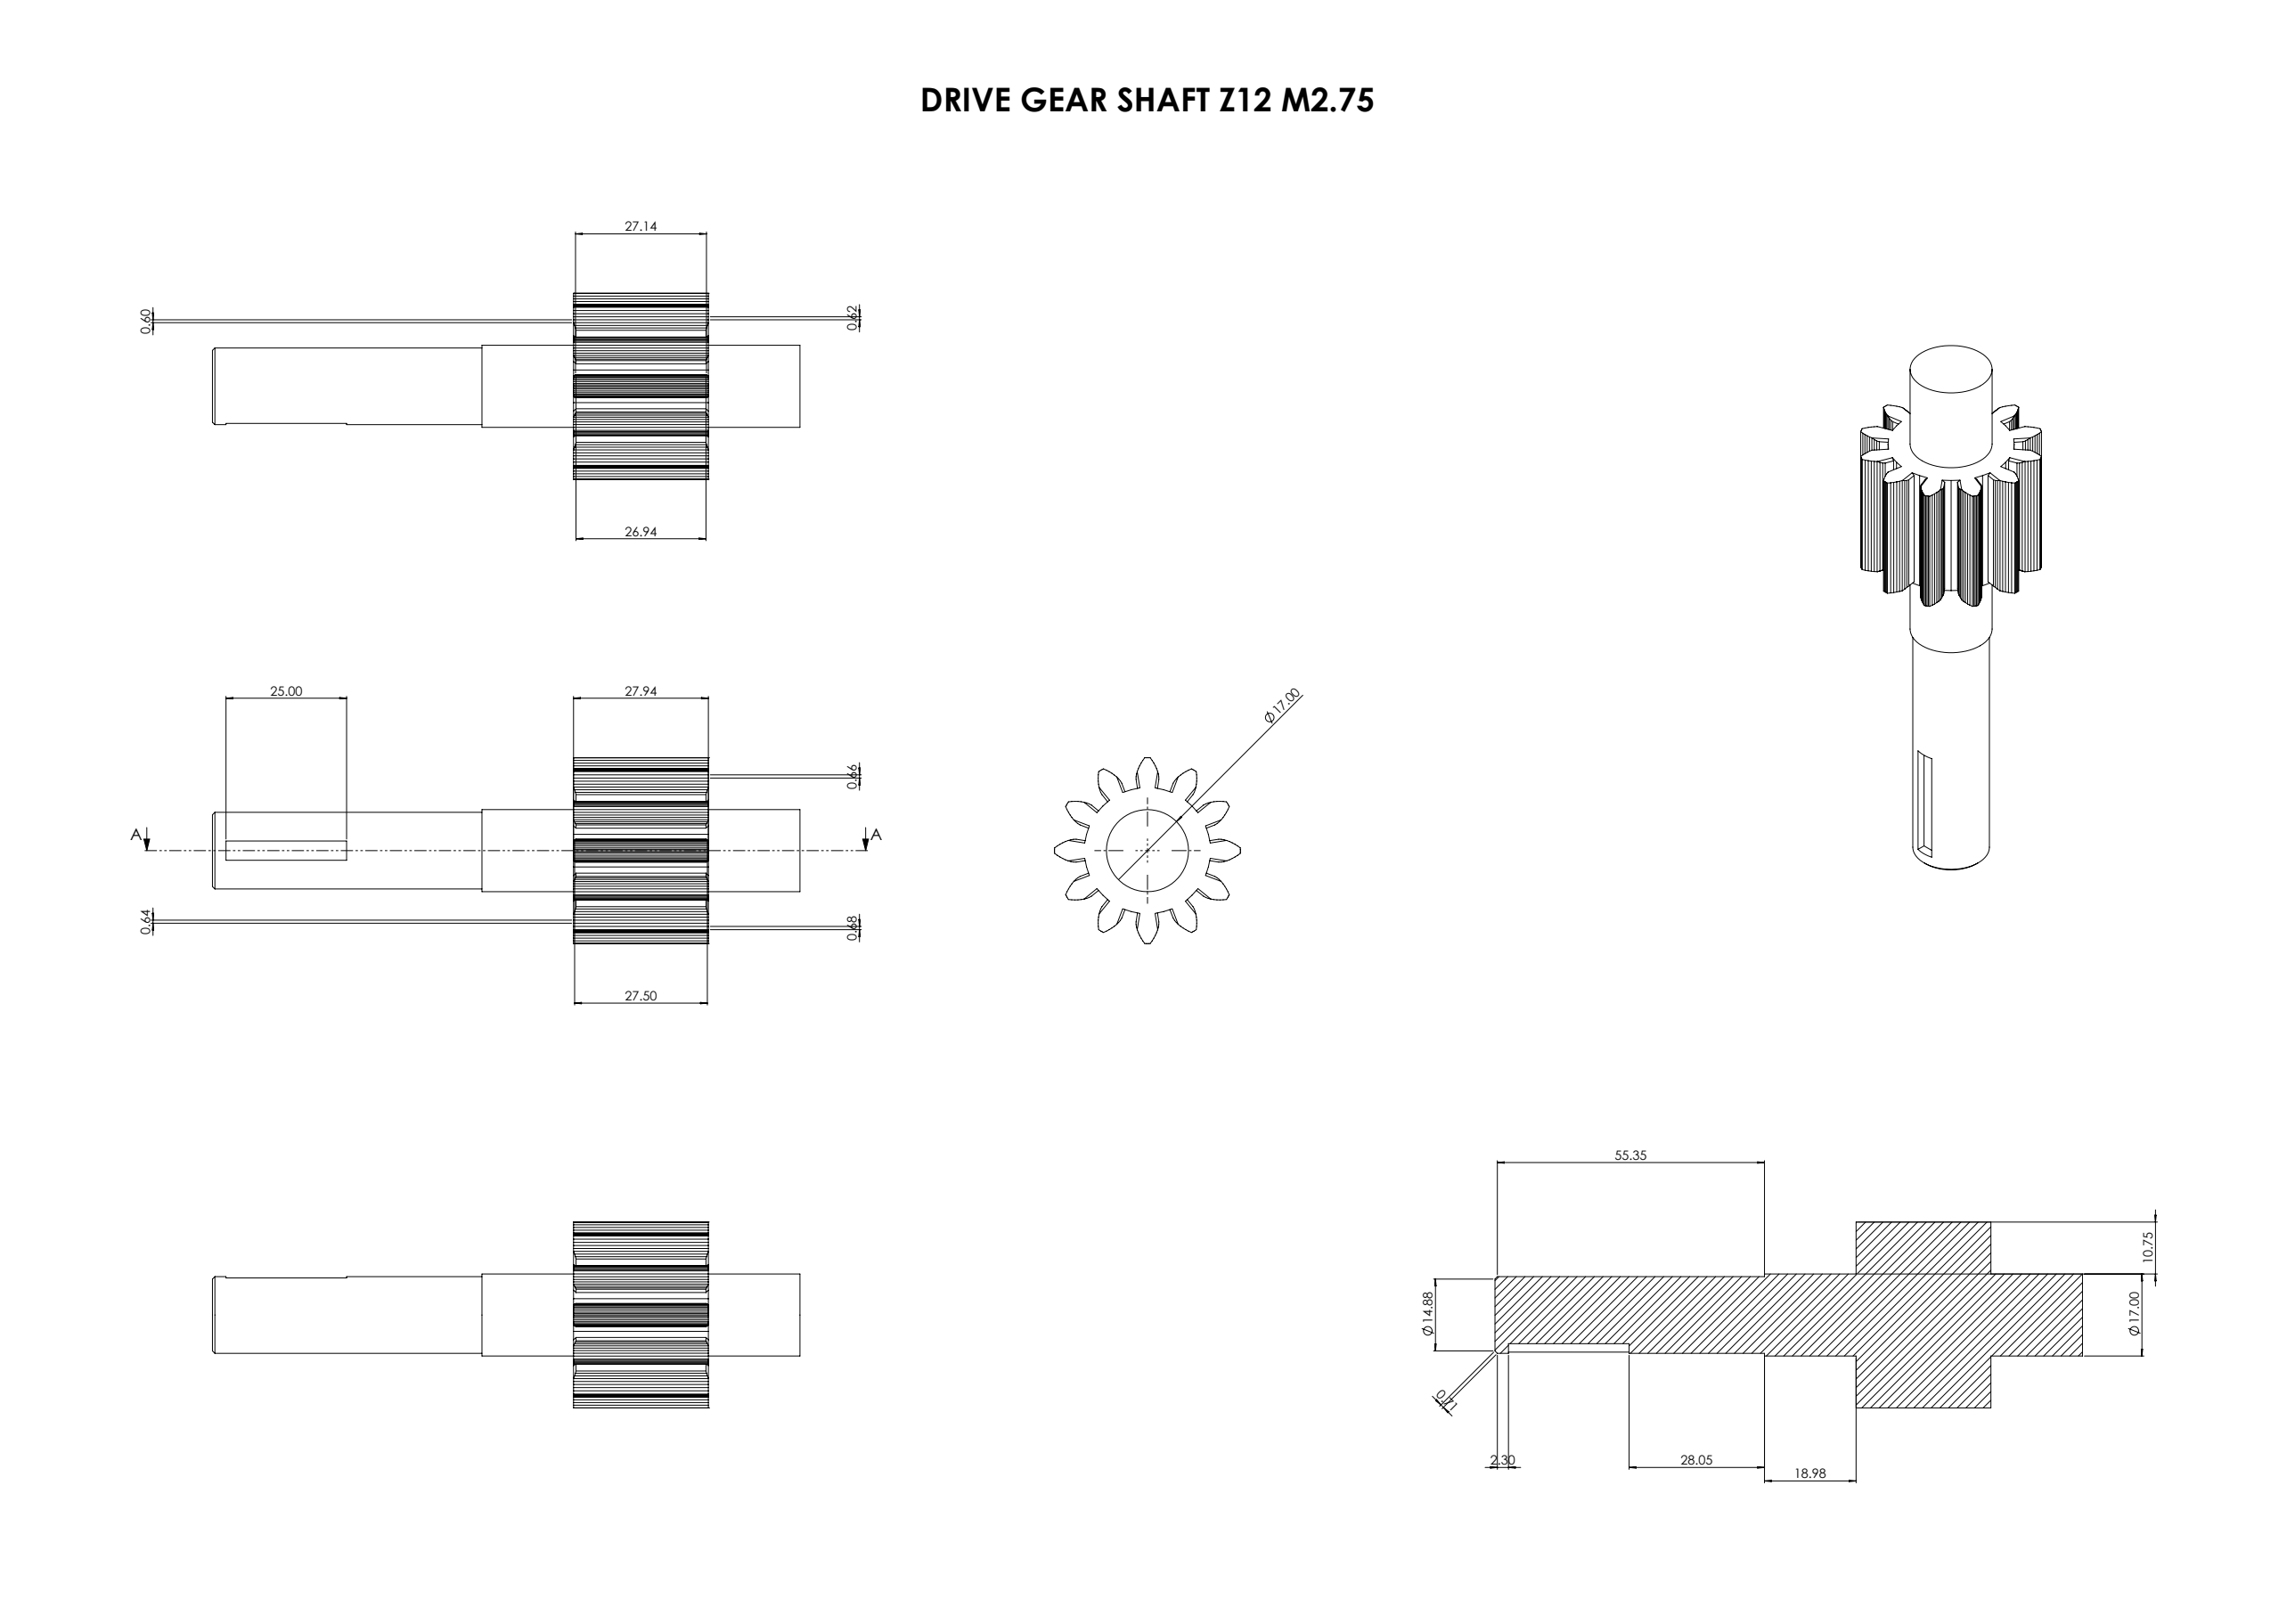
ISO-10303-21;
HEADER;
/* Generated by software containing ST-Developer
 * from STEP Tools, Inc. (www.steptools.com) 
 */

FILE_DESCRIPTION(
/* description */ (''),
/* implementation_level */ '2;1');

FILE_NAME(
/* name */ '04_Drive_Gear_Shaft_z12_m2.75.step',
/* time_stamp */ '2026-10-26T06:59:52-07:00',
/* author */ (''),
/* organization */ (''),
/* preprocessor_version */ 'ST-DEVELOPER v20.2',
/* originating_system */ 'Autodesk Translation Framework v15.15.0.0',
/* authorisation */ '');

FILE_SCHEMA (('AUTOMOTIVE_DESIGN { 1 0 10303 214 3 1 1 }'));
ENDSEC;

DATA;
#10=MECHANICAL_DESIGN_GEOMETRIC_PRESENTATION_REPRESENTATION('',(#167),#46395);
#139=SHAPE_REPRESENTATION_RELATIONSHIP('SRR','None',#46459,#153);
#153=ADVANCED_BREP_SHAPE_REPRESENTATION('',(#181),#46384);
#167=STYLED_ITEM('',(#46596),#181);
#181=MANIFOLD_SOLID_BREP('Body1',#24940);
#514=CYLINDRICAL_SURFACE('',#26051,8.5);
#515=CYLINDRICAL_SURFACE('',#26057,7.94);
#516=CYLINDRICAL_SURFACE('',#26060,8.5);
#645=FACE_BOUND('',#3444,.T.);
#646=FACE_BOUND('',#3518,.T.);
#647=FACE_BOUND('',#3791,.T.);
#648=FACE_BOUND('',#3793,.T.);
#814=PLANE('',#25704);
#815=PLANE('',#25705);
#816=PLANE('',#25707);
#817=PLANE('',#25708);
#818=PLANE('',#25709);
#819=PLANE('',#25710);
#820=PLANE('',#25711);
#821=PLANE('',#25712);
#822=PLANE('',#25713);
#823=PLANE('',#25714);
#824=PLANE('',#25715);
#825=PLANE('',#25716);
#826=PLANE('',#25717);
#827=PLANE('',#25718);
#828=PLANE('',#25719);
#829=PLANE('',#25720);
#830=PLANE('',#25721);
#831=PLANE('',#25722);
#832=PLANE('',#25723);
#833=PLANE('',#25724);
#834=PLANE('',#25725);
#835=PLANE('',#25726);
#836=PLANE('',#25727);
#837=PLANE('',#25728);
#838=PLANE('',#25729);
#839=PLANE('',#25730);
#840=PLANE('',#25731);
#841=PLANE('',#25732);
#842=PLANE('',#25733);
#843=PLANE('',#25734);
#844=PLANE('',#25735);
#845=PLANE('',#25736);
#846=PLANE('',#25737);
#847=PLANE('',#25738);
#848=PLANE('',#25739);
#849=PLANE('',#25740);
#850=PLANE('',#25741);
#851=PLANE('',#25742);
#852=PLANE('',#25743);
#853=PLANE('',#25744);
#854=PLANE('',#25745);
#855=PLANE('',#25746);
#856=PLANE('',#25747);
#857=PLANE('',#25748);
#858=PLANE('',#25749);
#859=PLANE('',#25750);
#860=PLANE('',#25751);
#861=PLANE('',#25752);
#862=PLANE('',#25753);
#863=PLANE('',#25754);
#864=PLANE('',#25755);
#865=PLANE('',#25756);
#866=PLANE('',#25757);
#867=PLANE('',#25758);
#868=PLANE('',#25759);
#869=PLANE('',#25760);
#870=PLANE('',#25761);
#871=PLANE('',#25762);
#872=PLANE('',#25763);
#873=PLANE('',#25764);
#874=PLANE('',#25765);
#875=PLANE('',#25766);
#876=PLANE('',#25767);
#877=PLANE('',#25768);
#878=PLANE('',#25769);
#879=PLANE('',#25770);
#880=PLANE('',#25771);
#881=PLANE('',#25772);
#882=PLANE('',#25773);
#883=PLANE('',#25774);
#884=PLANE('',#25775);
#885=PLANE('',#25776);
#886=PLANE('',#25777);
#887=PLANE('',#25778);
#888=PLANE('',#25779);
#889=PLANE('',#25781);
#890=PLANE('',#25782);
#891=PLANE('',#25783);
#892=PLANE('',#25784);
#893=PLANE('',#25785);
#894=PLANE('',#25786);
#895=PLANE('',#25787);
#896=PLANE('',#25788);
#897=PLANE('',#25789);
#898=PLANE('',#25790);
#899=PLANE('',#25791);
#900=PLANE('',#25792);
#901=PLANE('',#25793);
#902=PLANE('',#25794);
#903=PLANE('',#25795);
#904=PLANE('',#25796);
#905=PLANE('',#25797);
#906=PLANE('',#25798);
#907=PLANE('',#25799);
#908=PLANE('',#25800);
#909=PLANE('',#25801);
#910=PLANE('',#25802);
#911=PLANE('',#25803);
#912=PLANE('',#25804);
#913=PLANE('',#25806);
#914=PLANE('',#25807);
#915=PLANE('',#25808);
#916=PLANE('',#25810);
#917=PLANE('',#25811);
#918=PLANE('',#25812);
#919=PLANE('',#25813);
#920=PLANE('',#25814);
#921=PLANE('',#25815);
#922=PLANE('',#25816);
#923=PLANE('',#25817);
#924=PLANE('',#25818);
#925=PLANE('',#25819);
#926=PLANE('',#25820);
#927=PLANE('',#25821);
#928=PLANE('',#25822);
#929=PLANE('',#25823);
#930=PLANE('',#25824);
#931=PLANE('',#25825);
#932=PLANE('',#25826);
#933=PLANE('',#25827);
#934=PLANE('',#25828);
#935=PLANE('',#25829);
#936=PLANE('',#25830);
#937=PLANE('',#25831);
#938=PLANE('',#25832);
#939=PLANE('',#25833);
#940=PLANE('',#25834);
#941=PLANE('',#25835);
#942=PLANE('',#25836);
#943=PLANE('',#25837);
#944=PLANE('',#25838);
#945=PLANE('',#25839);
#946=PLANE('',#25840);
#947=PLANE('',#25841);
#948=PLANE('',#25842);
#949=PLANE('',#25843);
#950=PLANE('',#25844);
#951=PLANE('',#25845);
#952=PLANE('',#25846);
#953=PLANE('',#25847);
#954=PLANE('',#25848);
#955=PLANE('',#25849);
#956=PLANE('',#25850);
#957=PLANE('',#25851);
#958=PLANE('',#25852);
#959=PLANE('',#25853);
#960=PLANE('',#25854);
#961=PLANE('',#25855);
#962=PLANE('',#25856);
#963=PLANE('',#25857);
#964=PLANE('',#25858);
#965=PLANE('',#25859);
#966=PLANE('',#25860);
#967=PLANE('',#25861);
#968=PLANE('',#25862);
#969=PLANE('',#25863);
#970=PLANE('',#25864);
#971=PLANE('',#25865);
#972=PLANE('',#25866);
#973=PLANE('',#25867);
#974=PLANE('',#25868);
#975=PLANE('',#25869);
#976=PLANE('',#25870);
#977=PLANE('',#25871);
#978=PLANE('',#25872);
#979=PLANE('',#25873);
#980=PLANE('',#25874);
#981=PLANE('',#25875);
#982=PLANE('',#25876);
#983=PLANE('',#25877);
#984=PLANE('',#25878);
#985=PLANE('',#25879);
#986=PLANE('',#25880);
#987=PLANE('',#25881);
#988=PLANE('',#25882);
#989=PLANE('',#25883);
#990=PLANE('',#25884);
#991=PLANE('',#25885);
#992=PLANE('',#25886);
#993=PLANE('',#25887);
#994=PLANE('',#25888);
#995=PLANE('',#25889);
#996=PLANE('',#25890);
#997=PLANE('',#25891);
#998=PLANE('',#25892);
#999=PLANE('',#25893);
#1000=PLANE('',#25894);
#1001=PLANE('',#25895);
#1002=PLANE('',#25896);
#1003=PLANE('',#25897);
#1004=PLANE('',#25898);
#1005=PLANE('',#25899);
#1006=PLANE('',#25900);
#1007=PLANE('',#25901);
#1008=PLANE('',#25902);
#1009=PLANE('',#25903);
#1010=PLANE('',#25904);
#1011=PLANE('',#25905);
#1012=PLANE('',#25906);
#1013=PLANE('',#25907);
#1014=PLANE('',#25908);
#1015=PLANE('',#25909);
#1016=PLANE('',#25910);
#1017=PLANE('',#25911);
#1018=PLANE('',#25912);
#1019=PLANE('',#25913);
#1020=PLANE('',#25914);
#1021=PLANE('',#25915);
#1022=PLANE('',#25916);
#1023=PLANE('',#25917);
#1024=PLANE('',#25918);
#1025=PLANE('',#25919);
#1026=PLANE('',#25920);
#1027=PLANE('',#25921);
#1028=PLANE('',#25922);
#1029=PLANE('',#25923);
#1030=PLANE('',#25924);
#1031=PLANE('',#25925);
#1032=PLANE('',#25926);
#1033=PLANE('',#25927);
#1034=PLANE('',#25928);
#1035=PLANE('',#25929);
#1036=PLANE('',#25930);
#1037=PLANE('',#25931);
#1038=PLANE('',#25932);
#1039=PLANE('',#25933);
#1040=PLANE('',#25934);
#1041=PLANE('',#25935);
#1042=PLANE('',#25936);
#1043=PLANE('',#25937);
#1044=PLANE('',#25938);
#1045=PLANE('',#25939);
#1046=PLANE('',#25940);
#1047=PLANE('',#25941);
#1048=PLANE('',#25942);
#1049=PLANE('',#25943);
#1050=PLANE('',#25944);
#1051=PLANE('',#25945);
#1052=PLANE('',#25946);
#1053=PLANE('',#25947);
#1054=PLANE('',#25948);
#1055=PLANE('',#25949);
#1056=PLANE('',#25950);
#1057=PLANE('',#25951);
#1058=PLANE('',#25952);
#1059=PLANE('',#25953);
#1060=PLANE('',#25954);
#1061=PLANE('',#25955);
#1062=PLANE('',#25956);
#1063=PLANE('',#25957);
#1064=PLANE('',#25958);
#1065=PLANE('',#25959);
#1066=PLANE('',#25960);
#1067=PLANE('',#25961);
#1068=PLANE('',#25962);
#1069=PLANE('',#25963);
#1070=PLANE('',#25964);
#1071=PLANE('',#25965);
#1072=PLANE('',#25966);
#1073=PLANE('',#25967);
#1074=PLANE('',#25968);
#1075=PLANE('',#25969);
#1076=PLANE('',#25970);
#1077=PLANE('',#25971);
#1078=PLANE('',#25972);
#1079=PLANE('',#25973);
#1080=PLANE('',#25974);
#1081=PLANE('',#25975);
#1082=PLANE('',#25976);
#1083=PLANE('',#25977);
#1084=PLANE('',#25978);
#1085=PLANE('',#25979);
#1086=PLANE('',#25980);
#1087=PLANE('',#25981);
#1088=PLANE('',#25982);
#1089=PLANE('',#25983);
#1090=PLANE('',#25984);
#1091=PLANE('',#25985);
#1092=PLANE('',#25986);
#1093=PLANE('',#25987);
#1094=PLANE('',#25988);
#1095=PLANE('',#25989);
#1096=PLANE('',#25990);
#1097=PLANE('',#25991);
#1098=PLANE('',#25992);
#1099=PLANE('',#25993);
#1100=PLANE('',#25994);
#1101=PLANE('',#25995);
#1102=PLANE('',#25996);
#1103=PLANE('',#25997);
#1104=PLANE('',#25998);
#1105=PLANE('',#25999);
#1106=PLANE('',#26000);
#1107=PLANE('',#26001);
#1108=PLANE('',#26002);
#1109=PLANE('',#26003);
#1110=PLANE('',#26004);
#1111=PLANE('',#26005);
#1112=PLANE('',#26006);
#1113=PLANE('',#26007);
#1114=PLANE('',#26008);
#1115=PLANE('',#26009);
#1116=PLANE('',#26010);
#1117=PLANE('',#26011);
#1118=PLANE('',#26012);
#1119=PLANE('',#26013);
#1120=PLANE('',#26014);
#1121=PLANE('',#26015);
#1122=PLANE('',#26016);
#1123=PLANE('',#26017);
#1124=PLANE('',#26018);
#1125=PLANE('',#26019);
#1126=PLANE('',#26020);
#1127=PLANE('',#26021);
#1128=PLANE('',#26022);
#1129=PLANE('',#26023);
#1130=PLANE('',#26024);
#1131=PLANE('',#26025);
#1132=PLANE('',#26026);
#1133=PLANE('',#26027);
#1134=PLANE('',#26028);
#1135=PLANE('',#26029);
#1136=PLANE('',#26030);
#1137=PLANE('',#26031);
#1138=PLANE('',#26032);
#1139=PLANE('',#26033);
#1140=PLANE('',#26034);
#1141=PLANE('',#26035);
#1142=PLANE('',#26036);
#1143=PLANE('',#26037);
#1144=PLANE('',#26038);
#1145=PLANE('',#26039);
#1146=PLANE('',#26040);
#1147=PLANE('',#26041);
#1148=PLANE('',#26042);
#1149=PLANE('',#26043);
#1150=PLANE('',#26044);
#1151=PLANE('',#26045);
#1152=PLANE('',#26046);
#1153=PLANE('',#26047);
#1154=PLANE('',#26048);
#1155=PLANE('',#26049);
#1156=PLANE('',#26050);
#1157=PLANE('',#26053);
#1158=PLANE('',#26059);
#1159=PLANE('',#26062);
#2052=FACE_OUTER_BOUND('',#3442,.T.);
#2053=FACE_OUTER_BOUND('',#3443,.T.);
#2054=FACE_OUTER_BOUND('',#3445,.T.);
#2055=FACE_OUTER_BOUND('',#3446,.T.);
#2056=FACE_OUTER_BOUND('',#3447,.T.);
#2057=FACE_OUTER_BOUND('',#3448,.T.);
#2058=FACE_OUTER_BOUND('',#3449,.T.);
#2059=FACE_OUTER_BOUND('',#3450,.T.);
#2060=FACE_OUTER_BOUND('',#3451,.T.);
#2061=FACE_OUTER_BOUND('',#3452,.T.);
#2062=FACE_OUTER_BOUND('',#3453,.T.);
#2063=FACE_OUTER_BOUND('',#3454,.T.);
#2064=FACE_OUTER_BOUND('',#3455,.T.);
#2065=FACE_OUTER_BOUND('',#3456,.T.);
#2066=FACE_OUTER_BOUND('',#3457,.T.);
#2067=FACE_OUTER_BOUND('',#3458,.T.);
#2068=FACE_OUTER_BOUND('',#3459,.T.);
#2069=FACE_OUTER_BOUND('',#3460,.T.);
#2070=FACE_OUTER_BOUND('',#3461,.T.);
#2071=FACE_OUTER_BOUND('',#3462,.T.);
#2072=FACE_OUTER_BOUND('',#3463,.T.);
#2073=FACE_OUTER_BOUND('',#3464,.T.);
#2074=FACE_OUTER_BOUND('',#3465,.T.);
#2075=FACE_OUTER_BOUND('',#3466,.T.);
#2076=FACE_OUTER_BOUND('',#3467,.T.);
#2077=FACE_OUTER_BOUND('',#3468,.T.);
#2078=FACE_OUTER_BOUND('',#3469,.T.);
#2079=FACE_OUTER_BOUND('',#3470,.T.);
#2080=FACE_OUTER_BOUND('',#3471,.T.);
#2081=FACE_OUTER_BOUND('',#3472,.T.);
#2082=FACE_OUTER_BOUND('',#3473,.T.);
#2083=FACE_OUTER_BOUND('',#3474,.T.);
#2084=FACE_OUTER_BOUND('',#3475,.T.);
#2085=FACE_OUTER_BOUND('',#3476,.T.);
#2086=FACE_OUTER_BOUND('',#3477,.T.);
#2087=FACE_OUTER_BOUND('',#3478,.T.);
#2088=FACE_OUTER_BOUND('',#3479,.T.);
#2089=FACE_OUTER_BOUND('',#3480,.T.);
#2090=FACE_OUTER_BOUND('',#3481,.T.);
#2091=FACE_OUTER_BOUND('',#3482,.T.);
#2092=FACE_OUTER_BOUND('',#3483,.T.);
#2093=FACE_OUTER_BOUND('',#3484,.T.);
#2094=FACE_OUTER_BOUND('',#3485,.T.);
#2095=FACE_OUTER_BOUND('',#3486,.T.);
#2096=FACE_OUTER_BOUND('',#3487,.T.);
#2097=FACE_OUTER_BOUND('',#3488,.T.);
#2098=FACE_OUTER_BOUND('',#3489,.T.);
#2099=FACE_OUTER_BOUND('',#3490,.T.);
#2100=FACE_OUTER_BOUND('',#3491,.T.);
#2101=FACE_OUTER_BOUND('',#3492,.T.);
#2102=FACE_OUTER_BOUND('',#3493,.T.);
#2103=FACE_OUTER_BOUND('',#3494,.T.);
#2104=FACE_OUTER_BOUND('',#3495,.T.);
#2105=FACE_OUTER_BOUND('',#3496,.T.);
#2106=FACE_OUTER_BOUND('',#3497,.T.);
#2107=FACE_OUTER_BOUND('',#3498,.T.);
#2108=FACE_OUTER_BOUND('',#3499,.T.);
#2109=FACE_OUTER_BOUND('',#3500,.T.);
#2110=FACE_OUTER_BOUND('',#3501,.T.);
#2111=FACE_OUTER_BOUND('',#3502,.T.);
#2112=FACE_OUTER_BOUND('',#3503,.T.);
#2113=FACE_OUTER_BOUND('',#3504,.T.);
#2114=FACE_OUTER_BOUND('',#3505,.T.);
#2115=FACE_OUTER_BOUND('',#3506,.T.);
#2116=FACE_OUTER_BOUND('',#3507,.T.);
#2117=FACE_OUTER_BOUND('',#3508,.T.);
#2118=FACE_OUTER_BOUND('',#3509,.T.);
#2119=FACE_OUTER_BOUND('',#3510,.T.);
#2120=FACE_OUTER_BOUND('',#3511,.T.);
#2121=FACE_OUTER_BOUND('',#3512,.T.);
#2122=FACE_OUTER_BOUND('',#3513,.T.);
#2123=FACE_OUTER_BOUND('',#3514,.T.);
#2124=FACE_OUTER_BOUND('',#3515,.T.);
#2125=FACE_OUTER_BOUND('',#3516,.T.);
#2126=FACE_OUTER_BOUND('',#3517,.T.);
#2127=FACE_OUTER_BOUND('',#3519,.T.);
#2128=FACE_OUTER_BOUND('',#3520,.T.);
#2129=FACE_OUTER_BOUND('',#3521,.T.);
#2130=FACE_OUTER_BOUND('',#3522,.T.);
#2131=FACE_OUTER_BOUND('',#3523,.T.);
#2132=FACE_OUTER_BOUND('',#3524,.T.);
#2133=FACE_OUTER_BOUND('',#3525,.T.);
#2134=FACE_OUTER_BOUND('',#3526,.T.);
#2135=FACE_OUTER_BOUND('',#3527,.T.);
#2136=FACE_OUTER_BOUND('',#3528,.T.);
#2137=FACE_OUTER_BOUND('',#3529,.T.);
#2138=FACE_OUTER_BOUND('',#3530,.T.);
#2139=FACE_OUTER_BOUND('',#3531,.T.);
#2140=FACE_OUTER_BOUND('',#3532,.T.);
#2141=FACE_OUTER_BOUND('',#3533,.T.);
#2142=FACE_OUTER_BOUND('',#3534,.T.);
#2143=FACE_OUTER_BOUND('',#3535,.T.);
#2144=FACE_OUTER_BOUND('',#3536,.T.);
#2145=FACE_OUTER_BOUND('',#3537,.T.);
#2146=FACE_OUTER_BOUND('',#3538,.T.);
#2147=FACE_OUTER_BOUND('',#3539,.T.);
#2148=FACE_OUTER_BOUND('',#3540,.T.);
#2149=FACE_OUTER_BOUND('',#3541,.T.);
#2150=FACE_OUTER_BOUND('',#3542,.T.);
#2151=FACE_OUTER_BOUND('',#3543,.T.);
#2152=FACE_OUTER_BOUND('',#3544,.T.);
#2153=FACE_OUTER_BOUND('',#3545,.T.);
#2154=FACE_OUTER_BOUND('',#3546,.T.);
#2155=FACE_OUTER_BOUND('',#3547,.T.);
#2156=FACE_OUTER_BOUND('',#3548,.T.);
#2157=FACE_OUTER_BOUND('',#3549,.T.);
#2158=FACE_OUTER_BOUND('',#3550,.T.);
#2159=FACE_OUTER_BOUND('',#3551,.T.);
#2160=FACE_OUTER_BOUND('',#3552,.T.);
#2161=FACE_OUTER_BOUND('',#3553,.T.);
#2162=FACE_OUTER_BOUND('',#3554,.T.);
#2163=FACE_OUTER_BOUND('',#3555,.T.);
#2164=FACE_OUTER_BOUND('',#3556,.T.);
#2165=FACE_OUTER_BOUND('',#3557,.T.);
#2166=FACE_OUTER_BOUND('',#3558,.T.);
#2167=FACE_OUTER_BOUND('',#3559,.T.);
#2168=FACE_OUTER_BOUND('',#3560,.T.);
#2169=FACE_OUTER_BOUND('',#3561,.T.);
#2170=FACE_OUTER_BOUND('',#3562,.T.);
#2171=FACE_OUTER_BOUND('',#3563,.T.);
#2172=FACE_OUTER_BOUND('',#3564,.T.);
#2173=FACE_OUTER_BOUND('',#3565,.T.);
#2174=FACE_OUTER_BOUND('',#3566,.T.);
#2175=FACE_OUTER_BOUND('',#3567,.T.);
#2176=FACE_OUTER_BOUND('',#3568,.T.);
#2177=FACE_OUTER_BOUND('',#3569,.T.);
#2178=FACE_OUTER_BOUND('',#3570,.T.);
#2179=FACE_OUTER_BOUND('',#3571,.T.);
#2180=FACE_OUTER_BOUND('',#3572,.T.);
#2181=FACE_OUTER_BOUND('',#3573,.T.);
#2182=FACE_OUTER_BOUND('',#3574,.T.);
#2183=FACE_OUTER_BOUND('',#3575,.T.);
#2184=FACE_OUTER_BOUND('',#3576,.T.);
#2185=FACE_OUTER_BOUND('',#3577,.T.);
#2186=FACE_OUTER_BOUND('',#3578,.T.);
#2187=FACE_OUTER_BOUND('',#3579,.T.);
#2188=FACE_OUTER_BOUND('',#3580,.T.);
#2189=FACE_OUTER_BOUND('',#3581,.T.);
#2190=FACE_OUTER_BOUND('',#3582,.T.);
#2191=FACE_OUTER_BOUND('',#3583,.T.);
#2192=FACE_OUTER_BOUND('',#3584,.T.);
#2193=FACE_OUTER_BOUND('',#3585,.T.);
#2194=FACE_OUTER_BOUND('',#3586,.T.);
#2195=FACE_OUTER_BOUND('',#3587,.T.);
#2196=FACE_OUTER_BOUND('',#3588,.T.);
#2197=FACE_OUTER_BOUND('',#3589,.T.);
#2198=FACE_OUTER_BOUND('',#3590,.T.);
#2199=FACE_OUTER_BOUND('',#3591,.T.);
#2200=FACE_OUTER_BOUND('',#3592,.T.);
#2201=FACE_OUTER_BOUND('',#3593,.T.);
#2202=FACE_OUTER_BOUND('',#3594,.T.);
#2203=FACE_OUTER_BOUND('',#3595,.T.);
#2204=FACE_OUTER_BOUND('',#3596,.T.);
#2205=FACE_OUTER_BOUND('',#3597,.T.);
#2206=FACE_OUTER_BOUND('',#3598,.T.);
#2207=FACE_OUTER_BOUND('',#3599,.T.);
#2208=FACE_OUTER_BOUND('',#3600,.T.);
#2209=FACE_OUTER_BOUND('',#3601,.T.);
#2210=FACE_OUTER_BOUND('',#3602,.T.);
#2211=FACE_OUTER_BOUND('',#3603,.T.);
#2212=FACE_OUTER_BOUND('',#3604,.T.);
#2213=FACE_OUTER_BOUND('',#3605,.T.);
#2214=FACE_OUTER_BOUND('',#3606,.T.);
#2215=FACE_OUTER_BOUND('',#3607,.T.);
#2216=FACE_OUTER_BOUND('',#3608,.T.);
#2217=FACE_OUTER_BOUND('',#3609,.T.);
#2218=FACE_OUTER_BOUND('',#3610,.T.);
#2219=FACE_OUTER_BOUND('',#3611,.T.);
#2220=FACE_OUTER_BOUND('',#3612,.T.);
#2221=FACE_OUTER_BOUND('',#3613,.T.);
#2222=FACE_OUTER_BOUND('',#3614,.T.);
#2223=FACE_OUTER_BOUND('',#3615,.T.);
#2224=FACE_OUTER_BOUND('',#3616,.T.);
#2225=FACE_OUTER_BOUND('',#3617,.T.);
#2226=FACE_OUTER_BOUND('',#3618,.T.);
#2227=FACE_OUTER_BOUND('',#3619,.T.);
#2228=FACE_OUTER_BOUND('',#3620,.T.);
#2229=FACE_OUTER_BOUND('',#3621,.T.);
#2230=FACE_OUTER_BOUND('',#3622,.T.);
#2231=FACE_OUTER_BOUND('',#3623,.T.);
#2232=FACE_OUTER_BOUND('',#3624,.T.);
#2233=FACE_OUTER_BOUND('',#3625,.T.);
#2234=FACE_OUTER_BOUND('',#3626,.T.);
#2235=FACE_OUTER_BOUND('',#3627,.T.);
#2236=FACE_OUTER_BOUND('',#3628,.T.);
#2237=FACE_OUTER_BOUND('',#3629,.T.);
#2238=FACE_OUTER_BOUND('',#3630,.T.);
#2239=FACE_OUTER_BOUND('',#3631,.T.);
#2240=FACE_OUTER_BOUND('',#3632,.T.);
#2241=FACE_OUTER_BOUND('',#3633,.T.);
#2242=FACE_OUTER_BOUND('',#3634,.T.);
#2243=FACE_OUTER_BOUND('',#3635,.T.);
#2244=FACE_OUTER_BOUND('',#3636,.T.);
#2245=FACE_OUTER_BOUND('',#3637,.T.);
#2246=FACE_OUTER_BOUND('',#3638,.T.);
#2247=FACE_OUTER_BOUND('',#3639,.T.);
#2248=FACE_OUTER_BOUND('',#3640,.T.);
#2249=FACE_OUTER_BOUND('',#3641,.T.);
#2250=FACE_OUTER_BOUND('',#3642,.T.);
#2251=FACE_OUTER_BOUND('',#3643,.T.);
#2252=FACE_OUTER_BOUND('',#3644,.T.);
#2253=FACE_OUTER_BOUND('',#3645,.T.);
#2254=FACE_OUTER_BOUND('',#3646,.T.);
#2255=FACE_OUTER_BOUND('',#3647,.T.);
#2256=FACE_OUTER_BOUND('',#3648,.T.);
#2257=FACE_OUTER_BOUND('',#3649,.T.);
#2258=FACE_OUTER_BOUND('',#3650,.T.);
#2259=FACE_OUTER_BOUND('',#3651,.T.);
#2260=FACE_OUTER_BOUND('',#3652,.T.);
#2261=FACE_OUTER_BOUND('',#3653,.T.);
#2262=FACE_OUTER_BOUND('',#3654,.T.);
#2263=FACE_OUTER_BOUND('',#3655,.T.);
#2264=FACE_OUTER_BOUND('',#3656,.T.);
#2265=FACE_OUTER_BOUND('',#3657,.T.);
#2266=FACE_OUTER_BOUND('',#3658,.T.);
#2267=FACE_OUTER_BOUND('',#3659,.T.);
#2268=FACE_OUTER_BOUND('',#3660,.T.);
#2269=FACE_OUTER_BOUND('',#3661,.T.);
#2270=FACE_OUTER_BOUND('',#3662,.T.);
#2271=FACE_OUTER_BOUND('',#3663,.T.);
#2272=FACE_OUTER_BOUND('',#3664,.T.);
#2273=FACE_OUTER_BOUND('',#3665,.T.);
#2274=FACE_OUTER_BOUND('',#3666,.T.);
#2275=FACE_OUTER_BOUND('',#3667,.T.);
#2276=FACE_OUTER_BOUND('',#3668,.T.);
#2277=FACE_OUTER_BOUND('',#3669,.T.);
#2278=FACE_OUTER_BOUND('',#3670,.T.);
#2279=FACE_OUTER_BOUND('',#3671,.T.);
#2280=FACE_OUTER_BOUND('',#3672,.T.);
#2281=FACE_OUTER_BOUND('',#3673,.T.);
#2282=FACE_OUTER_BOUND('',#3674,.T.);
#2283=FACE_OUTER_BOUND('',#3675,.T.);
#2284=FACE_OUTER_BOUND('',#3676,.T.);
#2285=FACE_OUTER_BOUND('',#3677,.T.);
#2286=FACE_OUTER_BOUND('',#3678,.T.);
#2287=FACE_OUTER_BOUND('',#3679,.T.);
#2288=FACE_OUTER_BOUND('',#3680,.T.);
#2289=FACE_OUTER_BOUND('',#3681,.T.);
#2290=FACE_OUTER_BOUND('',#3682,.T.);
#2291=FACE_OUTER_BOUND('',#3683,.T.);
#2292=FACE_OUTER_BOUND('',#3684,.T.);
#2293=FACE_OUTER_BOUND('',#3685,.T.);
#2294=FACE_OUTER_BOUND('',#3686,.T.);
#2295=FACE_OUTER_BOUND('',#3687,.T.);
#2296=FACE_OUTER_BOUND('',#3688,.T.);
#2297=FACE_OUTER_BOUND('',#3689,.T.);
#2298=FACE_OUTER_BOUND('',#3690,.T.);
#2299=FACE_OUTER_BOUND('',#3691,.T.);
#2300=FACE_OUTER_BOUND('',#3692,.T.);
#2301=FACE_OUTER_BOUND('',#3693,.T.);
#2302=FACE_OUTER_BOUND('',#3694,.T.);
#2303=FACE_OUTER_BOUND('',#3695,.T.);
#2304=FACE_OUTER_BOUND('',#3696,.T.);
#2305=FACE_OUTER_BOUND('',#3697,.T.);
#2306=FACE_OUTER_BOUND('',#3698,.T.);
#2307=FACE_OUTER_BOUND('',#3699,.T.);
#2308=FACE_OUTER_BOUND('',#3700,.T.);
#2309=FACE_OUTER_BOUND('',#3701,.T.);
#2310=FACE_OUTER_BOUND('',#3702,.T.);
#2311=FACE_OUTER_BOUND('',#3703,.T.);
#2312=FACE_OUTER_BOUND('',#3704,.T.);
#2313=FACE_OUTER_BOUND('',#3705,.T.);
#2314=FACE_OUTER_BOUND('',#3706,.T.);
#2315=FACE_OUTER_BOUND('',#3707,.T.);
#2316=FACE_OUTER_BOUND('',#3708,.T.);
#2317=FACE_OUTER_BOUND('',#3709,.T.);
#2318=FACE_OUTER_BOUND('',#3710,.T.);
#2319=FACE_OUTER_BOUND('',#3711,.T.);
#2320=FACE_OUTER_BOUND('',#3712,.T.);
#2321=FACE_OUTER_BOUND('',#3713,.T.);
#2322=FACE_OUTER_BOUND('',#3714,.T.);
#2323=FACE_OUTER_BOUND('',#3715,.T.);
#2324=FACE_OUTER_BOUND('',#3716,.T.);
#2325=FACE_OUTER_BOUND('',#3717,.T.);
#2326=FACE_OUTER_BOUND('',#3718,.T.);
#2327=FACE_OUTER_BOUND('',#3719,.T.);
#2328=FACE_OUTER_BOUND('',#3720,.T.);
#2329=FACE_OUTER_BOUND('',#3721,.T.);
#2330=FACE_OUTER_BOUND('',#3722,.T.);
#2331=FACE_OUTER_BOUND('',#3723,.T.);
#2332=FACE_OUTER_BOUND('',#3724,.T.);
#2333=FACE_OUTER_BOUND('',#3725,.T.);
#2334=FACE_OUTER_BOUND('',#3726,.T.);
#2335=FACE_OUTER_BOUND('',#3727,.T.);
#2336=FACE_OUTER_BOUND('',#3728,.T.);
#2337=FACE_OUTER_BOUND('',#3729,.T.);
#2338=FACE_OUTER_BOUND('',#3730,.T.);
#2339=FACE_OUTER_BOUND('',#3731,.T.);
#2340=FACE_OUTER_BOUND('',#3732,.T.);
#2341=FACE_OUTER_BOUND('',#3733,.T.);
#2342=FACE_OUTER_BOUND('',#3734,.T.);
#2343=FACE_OUTER_BOUND('',#3735,.T.);
#2344=FACE_OUTER_BOUND('',#3736,.T.);
#2345=FACE_OUTER_BOUND('',#3737,.T.);
#2346=FACE_OUTER_BOUND('',#3738,.T.);
#2347=FACE_OUTER_BOUND('',#3739,.T.);
#2348=FACE_OUTER_BOUND('',#3740,.T.);
#2349=FACE_OUTER_BOUND('',#3741,.T.);
#2350=FACE_OUTER_BOUND('',#3742,.T.);
#2351=FACE_OUTER_BOUND('',#3743,.T.);
#2352=FACE_OUTER_BOUND('',#3744,.T.);
#2353=FACE_OUTER_BOUND('',#3745,.T.);
#2354=FACE_OUTER_BOUND('',#3746,.T.);
#2355=FACE_OUTER_BOUND('',#3747,.T.);
#2356=FACE_OUTER_BOUND('',#3748,.T.);
#2357=FACE_OUTER_BOUND('',#3749,.T.);
#2358=FACE_OUTER_BOUND('',#3750,.T.);
#2359=FACE_OUTER_BOUND('',#3751,.T.);
#2360=FACE_OUTER_BOUND('',#3752,.T.);
#2361=FACE_OUTER_BOUND('',#3753,.T.);
#2362=FACE_OUTER_BOUND('',#3754,.T.);
#2363=FACE_OUTER_BOUND('',#3755,.T.);
#2364=FACE_OUTER_BOUND('',#3756,.T.);
#2365=FACE_OUTER_BOUND('',#3757,.T.);
#2366=FACE_OUTER_BOUND('',#3758,.T.);
#2367=FACE_OUTER_BOUND('',#3759,.T.);
#2368=FACE_OUTER_BOUND('',#3760,.T.);
#2369=FACE_OUTER_BOUND('',#3761,.T.);
#2370=FACE_OUTER_BOUND('',#3762,.T.);
#2371=FACE_OUTER_BOUND('',#3763,.T.);
#2372=FACE_OUTER_BOUND('',#3764,.T.);
#2373=FACE_OUTER_BOUND('',#3765,.T.);
#2374=FACE_OUTER_BOUND('',#3766,.T.);
#2375=FACE_OUTER_BOUND('',#3767,.T.);
#2376=FACE_OUTER_BOUND('',#3768,.T.);
#2377=FACE_OUTER_BOUND('',#3769,.T.);
#2378=FACE_OUTER_BOUND('',#3770,.T.);
#2379=FACE_OUTER_BOUND('',#3771,.T.);
#2380=FACE_OUTER_BOUND('',#3772,.T.);
#2381=FACE_OUTER_BOUND('',#3773,.T.);
#2382=FACE_OUTER_BOUND('',#3774,.T.);
#2383=FACE_OUTER_BOUND('',#3775,.T.);
#2384=FACE_OUTER_BOUND('',#3776,.T.);
#2385=FACE_OUTER_BOUND('',#3777,.T.);
#2386=FACE_OUTER_BOUND('',#3778,.T.);
#2387=FACE_OUTER_BOUND('',#3779,.T.);
#2388=FACE_OUTER_BOUND('',#3780,.T.);
#2389=FACE_OUTER_BOUND('',#3781,.T.);
#2390=FACE_OUTER_BOUND('',#3782,.T.);
#2391=FACE_OUTER_BOUND('',#3783,.T.);
#2392=FACE_OUTER_BOUND('',#3784,.T.);
#2393=FACE_OUTER_BOUND('',#3785,.T.);
#2394=FACE_OUTER_BOUND('',#3786,.T.);
#2395=FACE_OUTER_BOUND('',#3787,.T.);
#2396=FACE_OUTER_BOUND('',#3788,.T.);
#2397=FACE_OUTER_BOUND('',#3789,.T.);
#2398=FACE_OUTER_BOUND('',#3790,.T.);
#2399=FACE_OUTER_BOUND('',#3792,.T.);
#2400=FACE_OUTER_BOUND('',#3794,.T.);
#2401=FACE_OUTER_BOUND('',#3795,.T.);
#3442=EDGE_LOOP('',(#17926,#17927,#17928,#17929,#17930,#17931));
#3443=EDGE_LOOP('',(#17932,#17933,#17934,#17935,#17936,#17937,#17938,#17939,
#17940,#17941,#17942,#17943,#17944,#17945,#17946,#17947,#17948,#17949,#17950,
#17951,#17952,#17953,#17954,#17955,#17956,#17957,#17958,#17959,#17960,#17961,
#17962,#17963,#17964,#17965,#17966,#17967,#17968,#17969,#17970,#17971,#17972,
#17973,#17974,#17975,#17976,#17977,#17978,#17979,#17980,#17981,#17982,#17983,
#17984,#17985,#17986,#17987,#17988,#17989,#17990,#17991,#17992,#17993,#17994,
#17995,#17996,#17997,#17998,#17999,#18000,#18001,#18002,#18003,#18004,#18005,
#18006,#18007,#18008,#18009,#18010,#18011,#18012,#18013,#18014,#18015,#18016,
#18017,#18018,#18019,#18020,#18021,#18022,#18023,#18024,#18025,#18026,#18027,
#18028,#18029,#18030,#18031,#18032,#18033,#18034,#18035,#18036,#18037,#18038,
#18039,#18040,#18041,#18042,#18043,#18044,#18045,#18046,#18047,#18048,#18049,
#18050,#18051,#18052,#18053,#18054,#18055,#18056,#18057,#18058,#18059,#18060,
#18061,#18062,#18063,#18064,#18065,#18066,#18067,#18068,#18069,#18070,#18071,
#18072,#18073,#18074,#18075,#18076,#18077,#18078,#18079,#18080,#18081,#18082,
#18083,#18084,#18085,#18086,#18087,#18088,#18089,#18090,#18091,#18092,#18093,
#18094,#18095,#18096,#18097,#18098,#18099,#18100,#18101,#18102,#18103,#18104,
#18105,#18106,#18107,#18108,#18109,#18110,#18111,#18112,#18113,#18114,#18115,
#18116,#18117,#18118,#18119,#18120,#18121,#18122,#18123,#18124,#18125,#18126,
#18127,#18128,#18129,#18130,#18131,#18132,#18133,#18134,#18135,#18136,#18137,
#18138,#18139,#18140,#18141,#18142,#18143,#18144,#18145,#18146,#18147,#18148,
#18149,#18150,#18151,#18152,#18153,#18154,#18155,#18156,#18157,#18158,#18159,
#18160,#18161,#18162,#18163,#18164,#18165,#18166,#18167,#18168,#18169,#18170,
#18171));
#3444=EDGE_LOOP('',(#18172));
#3445=EDGE_LOOP('',(#18173,#18174,#18175,#18176,#18177,#18178));
#3446=EDGE_LOOP('',(#18179,#18180,#18181,#18182));
#3447=EDGE_LOOP('',(#18183,#18184,#18185,#18186,#18187,#18188));
#3448=EDGE_LOOP('',(#18189,#18190,#18191,#18192,#18193,#18194));
#3449=EDGE_LOOP('',(#18195,#18196,#18197,#18198));
#3450=EDGE_LOOP('',(#18199,#18200,#18201,#18202,#18203,#18204));
#3451=EDGE_LOOP('',(#18205,#18206,#18207,#18208,#18209,#18210));
#3452=EDGE_LOOP('',(#18211,#18212,#18213,#18214));
#3453=EDGE_LOOP('',(#18215,#18216,#18217,#18218,#18219,#18220));
#3454=EDGE_LOOP('',(#18221,#18222,#18223,#18224,#18225,#18226));
#3455=EDGE_LOOP('',(#18227,#18228,#18229,#18230));
#3456=EDGE_LOOP('',(#18231,#18232,#18233,#18234,#18235,#18236));
#3457=EDGE_LOOP('',(#18237,#18238,#18239,#18240,#18241,#18242));
#3458=EDGE_LOOP('',(#18243,#18244,#18245,#18246));
#3459=EDGE_LOOP('',(#18247,#18248,#18249,#18250,#18251,#18252));
#3460=EDGE_LOOP('',(#18253,#18254,#18255,#18256,#18257,#18258));
#3461=EDGE_LOOP('',(#18259,#18260,#18261,#18262));
#3462=EDGE_LOOP('',(#18263,#18264,#18265,#18266,#18267,#18268));
#3463=EDGE_LOOP('',(#18269,#18270,#18271,#18272,#18273,#18274));
#3464=EDGE_LOOP('',(#18275,#18276,#18277,#18278));
#3465=EDGE_LOOP('',(#18279,#18280,#18281,#18282,#18283,#18284));
#3466=EDGE_LOOP('',(#18285,#18286,#18287,#18288,#18289,#18290));
#3467=EDGE_LOOP('',(#18291,#18292,#18293,#18294));
#3468=EDGE_LOOP('',(#18295,#18296,#18297,#18298,#18299,#18300));
#3469=EDGE_LOOP('',(#18301,#18302,#18303,#18304,#18305,#18306));
#3470=EDGE_LOOP('',(#18307,#18308,#18309,#18310));
#3471=EDGE_LOOP('',(#18311,#18312,#18313,#18314,#18315,#18316));
#3472=EDGE_LOOP('',(#18317,#18318,#18319,#18320,#18321,#18322));
#3473=EDGE_LOOP('',(#18323,#18324,#18325,#18326));
#3474=EDGE_LOOP('',(#18327,#18328,#18329,#18330,#18331,#18332));
#3475=EDGE_LOOP('',(#18333,#18334,#18335,#18336,#18337,#18338));
#3476=EDGE_LOOP('',(#18339,#18340,#18341,#18342));
#3477=EDGE_LOOP('',(#18343,#18344,#18345,#18346,#18347,#18348));
#3478=EDGE_LOOP('',(#18349,#18350,#18351,#18352,#18353,#18354));
#3479=EDGE_LOOP('',(#18355,#18356,#18357,#18358));
#3480=EDGE_LOOP('',(#18359,#18360,#18361,#18362,#18363,#18364));
#3481=EDGE_LOOP('',(#18365,#18366,#18367,#18368));
#3482=EDGE_LOOP('',(#18369,#18370,#18371,#18372));
#3483=EDGE_LOOP('',(#18373,#18374,#18375,#18376,#18377,#18378));
#3484=EDGE_LOOP('',(#18379,#18380,#18381,#18382));
#3485=EDGE_LOOP('',(#18383,#18384,#18385,#18386));
#3486=EDGE_LOOP('',(#18387,#18388,#18389,#18390,#18391,#18392));
#3487=EDGE_LOOP('',(#18393,#18394,#18395,#18396));
#3488=EDGE_LOOP('',(#18397,#18398,#18399,#18400));
#3489=EDGE_LOOP('',(#18401,#18402,#18403,#18404,#18405,#18406));
#3490=EDGE_LOOP('',(#18407,#18408,#18409,#18410));
#3491=EDGE_LOOP('',(#18411,#18412,#18413,#18414));
#3492=EDGE_LOOP('',(#18415,#18416,#18417,#18418,#18419,#18420));
#3493=EDGE_LOOP('',(#18421,#18422,#18423,#18424));
#3494=EDGE_LOOP('',(#18425,#18426,#18427,#18428));
#3495=EDGE_LOOP('',(#18429,#18430,#18431,#18432,#18433,#18434));
#3496=EDGE_LOOP('',(#18435,#18436,#18437,#18438));
#3497=EDGE_LOOP('',(#18439,#18440,#18441,#18442));
#3498=EDGE_LOOP('',(#18443,#18444,#18445,#18446,#18447,#18448));
#3499=EDGE_LOOP('',(#18449,#18450,#18451,#18452));
#3500=EDGE_LOOP('',(#18453,#18454,#18455,#18456));
#3501=EDGE_LOOP('',(#18457,#18458,#18459,#18460,#18461,#18462));
#3502=EDGE_LOOP('',(#18463,#18464,#18465,#18466));
#3503=EDGE_LOOP('',(#18467,#18468,#18469,#18470));
#3504=EDGE_LOOP('',(#18471,#18472,#18473,#18474,#18475,#18476));
#3505=EDGE_LOOP('',(#18477,#18478,#18479,#18480));
#3506=EDGE_LOOP('',(#18481,#18482,#18483,#18484));
#3507=EDGE_LOOP('',(#18485,#18486,#18487,#18488,#18489,#18490));
#3508=EDGE_LOOP('',(#18491,#18492,#18493,#18494));
#3509=EDGE_LOOP('',(#18495,#18496,#18497,#18498));
#3510=EDGE_LOOP('',(#18499,#18500,#18501,#18502,#18503,#18504));
#3511=EDGE_LOOP('',(#18505,#18506,#18507,#18508));
#3512=EDGE_LOOP('',(#18509,#18510,#18511,#18512));
#3513=EDGE_LOOP('',(#18513,#18514,#18515,#18516,#18517,#18518));
#3514=EDGE_LOOP('',(#18519,#18520,#18521,#18522));
#3515=EDGE_LOOP('',(#18523,#18524,#18525,#18526));
#3516=EDGE_LOOP('',(#18527,#18528,#18529,#18530,#18531,#18532));
#3517=EDGE_LOOP('',(#18533,#18534,#18535,#18536,#18537,#18538,#18539,#18540,
#18541,#18542,#18543,#18544,#18545,#18546,#18547,#18548,#18549,#18550,#18551,
#18552,#18553,#18554,#18555,#18556,#18557,#18558,#18559,#18560,#18561,#18562,
#18563,#18564,#18565,#18566,#18567,#18568,#18569,#18570,#18571,#18572,#18573,
#18574,#18575,#18576,#18577,#18578,#18579,#18580,#18581,#18582,#18583,#18584,
#18585,#18586,#18587,#18588,#18589,#18590,#18591,#18592,#18593,#18594,#18595,
#18596,#18597,#18598,#18599,#18600,#18601,#18602,#18603,#18604,#18605,#18606,
#18607,#18608,#18609,#18610,#18611,#18612,#18613,#18614,#18615,#18616,#18617,
#18618,#18619,#18620,#18621,#18622,#18623,#18624,#18625,#18626,#18627,#18628,
#18629,#18630,#18631,#18632,#18633,#18634,#18635,#18636,#18637,#18638,#18639,
#18640,#18641,#18642,#18643,#18644,#18645,#18646,#18647,#18648,#18649,#18650,
#18651,#18652,#18653,#18654,#18655,#18656,#18657,#18658,#18659,#18660,#18661,
#18662,#18663,#18664,#18665,#18666,#18667,#18668,#18669,#18670,#18671,#18672,
#18673,#18674,#18675,#18676,#18677,#18678,#18679,#18680,#18681,#18682,#18683,
#18684,#18685,#18686,#18687,#18688,#18689,#18690,#18691,#18692,#18693,#18694,
#18695,#18696,#18697,#18698,#18699,#18700,#18701,#18702,#18703,#18704,#18705,
#18706,#18707,#18708,#18709,#18710,#18711,#18712,#18713,#18714,#18715,#18716,
#18717,#18718,#18719,#18720,#18721,#18722,#18723,#18724,#18725,#18726,#18727,
#18728,#18729,#18730,#18731,#18732,#18733,#18734,#18735,#18736,#18737,#18738,
#18739,#18740,#18741,#18742,#18743,#18744,#18745,#18746,#18747,#18748,#18749,
#18750,#18751,#18752,#18753,#18754,#18755,#18756,#18757,#18758,#18759,#18760,
#18761,#18762,#18763,#18764,#18765,#18766,#18767,#18768,#18769,#18770,#18771,
#18772));
#3518=EDGE_LOOP('',(#18773));
#3519=EDGE_LOOP('',(#18774,#18775,#18776,#18777,#18778,#18779));
#3520=EDGE_LOOP('',(#18780,#18781,#18782,#18783,#18784,#18785));
#3521=EDGE_LOOP('',(#18786,#18787,#18788,#18789,#18790,#18791));
#3522=EDGE_LOOP('',(#18792,#18793,#18794,#18795,#18796,#18797));
#3523=EDGE_LOOP('',(#18798,#18799,#18800,#18801,#18802,#18803));
#3524=EDGE_LOOP('',(#18804,#18805,#18806,#18807,#18808,#18809));
#3525=EDGE_LOOP('',(#18810,#18811,#18812,#18813,#18814,#18815));
#3526=EDGE_LOOP('',(#18816,#18817,#18818,#18819,#18820,#18821));
#3527=EDGE_LOOP('',(#18822,#18823,#18824,#18825,#18826,#18827));
#3528=EDGE_LOOP('',(#18828,#18829,#18830,#18831,#18832,#18833));
#3529=EDGE_LOOP('',(#18834,#18835,#18836,#18837,#18838,#18839));
#3530=EDGE_LOOP('',(#18840,#18841,#18842,#18843,#18844,#18845));
#3531=EDGE_LOOP('',(#18846,#18847,#18848,#18849,#18850,#18851));
#3532=EDGE_LOOP('',(#18852,#18853,#18854,#18855,#18856,#18857));
#3533=EDGE_LOOP('',(#18858,#18859,#18860,#18861,#18862,#18863));
#3534=EDGE_LOOP('',(#18864,#18865,#18866,#18867,#18868,#18869));
#3535=EDGE_LOOP('',(#18870,#18871,#18872,#18873,#18874,#18875));
#3536=EDGE_LOOP('',(#18876,#18877,#18878,#18879,#18880,#18881));
#3537=EDGE_LOOP('',(#18882,#18883,#18884,#18885,#18886,#18887));
#3538=EDGE_LOOP('',(#18888,#18889,#18890,#18891,#18892,#18893));
#3539=EDGE_LOOP('',(#18894,#18895,#18896,#18897,#18898,#18899));
#3540=EDGE_LOOP('',(#18900,#18901,#18902,#18903,#18904,#18905));
#3541=EDGE_LOOP('',(#18906,#18907,#18908,#18909,#18910,#18911));
#3542=EDGE_LOOP('',(#18912,#18913,#18914,#18915));
#3543=EDGE_LOOP('',(#18916,#18917,#18918,#18919));
#3544=EDGE_LOOP('',(#18920,#18921,#18922,#18923));
#3545=EDGE_LOOP('',(#18924,#18925,#18926,#18927));
#3546=EDGE_LOOP('',(#18928,#18929,#18930,#18931));
#3547=EDGE_LOOP('',(#18932,#18933,#18934,#18935,#18936,#18937));
#3548=EDGE_LOOP('',(#18938,#18939,#18940,#18941));
#3549=EDGE_LOOP('',(#18942,#18943,#18944,#18945));
#3550=EDGE_LOOP('',(#18946,#18947,#18948,#18949));
#3551=EDGE_LOOP('',(#18950,#18951,#18952,#18953));
#3552=EDGE_LOOP('',(#18954,#18955,#18956,#18957));
#3553=EDGE_LOOP('',(#18958,#18959,#18960,#18961));
#3554=EDGE_LOOP('',(#18962,#18963,#18964,#18965));
#3555=EDGE_LOOP('',(#18966,#18967,#18968,#18969));
#3556=EDGE_LOOP('',(#18970,#18971,#18972,#18973));
#3557=EDGE_LOOP('',(#18974,#18975,#18976,#18977));
#3558=EDGE_LOOP('',(#18978,#18979,#18980,#18981));
#3559=EDGE_LOOP('',(#18982,#18983,#18984,#18985));
#3560=EDGE_LOOP('',(#18986,#18987,#18988,#18989));
#3561=EDGE_LOOP('',(#18990,#18991,#18992,#18993));
#3562=EDGE_LOOP('',(#18994,#18995,#18996,#18997));
#3563=EDGE_LOOP('',(#18998,#18999,#19000,#19001));
#3564=EDGE_LOOP('',(#19002,#19003,#19004,#19005,#19006,#19007));
#3565=EDGE_LOOP('',(#19008,#19009,#19010,#19011));
#3566=EDGE_LOOP('',(#19012,#19013,#19014,#19015,#19016,#19017));
#3567=EDGE_LOOP('',(#19018,#19019,#19020,#19021,#19022,#19023));
#3568=EDGE_LOOP('',(#19024,#19025,#19026,#19027));
#3569=EDGE_LOOP('',(#19028,#19029,#19030,#19031));
#3570=EDGE_LOOP('',(#19032,#19033,#19034,#19035));
#3571=EDGE_LOOP('',(#19036,#19037,#19038,#19039));
#3572=EDGE_LOOP('',(#19040,#19041,#19042,#19043));
#3573=EDGE_LOOP('',(#19044,#19045,#19046,#19047));
#3574=EDGE_LOOP('',(#19048,#19049,#19050,#19051));
#3575=EDGE_LOOP('',(#19052,#19053,#19054,#19055));
#3576=EDGE_LOOP('',(#19056,#19057,#19058,#19059));
#3577=EDGE_LOOP('',(#19060,#19061,#19062,#19063));
#3578=EDGE_LOOP('',(#19064,#19065,#19066,#19067));
#3579=EDGE_LOOP('',(#19068,#19069,#19070,#19071));
#3580=EDGE_LOOP('',(#19072,#19073,#19074,#19075));
#3581=EDGE_LOOP('',(#19076,#19077,#19078,#19079));
#3582=EDGE_LOOP('',(#19080,#19081,#19082,#19083));
#3583=EDGE_LOOP('',(#19084,#19085,#19086,#19087));
#3584=EDGE_LOOP('',(#19088,#19089,#19090,#19091,#19092,#19093));
#3585=EDGE_LOOP('',(#19094,#19095,#19096,#19097));
#3586=EDGE_LOOP('',(#19098,#19099,#19100,#19101,#19102,#19103));
#3587=EDGE_LOOP('',(#19104,#19105,#19106,#19107,#19108,#19109));
#3588=EDGE_LOOP('',(#19110,#19111,#19112,#19113));
#3589=EDGE_LOOP('',(#19114,#19115,#19116,#19117));
#3590=EDGE_LOOP('',(#19118,#19119,#19120,#19121));
#3591=EDGE_LOOP('',(#19122,#19123,#19124,#19125));
#3592=EDGE_LOOP('',(#19126,#19127,#19128,#19129));
#3593=EDGE_LOOP('',(#19130,#19131,#19132,#19133));
#3594=EDGE_LOOP('',(#19134,#19135,#19136,#19137));
#3595=EDGE_LOOP('',(#19138,#19139,#19140,#19141));
#3596=EDGE_LOOP('',(#19142,#19143,#19144,#19145));
#3597=EDGE_LOOP('',(#19146,#19147,#19148,#19149));
#3598=EDGE_LOOP('',(#19150,#19151,#19152,#19153));
#3599=EDGE_LOOP('',(#19154,#19155,#19156,#19157));
#3600=EDGE_LOOP('',(#19158,#19159,#19160,#19161));
#3601=EDGE_LOOP('',(#19162,#19163,#19164,#19165));
#3602=EDGE_LOOP('',(#19166,#19167,#19168,#19169));
#3603=EDGE_LOOP('',(#19170,#19171,#19172,#19173));
#3604=EDGE_LOOP('',(#19174,#19175,#19176,#19177,#19178,#19179));
#3605=EDGE_LOOP('',(#19180,#19181,#19182,#19183));
#3606=EDGE_LOOP('',(#19184,#19185,#19186,#19187,#19188,#19189));
#3607=EDGE_LOOP('',(#19190,#19191,#19192,#19193,#19194,#19195));
#3608=EDGE_LOOP('',(#19196,#19197,#19198,#19199));
#3609=EDGE_LOOP('',(#19200,#19201,#19202,#19203));
#3610=EDGE_LOOP('',(#19204,#19205,#19206,#19207));
#3611=EDGE_LOOP('',(#19208,#19209,#19210,#19211));
#3612=EDGE_LOOP('',(#19212,#19213,#19214,#19215));
#3613=EDGE_LOOP('',(#19216,#19217,#19218,#19219));
#3614=EDGE_LOOP('',(#19220,#19221,#19222,#19223));
#3615=EDGE_LOOP('',(#19224,#19225,#19226,#19227));
#3616=EDGE_LOOP('',(#19228,#19229,#19230,#19231));
#3617=EDGE_LOOP('',(#19232,#19233,#19234,#19235));
#3618=EDGE_LOOP('',(#19236,#19237,#19238,#19239));
#3619=EDGE_LOOP('',(#19240,#19241,#19242,#19243));
#3620=EDGE_LOOP('',(#19244,#19245,#19246,#19247));
#3621=EDGE_LOOP('',(#19248,#19249,#19250,#19251));
#3622=EDGE_LOOP('',(#19252,#19253,#19254,#19255));
#3623=EDGE_LOOP('',(#19256,#19257,#19258,#19259));
#3624=EDGE_LOOP('',(#19260,#19261,#19262,#19263,#19264,#19265));
#3625=EDGE_LOOP('',(#19266,#19267,#19268,#19269));
#3626=EDGE_LOOP('',(#19270,#19271,#19272,#19273,#19274,#19275));
#3627=EDGE_LOOP('',(#19276,#19277,#19278,#19279,#19280,#19281));
#3628=EDGE_LOOP('',(#19282,#19283,#19284,#19285));
#3629=EDGE_LOOP('',(#19286,#19287,#19288,#19289));
#3630=EDGE_LOOP('',(#19290,#19291,#19292,#19293));
#3631=EDGE_LOOP('',(#19294,#19295,#19296,#19297));
#3632=EDGE_LOOP('',(#19298,#19299,#19300,#19301));
#3633=EDGE_LOOP('',(#19302,#19303,#19304,#19305));
#3634=EDGE_LOOP('',(#19306,#19307,#19308,#19309));
#3635=EDGE_LOOP('',(#19310,#19311,#19312,#19313));
#3636=EDGE_LOOP('',(#19314,#19315,#19316,#19317));
#3637=EDGE_LOOP('',(#19318,#19319,#19320,#19321));
#3638=EDGE_LOOP('',(#19322,#19323,#19324,#19325));
#3639=EDGE_LOOP('',(#19326,#19327,#19328,#19329));
#3640=EDGE_LOOP('',(#19330,#19331,#19332,#19333));
#3641=EDGE_LOOP('',(#19334,#19335,#19336,#19337));
#3642=EDGE_LOOP('',(#19338,#19339,#19340,#19341));
#3643=EDGE_LOOP('',(#19342,#19343,#19344,#19345));
#3644=EDGE_LOOP('',(#19346,#19347,#19348,#19349,#19350,#19351));
#3645=EDGE_LOOP('',(#19352,#19353,#19354,#19355));
#3646=EDGE_LOOP('',(#19356,#19357,#19358,#19359,#19360,#19361));
#3647=EDGE_LOOP('',(#19362,#19363,#19364,#19365,#19366,#19367));
#3648=EDGE_LOOP('',(#19368,#19369,#19370,#19371));
#3649=EDGE_LOOP('',(#19372,#19373,#19374,#19375));
#3650=EDGE_LOOP('',(#19376,#19377,#19378,#19379));
#3651=EDGE_LOOP('',(#19380,#19381,#19382,#19383));
#3652=EDGE_LOOP('',(#19384,#19385,#19386,#19387));
#3653=EDGE_LOOP('',(#19388,#19389,#19390,#19391));
#3654=EDGE_LOOP('',(#19392,#19393,#19394,#19395));
#3655=EDGE_LOOP('',(#19396,#19397,#19398,#19399));
#3656=EDGE_LOOP('',(#19400,#19401,#19402,#19403));
#3657=EDGE_LOOP('',(#19404,#19405,#19406,#19407));
#3658=EDGE_LOOP('',(#19408,#19409,#19410,#19411));
#3659=EDGE_LOOP('',(#19412,#19413,#19414,#19415));
#3660=EDGE_LOOP('',(#19416,#19417,#19418,#19419));
#3661=EDGE_LOOP('',(#19420,#19421,#19422,#19423));
#3662=EDGE_LOOP('',(#19424,#19425,#19426,#19427));
#3663=EDGE_LOOP('',(#19428,#19429,#19430,#19431));
#3664=EDGE_LOOP('',(#19432,#19433,#19434,#19435,#19436,#19437));
#3665=EDGE_LOOP('',(#19438,#19439,#19440,#19441));
#3666=EDGE_LOOP('',(#19442,#19443,#19444,#19445,#19446,#19447));
#3667=EDGE_LOOP('',(#19448,#19449,#19450,#19451,#19452,#19453));
#3668=EDGE_LOOP('',(#19454,#19455,#19456,#19457));
#3669=EDGE_LOOP('',(#19458,#19459,#19460,#19461));
#3670=EDGE_LOOP('',(#19462,#19463,#19464,#19465));
#3671=EDGE_LOOP('',(#19466,#19467,#19468,#19469));
#3672=EDGE_LOOP('',(#19470,#19471,#19472,#19473));
#3673=EDGE_LOOP('',(#19474,#19475,#19476,#19477));
#3674=EDGE_LOOP('',(#19478,#19479,#19480,#19481));
#3675=EDGE_LOOP('',(#19482,#19483,#19484,#19485));
#3676=EDGE_LOOP('',(#19486,#19487,#19488,#19489));
#3677=EDGE_LOOP('',(#19490,#19491,#19492,#19493));
#3678=EDGE_LOOP('',(#19494,#19495,#19496,#19497));
#3679=EDGE_LOOP('',(#19498,#19499,#19500,#19501));
#3680=EDGE_LOOP('',(#19502,#19503,#19504,#19505));
#3681=EDGE_LOOP('',(#19506,#19507,#19508,#19509));
#3682=EDGE_LOOP('',(#19510,#19511,#19512,#19513));
#3683=EDGE_LOOP('',(#19514,#19515,#19516,#19517));
#3684=EDGE_LOOP('',(#19518,#19519,#19520,#19521,#19522,#19523));
#3685=EDGE_LOOP('',(#19524,#19525,#19526,#19527));
#3686=EDGE_LOOP('',(#19528,#19529,#19530,#19531,#19532,#19533));
#3687=EDGE_LOOP('',(#19534,#19535,#19536,#19537,#19538,#19539));
#3688=EDGE_LOOP('',(#19540,#19541,#19542,#19543));
#3689=EDGE_LOOP('',(#19544,#19545,#19546,#19547));
#3690=EDGE_LOOP('',(#19548,#19549,#19550,#19551));
#3691=EDGE_LOOP('',(#19552,#19553,#19554,#19555));
#3692=EDGE_LOOP('',(#19556,#19557,#19558,#19559));
#3693=EDGE_LOOP('',(#19560,#19561,#19562,#19563));
#3694=EDGE_LOOP('',(#19564,#19565,#19566,#19567));
#3695=EDGE_LOOP('',(#19568,#19569,#19570,#19571));
#3696=EDGE_LOOP('',(#19572,#19573,#19574,#19575));
#3697=EDGE_LOOP('',(#19576,#19577,#19578,#19579));
#3698=EDGE_LOOP('',(#19580,#19581,#19582,#19583));
#3699=EDGE_LOOP('',(#19584,#19585,#19586,#19587));
#3700=EDGE_LOOP('',(#19588,#19589,#19590,#19591));
#3701=EDGE_LOOP('',(#19592,#19593,#19594,#19595));
#3702=EDGE_LOOP('',(#19596,#19597,#19598,#19599));
#3703=EDGE_LOOP('',(#19600,#19601,#19602,#19603));
#3704=EDGE_LOOP('',(#19604,#19605,#19606,#19607,#19608,#19609));
#3705=EDGE_LOOP('',(#19610,#19611,#19612,#19613));
#3706=EDGE_LOOP('',(#19614,#19615,#19616,#19617,#19618,#19619));
#3707=EDGE_LOOP('',(#19620,#19621,#19622,#19623,#19624,#19625));
#3708=EDGE_LOOP('',(#19626,#19627,#19628,#19629));
#3709=EDGE_LOOP('',(#19630,#19631,#19632,#19633));
#3710=EDGE_LOOP('',(#19634,#19635,#19636,#19637));
#3711=EDGE_LOOP('',(#19638,#19639,#19640,#19641));
#3712=EDGE_LOOP('',(#19642,#19643,#19644,#19645));
#3713=EDGE_LOOP('',(#19646,#19647,#19648,#19649));
#3714=EDGE_LOOP('',(#19650,#19651,#19652,#19653));
#3715=EDGE_LOOP('',(#19654,#19655,#19656,#19657));
#3716=EDGE_LOOP('',(#19658,#19659,#19660,#19661));
#3717=EDGE_LOOP('',(#19662,#19663,#19664,#19665));
#3718=EDGE_LOOP('',(#19666,#19667,#19668,#19669));
#3719=EDGE_LOOP('',(#19670,#19671,#19672,#19673));
#3720=EDGE_LOOP('',(#19674,#19675,#19676,#19677));
#3721=EDGE_LOOP('',(#19678,#19679,#19680,#19681));
#3722=EDGE_LOOP('',(#19682,#19683,#19684,#19685));
#3723=EDGE_LOOP('',(#19686,#19687,#19688,#19689));
#3724=EDGE_LOOP('',(#19690,#19691,#19692,#19693,#19694,#19695));
#3725=EDGE_LOOP('',(#19696,#19697,#19698,#19699));
#3726=EDGE_LOOP('',(#19700,#19701,#19702,#19703,#19704,#19705));
#3727=EDGE_LOOP('',(#19706,#19707,#19708,#19709,#19710,#19711));
#3728=EDGE_LOOP('',(#19712,#19713,#19714,#19715));
#3729=EDGE_LOOP('',(#19716,#19717,#19718,#19719));
#3730=EDGE_LOOP('',(#19720,#19721,#19722,#19723));
#3731=EDGE_LOOP('',(#19724,#19725,#19726,#19727));
#3732=EDGE_LOOP('',(#19728,#19729,#19730,#19731));
#3733=EDGE_LOOP('',(#19732,#19733,#19734,#19735));
#3734=EDGE_LOOP('',(#19736,#19737,#19738,#19739));
#3735=EDGE_LOOP('',(#19740,#19741,#19742,#19743));
#3736=EDGE_LOOP('',(#19744,#19745,#19746,#19747));
#3737=EDGE_LOOP('',(#19748,#19749,#19750,#19751));
#3738=EDGE_LOOP('',(#19752,#19753,#19754,#19755));
#3739=EDGE_LOOP('',(#19756,#19757,#19758,#19759));
#3740=EDGE_LOOP('',(#19760,#19761,#19762,#19763));
#3741=EDGE_LOOP('',(#19764,#19765,#19766,#19767));
#3742=EDGE_LOOP('',(#19768,#19769,#19770,#19771));
#3743=EDGE_LOOP('',(#19772,#19773,#19774,#19775));
#3744=EDGE_LOOP('',(#19776,#19777,#19778,#19779,#19780,#19781));
#3745=EDGE_LOOP('',(#19782,#19783,#19784,#19785));
#3746=EDGE_LOOP('',(#19786,#19787,#19788,#19789,#19790,#19791));
#3747=EDGE_LOOP('',(#19792,#19793,#19794,#19795,#19796,#19797));
#3748=EDGE_LOOP('',(#19798,#19799,#19800,#19801));
#3749=EDGE_LOOP('',(#19802,#19803,#19804,#19805));
#3750=EDGE_LOOP('',(#19806,#19807,#19808,#19809));
#3751=EDGE_LOOP('',(#19810,#19811,#19812,#19813));
#3752=EDGE_LOOP('',(#19814,#19815,#19816,#19817));
#3753=EDGE_LOOP('',(#19818,#19819,#19820,#19821));
#3754=EDGE_LOOP('',(#19822,#19823,#19824,#19825));
#3755=EDGE_LOOP('',(#19826,#19827,#19828,#19829));
#3756=EDGE_LOOP('',(#19830,#19831,#19832,#19833));
#3757=EDGE_LOOP('',(#19834,#19835,#19836,#19837));
#3758=EDGE_LOOP('',(#19838,#19839,#19840,#19841));
#3759=EDGE_LOOP('',(#19842,#19843,#19844,#19845));
#3760=EDGE_LOOP('',(#19846,#19847,#19848,#19849));
#3761=EDGE_LOOP('',(#19850,#19851,#19852,#19853));
#3762=EDGE_LOOP('',(#19854,#19855,#19856,#19857));
#3763=EDGE_LOOP('',(#19858,#19859,#19860,#19861));
#3764=EDGE_LOOP('',(#19862,#19863,#19864,#19865,#19866,#19867));
#3765=EDGE_LOOP('',(#19868,#19869,#19870,#19871));
#3766=EDGE_LOOP('',(#19872,#19873,#19874,#19875,#19876,#19877));
#3767=EDGE_LOOP('',(#19878,#19879,#19880,#19881,#19882,#19883));
#3768=EDGE_LOOP('',(#19884,#19885,#19886,#19887));
#3769=EDGE_LOOP('',(#19888,#19889,#19890,#19891));
#3770=EDGE_LOOP('',(#19892,#19893,#19894,#19895));
#3771=EDGE_LOOP('',(#19896,#19897,#19898,#19899));
#3772=EDGE_LOOP('',(#19900,#19901,#19902,#19903));
#3773=EDGE_LOOP('',(#19904,#19905,#19906,#19907));
#3774=EDGE_LOOP('',(#19908,#19909,#19910,#19911));
#3775=EDGE_LOOP('',(#19912,#19913,#19914,#19915));
#3776=EDGE_LOOP('',(#19916,#19917,#19918,#19919));
#3777=EDGE_LOOP('',(#19920,#19921,#19922,#19923));
#3778=EDGE_LOOP('',(#19924,#19925,#19926,#19927));
#3779=EDGE_LOOP('',(#19928,#19929,#19930,#19931));
#3780=EDGE_LOOP('',(#19932,#19933,#19934,#19935));
#3781=EDGE_LOOP('',(#19936,#19937,#19938,#19939));
#3782=EDGE_LOOP('',(#19940,#19941,#19942,#19943));
#3783=EDGE_LOOP('',(#19944,#19945,#19946,#19947));
#3784=EDGE_LOOP('',(#19948,#19949,#19950,#19951,#19952,#19953));
#3785=EDGE_LOOP('',(#19954,#19955,#19956,#19957));
#3786=EDGE_LOOP('',(#19958,#19959,#19960,#19961,#19962,#19963));
#3787=EDGE_LOOP('',(#19964,#19965,#19966,#19967));
#3788=EDGE_LOOP('',(#19968));
#3789=EDGE_LOOP('',(#19969,#19970,#19971,#19972));
#3790=EDGE_LOOP('',(#19973,#19974,#19975,#19976));
#3791=EDGE_LOOP('',(#19977,#19978,#19979,#19980));
#3792=EDGE_LOOP('',(#19981));
#3793=EDGE_LOOP('',(#19982));
#3794=EDGE_LOOP('',(#19983,#19984,#19985,#19986));
#3795=EDGE_LOOP('',(#19987));
#4867=LINE('',#36031,#7736);
#4868=LINE('',#36033,#7737);
#4869=LINE('',#36035,#7738);
#4870=LINE('',#36037,#7739);
#4871=LINE('',#36039,#7740);
#4872=LINE('',#36040,#7741);
#4873=LINE('',#36043,#7742);
#4874=LINE('',#36045,#7743);
#4875=LINE('',#36047,#7744);
#4876=LINE('',#36049,#7745);
#4877=LINE('',#36051,#7746);
#4878=LINE('',#36053,#7747);
#4879=LINE('',#36055,#7748);
#4880=LINE('',#36057,#7749);
#4881=LINE('',#36059,#7750);
#4882=LINE('',#36061,#7751);
#4883=LINE('',#36063,#7752);
#4884=LINE('',#36065,#7753);
#4885=LINE('',#36067,#7754);
#4886=LINE('',#36069,#7755);
#4887=LINE('',#36071,#7756);
#4888=LINE('',#36073,#7757);
#4889=LINE('',#36075,#7758);
#4890=LINE('',#36077,#7759);
#4891=LINE('',#36079,#7760);
#4892=LINE('',#36081,#7761);
#4893=LINE('',#36083,#7762);
#4894=LINE('',#36085,#7763);
#4895=LINE('',#36087,#7764);
#4896=LINE('',#36089,#7765);
#4897=LINE('',#36091,#7766);
#4898=LINE('',#36093,#7767);
#4899=LINE('',#36095,#7768);
#4900=LINE('',#36097,#7769);
#4901=LINE('',#36099,#7770);
#4902=LINE('',#36101,#7771);
#4903=LINE('',#36103,#7772);
#4904=LINE('',#36105,#7773);
#4905=LINE('',#36107,#7774);
#4906=LINE('',#36109,#7775);
#4907=LINE('',#36111,#7776);
#4908=LINE('',#36113,#7777);
#4909=LINE('',#36115,#7778);
#4910=LINE('',#36117,#7779);
#4911=LINE('',#36119,#7780);
#4912=LINE('',#36121,#7781);
#4913=LINE('',#36123,#7782);
#4914=LINE('',#36125,#7783);
#4915=LINE('',#36127,#7784);
#4916=LINE('',#36129,#7785);
#4917=LINE('',#36131,#7786);
#4918=LINE('',#36133,#7787);
#4919=LINE('',#36135,#7788);
#4920=LINE('',#36137,#7789);
#4921=LINE('',#36139,#7790);
#4922=LINE('',#36141,#7791);
#4923=LINE('',#36143,#7792);
#4924=LINE('',#36145,#7793);
#4925=LINE('',#36147,#7794);
#4926=LINE('',#36149,#7795);
#4927=LINE('',#36151,#7796);
#4928=LINE('',#36153,#7797);
#4929=LINE('',#36155,#7798);
#4930=LINE('',#36157,#7799);
#4931=LINE('',#36159,#7800);
#4932=LINE('',#36161,#7801);
#4933=LINE('',#36163,#7802);
#4934=LINE('',#36165,#7803);
#4935=LINE('',#36167,#7804);
#4936=LINE('',#36169,#7805);
#4937=LINE('',#36171,#7806);
#4938=LINE('',#36173,#7807);
#4939=LINE('',#36175,#7808);
#4940=LINE('',#36177,#7809);
#4941=LINE('',#36179,#7810);
#4942=LINE('',#36181,#7811);
#4943=LINE('',#36183,#7812);
#4944=LINE('',#36185,#7813);
#4945=LINE('',#36187,#7814);
#4946=LINE('',#36189,#7815);
#4947=LINE('',#36191,#7816);
#4948=LINE('',#36193,#7817);
#4949=LINE('',#36195,#7818);
#4950=LINE('',#36197,#7819);
#4951=LINE('',#36199,#7820);
#4952=LINE('',#36201,#7821);
#4953=LINE('',#36203,#7822);
#4954=LINE('',#36205,#7823);
#4955=LINE('',#36207,#7824);
#4956=LINE('',#36209,#7825);
#4957=LINE('',#36211,#7826);
#4958=LINE('',#36213,#7827);
#4959=LINE('',#36215,#7828);
#4960=LINE('',#36217,#7829);
#4961=LINE('',#36219,#7830);
#4962=LINE('',#36221,#7831);
#4963=LINE('',#36223,#7832);
#4964=LINE('',#36225,#7833);
#4965=LINE('',#36227,#7834);
#4966=LINE('',#36229,#7835);
#4967=LINE('',#36231,#7836);
#4968=LINE('',#36233,#7837);
#4969=LINE('',#36235,#7838);
#4970=LINE('',#36237,#7839);
#4971=LINE('',#36239,#7840);
#4972=LINE('',#36241,#7841);
#4973=LINE('',#36243,#7842);
#4974=LINE('',#36245,#7843);
#4975=LINE('',#36247,#7844);
#4976=LINE('',#36249,#7845);
#4977=LINE('',#36251,#7846);
#4978=LINE('',#36253,#7847);
#4979=LINE('',#36255,#7848);
#4980=LINE('',#36257,#7849);
#4981=LINE('',#36259,#7850);
#4982=LINE('',#36261,#7851);
#4983=LINE('',#36263,#7852);
#4984=LINE('',#36265,#7853);
#4985=LINE('',#36267,#7854);
#4986=LINE('',#36269,#7855);
#4987=LINE('',#36271,#7856);
#4988=LINE('',#36273,#7857);
#4989=LINE('',#36275,#7858);
#4990=LINE('',#36277,#7859);
#4991=LINE('',#36279,#7860);
#4992=LINE('',#36281,#7861);
#4993=LINE('',#36283,#7862);
#4994=LINE('',#36285,#7863);
#4995=LINE('',#36287,#7864);
#4996=LINE('',#36289,#7865);
#4997=LINE('',#36291,#7866);
#4998=LINE('',#36293,#7867);
#4999=LINE('',#36295,#7868);
#5000=LINE('',#36297,#7869);
#5001=LINE('',#36299,#7870);
#5002=LINE('',#36301,#7871);
#5003=LINE('',#36303,#7872);
#5004=LINE('',#36305,#7873);
#5005=LINE('',#36307,#7874);
#5006=LINE('',#36309,#7875);
#5007=LINE('',#36311,#7876);
#5008=LINE('',#36313,#7877);
#5009=LINE('',#36315,#7878);
#5010=LINE('',#36317,#7879);
#5011=LINE('',#36319,#7880);
#5012=LINE('',#36321,#7881);
#5013=LINE('',#36323,#7882);
#5014=LINE('',#36325,#7883);
#5015=LINE('',#36327,#7884);
#5016=LINE('',#36329,#7885);
#5017=LINE('',#36331,#7886);
#5018=LINE('',#36333,#7887);
#5019=LINE('',#36335,#7888);
#5020=LINE('',#36337,#7889);
#5021=LINE('',#36339,#7890);
#5022=LINE('',#36341,#7891);
#5023=LINE('',#36343,#7892);
#5024=LINE('',#36345,#7893);
#5025=LINE('',#36347,#7894);
#5026=LINE('',#36349,#7895);
#5027=LINE('',#36351,#7896);
#5028=LINE('',#36353,#7897);
#5029=LINE('',#36355,#7898);
#5030=LINE('',#36357,#7899);
#5031=LINE('',#36359,#7900);
#5032=LINE('',#36361,#7901);
#5033=LINE('',#36363,#7902);
#5034=LINE('',#36365,#7903);
#5035=LINE('',#36367,#7904);
#5036=LINE('',#36369,#7905);
#5037=LINE('',#36371,#7906);
#5038=LINE('',#36373,#7907);
#5039=LINE('',#36375,#7908);
#5040=LINE('',#36377,#7909);
#5041=LINE('',#36379,#7910);
#5042=LINE('',#36381,#7911);
#5043=LINE('',#36383,#7912);
#5044=LINE('',#36385,#7913);
#5045=LINE('',#36387,#7914);
#5046=LINE('',#36389,#7915);
#5047=LINE('',#36391,#7916);
#5048=LINE('',#36393,#7917);
#5049=LINE('',#36395,#7918);
#5050=LINE('',#36397,#7919);
#5051=LINE('',#36399,#7920);
#5052=LINE('',#36401,#7921);
#5053=LINE('',#36403,#7922);
#5054=LINE('',#36405,#7923);
#5055=LINE('',#36407,#7924);
#5056=LINE('',#36409,#7925);
#5057=LINE('',#36411,#7926);
#5058=LINE('',#36413,#7927);
#5059=LINE('',#36415,#7928);
#5060=LINE('',#36417,#7929);
#5061=LINE('',#36419,#7930);
#5062=LINE('',#36421,#7931);
#5063=LINE('',#36423,#7932);
#5064=LINE('',#36425,#7933);
#5065=LINE('',#36427,#7934);
#5066=LINE('',#36429,#7935);
#5067=LINE('',#36431,#7936);
#5068=LINE('',#36433,#7937);
#5069=LINE('',#36435,#7938);
#5070=LINE('',#36437,#7939);
#5071=LINE('',#36439,#7940);
#5072=LINE('',#36441,#7941);
#5073=LINE('',#36443,#7942);
#5074=LINE('',#36445,#7943);
#5075=LINE('',#36447,#7944);
#5076=LINE('',#36449,#7945);
#5077=LINE('',#36451,#7946);
#5078=LINE('',#36453,#7947);
#5079=LINE('',#36455,#7948);
#5080=LINE('',#36457,#7949);
#5081=LINE('',#36459,#7950);
#5082=LINE('',#36461,#7951);
#5083=LINE('',#36463,#7952);
#5084=LINE('',#36465,#7953);
#5085=LINE('',#36467,#7954);
#5086=LINE('',#36469,#7955);
#5087=LINE('',#36471,#7956);
#5088=LINE('',#36473,#7957);
#5089=LINE('',#36475,#7958);
#5090=LINE('',#36477,#7959);
#5091=LINE('',#36479,#7960);
#5092=LINE('',#36481,#7961);
#5093=LINE('',#36483,#7962);
#5094=LINE('',#36485,#7963);
#5095=LINE('',#36487,#7964);
#5096=LINE('',#36489,#7965);
#5097=LINE('',#36491,#7966);
#5098=LINE('',#36493,#7967);
#5099=LINE('',#36495,#7968);
#5100=LINE('',#36497,#7969);
#5101=LINE('',#36499,#7970);
#5102=LINE('',#36501,#7971);
#5103=LINE('',#36503,#7972);
#5104=LINE('',#36505,#7973);
#5105=LINE('',#36507,#7974);
#5106=LINE('',#36509,#7975);
#5107=LINE('',#36511,#7976);
#5108=LINE('',#36513,#7977);
#5109=LINE('',#36515,#7978);
#5110=LINE('',#36517,#7979);
#5111=LINE('',#36518,#7980);
#5112=LINE('',#36523,#7981);
#5113=LINE('',#36525,#7982);
#5114=LINE('',#36527,#7983);
#5115=LINE('',#36528,#7984);
#5116=LINE('',#36531,#7985);
#5117=LINE('',#36532,#7986);
#5118=LINE('',#36535,#7987);
#5119=LINE('',#36537,#7988);
#5120=LINE('',#36539,#7989);
#5121=LINE('',#36541,#7990);
#5122=LINE('',#36542,#7991);
#5123=LINE('',#36545,#7992);
#5124=LINE('',#36547,#7993);
#5125=LINE('',#36549,#7994);
#5126=LINE('',#36550,#7995);
#5127=LINE('',#36553,#7996);
#5128=LINE('',#36554,#7997);
#5129=LINE('',#36557,#7998);
#5130=LINE('',#36559,#7999);
#5131=LINE('',#36561,#8000);
#5132=LINE('',#36563,#8001);
#5133=LINE('',#36564,#8002);
#5134=LINE('',#36567,#8003);
#5135=LINE('',#36569,#8004);
#5136=LINE('',#36571,#8005);
#5137=LINE('',#36572,#8006);
#5138=LINE('',#36575,#8007);
#5139=LINE('',#36576,#8008);
#5140=LINE('',#36579,#8009);
#5141=LINE('',#36581,#8010);
#5142=LINE('',#36583,#8011);
#5143=LINE('',#36585,#8012);
#5144=LINE('',#36586,#8013);
#5145=LINE('',#36589,#8014);
#5146=LINE('',#36591,#8015);
#5147=LINE('',#36593,#8016);
#5148=LINE('',#36594,#8017);
#5149=LINE('',#36597,#8018);
#5150=LINE('',#36598,#8019);
#5151=LINE('',#36601,#8020);
#5152=LINE('',#36603,#8021);
#5153=LINE('',#36605,#8022);
#5154=LINE('',#36607,#8023);
#5155=LINE('',#36608,#8024);
#5156=LINE('',#36611,#8025);
#5157=LINE('',#36613,#8026);
#5158=LINE('',#36615,#8027);
#5159=LINE('',#36616,#8028);
#5160=LINE('',#36619,#8029);
#5161=LINE('',#36620,#8030);
#5162=LINE('',#36623,#8031);
#5163=LINE('',#36625,#8032);
#5164=LINE('',#36627,#8033);
#5165=LINE('',#36629,#8034);
#5166=LINE('',#36630,#8035);
#5167=LINE('',#36633,#8036);
#5168=LINE('',#36635,#8037);
#5169=LINE('',#36637,#8038);
#5170=LINE('',#36638,#8039);
#5171=LINE('',#36641,#8040);
#5172=LINE('',#36642,#8041);
#5173=LINE('',#36645,#8042);
#5174=LINE('',#36647,#8043);
#5175=LINE('',#36649,#8044);
#5176=LINE('',#36651,#8045);
#5177=LINE('',#36652,#8046);
#5178=LINE('',#36655,#8047);
#5179=LINE('',#36657,#8048);
#5180=LINE('',#36659,#8049);
#5181=LINE('',#36660,#8050);
#5182=LINE('',#36663,#8051);
#5183=LINE('',#36664,#8052);
#5184=LINE('',#36667,#8053);
#5185=LINE('',#36669,#8054);
#5186=LINE('',#36671,#8055);
#5187=LINE('',#36673,#8056);
#5188=LINE('',#36674,#8057);
#5189=LINE('',#36677,#8058);
#5190=LINE('',#36679,#8059);
#5191=LINE('',#36681,#8060);
#5192=LINE('',#36682,#8061);
#5193=LINE('',#36685,#8062);
#5194=LINE('',#36686,#8063);
#5195=LINE('',#36689,#8064);
#5196=LINE('',#36691,#8065);
#5197=LINE('',#36693,#8066);
#5198=LINE('',#36695,#8067);
#5199=LINE('',#36696,#8068);
#5200=LINE('',#36699,#8069);
#5201=LINE('',#36701,#8070);
#5202=LINE('',#36703,#8071);
#5203=LINE('',#36704,#8072);
#5204=LINE('',#36707,#8073);
#5205=LINE('',#36708,#8074);
#5206=LINE('',#36711,#8075);
#5207=LINE('',#36713,#8076);
#5208=LINE('',#36715,#8077);
#5209=LINE('',#36717,#8078);
#5210=LINE('',#36718,#8079);
#5211=LINE('',#36721,#8080);
#5212=LINE('',#36723,#8081);
#5213=LINE('',#36725,#8082);
#5214=LINE('',#36726,#8083);
#5215=LINE('',#36729,#8084);
#5216=LINE('',#36730,#8085);
#5217=LINE('',#36733,#8086);
#5218=LINE('',#36735,#8087);
#5219=LINE('',#36737,#8088);
#5220=LINE('',#36739,#8089);
#5221=LINE('',#36740,#8090);
#5222=LINE('',#36743,#8091);
#5223=LINE('',#36745,#8092);
#5224=LINE('',#36747,#8093);
#5225=LINE('',#36748,#8094);
#5226=LINE('',#36751,#8095);
#5227=LINE('',#36752,#8096);
#5228=LINE('',#36755,#8097);
#5229=LINE('',#36757,#8098);
#5230=LINE('',#36759,#8099);
#5231=LINE('',#36761,#8100);
#5232=LINE('',#36762,#8101);
#5233=LINE('',#36765,#8102);
#5234=LINE('',#36767,#8103);
#5235=LINE('',#36769,#8104);
#5236=LINE('',#36770,#8105);
#5237=LINE('',#36773,#8106);
#5238=LINE('',#36774,#8107);
#5239=LINE('',#36778,#8108);
#5240=LINE('',#36780,#8109);
#5241=LINE('',#36781,#8110);
#5242=LINE('',#36783,#8111);
#5243=LINE('',#36784,#8112);
#5244=LINE('',#36787,#8113);
#5245=LINE('',#36789,#8114);
#5246=LINE('',#36790,#8115);
#5247=LINE('',#36793,#8116);
#5248=LINE('',#36794,#8117);
#5249=LINE('',#36798,#8118);
#5250=LINE('',#36800,#8119);
#5251=LINE('',#36801,#8120);
#5252=LINE('',#36803,#8121);
#5253=LINE('',#36804,#8122);
#5254=LINE('',#36807,#8123);
#5255=LINE('',#36809,#8124);
#5256=LINE('',#36810,#8125);
#5257=LINE('',#36813,#8126);
#5258=LINE('',#36814,#8127);
#5259=LINE('',#36818,#8128);
#5260=LINE('',#36820,#8129);
#5261=LINE('',#36821,#8130);
#5262=LINE('',#36823,#8131);
#5263=LINE('',#36824,#8132);
#5264=LINE('',#36827,#8133);
#5265=LINE('',#36829,#8134);
#5266=LINE('',#36830,#8135);
#5267=LINE('',#36833,#8136);
#5268=LINE('',#36834,#8137);
#5269=LINE('',#36838,#8138);
#5270=LINE('',#36840,#8139);
#5271=LINE('',#36841,#8140);
#5272=LINE('',#36843,#8141);
#5273=LINE('',#36844,#8142);
#5274=LINE('',#36847,#8143);
#5275=LINE('',#36849,#8144);
#5276=LINE('',#36850,#8145);
#5277=LINE('',#36853,#8146);
#5278=LINE('',#36854,#8147);
#5279=LINE('',#36858,#8148);
#5280=LINE('',#36860,#8149);
#5281=LINE('',#36861,#8150);
#5282=LINE('',#36863,#8151);
#5283=LINE('',#36864,#8152);
#5284=LINE('',#36867,#8153);
#5285=LINE('',#36869,#8154);
#5286=LINE('',#36870,#8155);
#5287=LINE('',#36873,#8156);
#5288=LINE('',#36874,#8157);
#5289=LINE('',#36878,#8158);
#5290=LINE('',#36880,#8159);
#5291=LINE('',#36881,#8160);
#5292=LINE('',#36883,#8161);
#5293=LINE('',#36884,#8162);
#5294=LINE('',#36887,#8163);
#5295=LINE('',#36889,#8164);
#5296=LINE('',#36890,#8165);
#5297=LINE('',#36893,#8166);
#5298=LINE('',#36894,#8167);
#5299=LINE('',#36898,#8168);
#5300=LINE('',#36900,#8169);
#5301=LINE('',#36901,#8170);
#5302=LINE('',#36903,#8171);
#5303=LINE('',#36904,#8172);
#5304=LINE('',#36907,#8173);
#5305=LINE('',#36909,#8174);
#5306=LINE('',#36910,#8175);
#5307=LINE('',#36913,#8176);
#5308=LINE('',#36914,#8177);
#5309=LINE('',#36918,#8178);
#5310=LINE('',#36920,#8179);
#5311=LINE('',#36921,#8180);
#5312=LINE('',#36923,#8181);
#5313=LINE('',#36924,#8182);
#5314=LINE('',#36927,#8183);
#5315=LINE('',#36929,#8184);
#5316=LINE('',#36930,#8185);
#5317=LINE('',#36933,#8186);
#5318=LINE('',#36934,#8187);
#5319=LINE('',#36938,#8188);
#5320=LINE('',#36940,#8189);
#5321=LINE('',#36941,#8190);
#5322=LINE('',#36943,#8191);
#5323=LINE('',#36944,#8192);
#5324=LINE('',#36947,#8193);
#5325=LINE('',#36949,#8194);
#5326=LINE('',#36950,#8195);
#5327=LINE('',#36953,#8196);
#5328=LINE('',#36954,#8197);
#5329=LINE('',#36958,#8198);
#5330=LINE('',#36960,#8199);
#5331=LINE('',#36961,#8200);
#5332=LINE('',#36963,#8201);
#5333=LINE('',#36964,#8202);
#5334=LINE('',#36967,#8203);
#5335=LINE('',#36969,#8204);
#5336=LINE('',#36970,#8205);
#5337=LINE('',#36973,#8206);
#5338=LINE('',#36974,#8207);
#5339=LINE('',#36978,#8208);
#5340=LINE('',#36980,#8209);
#5341=LINE('',#36981,#8210);
#5342=LINE('',#36983,#8211);
#5343=LINE('',#36984,#8212);
#5344=LINE('',#36987,#8213);
#5345=LINE('',#36989,#8214);
#5346=LINE('',#36990,#8215);
#5347=LINE('',#36993,#8216);
#5348=LINE('',#36994,#8217);
#5349=LINE('',#36998,#8218);
#5350=LINE('',#37000,#8219);
#5351=LINE('',#37001,#8220);
#5352=LINE('',#37003,#8221);
#5353=LINE('',#37004,#8222);
#5354=LINE('',#37007,#8223);
#5355=LINE('',#37009,#8224);
#5356=LINE('',#37010,#8225);
#5357=LINE('',#37013,#8226);
#5358=LINE('',#37014,#8227);
#5359=LINE('',#37017,#8228);
#5360=LINE('',#37019,#8229);
#5361=LINE('',#37021,#8230);
#5362=LINE('',#37022,#8231);
#5363=LINE('',#37025,#8232);
#5364=LINE('',#37027,#8233);
#5365=LINE('',#37029,#8234);
#5366=LINE('',#37031,#8235);
#5367=LINE('',#37033,#8236);
#5368=LINE('',#37035,#8237);
#5369=LINE('',#37037,#8238);
#5370=LINE('',#37039,#8239);
#5371=LINE('',#37041,#8240);
#5372=LINE('',#37043,#8241);
#5373=LINE('',#37045,#8242);
#5374=LINE('',#37047,#8243);
#5375=LINE('',#37049,#8244);
#5376=LINE('',#37051,#8245);
#5377=LINE('',#37053,#8246);
#5378=LINE('',#37055,#8247);
#5379=LINE('',#37057,#8248);
#5380=LINE('',#37058,#8249);
#5381=LINE('',#37060,#8250);
#5382=LINE('',#37062,#8251);
#5383=LINE('',#37064,#8252);
#5384=LINE('',#37066,#8253);
#5385=LINE('',#37068,#8254);
#5386=LINE('',#37070,#8255);
#5387=LINE('',#37072,#8256);
#5388=LINE('',#37074,#8257);
#5389=LINE('',#37076,#8258);
#5390=LINE('',#37078,#8259);
#5391=LINE('',#37080,#8260);
#5392=LINE('',#37082,#8261);
#5393=LINE('',#37084,#8262);
#5394=LINE('',#37086,#8263);
#5395=LINE('',#37088,#8264);
#5396=LINE('',#37090,#8265);
#5397=LINE('',#37092,#8266);
#5398=LINE('',#37094,#8267);
#5399=LINE('',#37095,#8268);
#5400=LINE('',#37097,#8269);
#5401=LINE('',#37099,#8270);
#5402=LINE('',#37101,#8271);
#5403=LINE('',#37103,#8272);
#5404=LINE('',#37105,#8273);
#5405=LINE('',#37107,#8274);
#5406=LINE('',#37109,#8275);
#5407=LINE('',#37111,#8276);
#5408=LINE('',#37113,#8277);
#5409=LINE('',#37115,#8278);
#5410=LINE('',#37117,#8279);
#5411=LINE('',#37119,#8280);
#5412=LINE('',#37121,#8281);
#5413=LINE('',#37123,#8282);
#5414=LINE('',#37125,#8283);
#5415=LINE('',#37127,#8284);
#5416=LINE('',#37129,#8285);
#5417=LINE('',#37131,#8286);
#5418=LINE('',#37132,#8287);
#5419=LINE('',#37134,#8288);
#5420=LINE('',#37136,#8289);
#5421=LINE('',#37138,#8290);
#5422=LINE('',#37140,#8291);
#5423=LINE('',#37142,#8292);
#5424=LINE('',#37144,#8293);
#5425=LINE('',#37146,#8294);
#5426=LINE('',#37148,#8295);
#5427=LINE('',#37150,#8296);
#5428=LINE('',#37152,#8297);
#5429=LINE('',#37154,#8298);
#5430=LINE('',#37156,#8299);
#5431=LINE('',#37158,#8300);
#5432=LINE('',#37160,#8301);
#5433=LINE('',#37162,#8302);
#5434=LINE('',#37164,#8303);
#5435=LINE('',#37166,#8304);
#5436=LINE('',#37168,#8305);
#5437=LINE('',#37169,#8306);
#5438=LINE('',#37171,#8307);
#5439=LINE('',#37173,#8308);
#5440=LINE('',#37175,#8309);
#5441=LINE('',#37177,#8310);
#5442=LINE('',#37179,#8311);
#5443=LINE('',#37181,#8312);
#5444=LINE('',#37183,#8313);
#5445=LINE('',#37185,#8314);
#5446=LINE('',#37187,#8315);
#5447=LINE('',#37189,#8316);
#5448=LINE('',#37191,#8317);
#5449=LINE('',#37193,#8318);
#5450=LINE('',#37195,#8319);
#5451=LINE('',#37197,#8320);
#5452=LINE('',#37199,#8321);
#5453=LINE('',#37201,#8322);
#5454=LINE('',#37203,#8323);
#5455=LINE('',#37205,#8324);
#5456=LINE('',#37206,#8325);
#5457=LINE('',#37208,#8326);
#5458=LINE('',#37210,#8327);
#5459=LINE('',#37212,#8328);
#5460=LINE('',#37214,#8329);
#5461=LINE('',#37216,#8330);
#5462=LINE('',#37218,#8331);
#5463=LINE('',#37220,#8332);
#5464=LINE('',#37222,#8333);
#5465=LINE('',#37224,#8334);
#5466=LINE('',#37226,#8335);
#5467=LINE('',#37228,#8336);
#5468=LINE('',#37230,#8337);
#5469=LINE('',#37232,#8338);
#5470=LINE('',#37234,#8339);
#5471=LINE('',#37236,#8340);
#5472=LINE('',#37238,#8341);
#5473=LINE('',#37240,#8342);
#5474=LINE('',#37242,#8343);
#5475=LINE('',#37243,#8344);
#5476=LINE('',#37245,#8345);
#5477=LINE('',#37247,#8346);
#5478=LINE('',#37249,#8347);
#5479=LINE('',#37251,#8348);
#5480=LINE('',#37253,#8349);
#5481=LINE('',#37255,#8350);
#5482=LINE('',#37257,#8351);
#5483=LINE('',#37259,#8352);
#5484=LINE('',#37261,#8353);
#5485=LINE('',#37263,#8354);
#5486=LINE('',#37265,#8355);
#5487=LINE('',#37267,#8356);
#5488=LINE('',#37269,#8357);
#5489=LINE('',#37271,#8358);
#5490=LINE('',#37273,#8359);
#5491=LINE('',#37275,#8360);
#5492=LINE('',#37277,#8361);
#5493=LINE('',#37279,#8362);
#5494=LINE('',#37280,#8363);
#5495=LINE('',#37282,#8364);
#5496=LINE('',#37284,#8365);
#5497=LINE('',#37286,#8366);
#5498=LINE('',#37288,#8367);
#5499=LINE('',#37290,#8368);
#5500=LINE('',#37292,#8369);
#5501=LINE('',#37294,#8370);
#5502=LINE('',#37296,#8371);
#5503=LINE('',#37298,#8372);
#5504=LINE('',#37300,#8373);
#5505=LINE('',#37302,#8374);
#5506=LINE('',#37304,#8375);
#5507=LINE('',#37306,#8376);
#5508=LINE('',#37308,#8377);
#5509=LINE('',#37310,#8378);
#5510=LINE('',#37312,#8379);
#5511=LINE('',#37314,#8380);
#5512=LINE('',#37316,#8381);
#5513=LINE('',#37317,#8382);
#5514=LINE('',#37319,#8383);
#5515=LINE('',#37321,#8384);
#5516=LINE('',#37323,#8385);
#5517=LINE('',#37325,#8386);
#5518=LINE('',#37327,#8387);
#5519=LINE('',#37329,#8388);
#5520=LINE('',#37331,#8389);
#5521=LINE('',#37333,#8390);
#5522=LINE('',#37335,#8391);
#5523=LINE('',#37337,#8392);
#5524=LINE('',#37339,#8393);
#5525=LINE('',#37341,#8394);
#5526=LINE('',#37343,#8395);
#5527=LINE('',#37345,#8396);
#5528=LINE('',#37347,#8397);
#5529=LINE('',#37349,#8398);
#5530=LINE('',#37351,#8399);
#5531=LINE('',#37353,#8400);
#5532=LINE('',#37354,#8401);
#5533=LINE('',#37356,#8402);
#5534=LINE('',#37358,#8403);
#5535=LINE('',#37360,#8404);
#5536=LINE('',#37362,#8405);
#5537=LINE('',#37364,#8406);
#5538=LINE('',#37366,#8407);
#5539=LINE('',#37368,#8408);
#5540=LINE('',#37370,#8409);
#5541=LINE('',#37372,#8410);
#5542=LINE('',#37374,#8411);
#5543=LINE('',#37376,#8412);
#5544=LINE('',#37378,#8413);
#5545=LINE('',#37380,#8414);
#5546=LINE('',#37382,#8415);
#5547=LINE('',#37384,#8416);
#5548=LINE('',#37386,#8417);
#5549=LINE('',#37388,#8418);
#5550=LINE('',#37390,#8419);
#5551=LINE('',#37391,#8420);
#5552=LINE('',#37393,#8421);
#5553=LINE('',#37395,#8422);
#5554=LINE('',#37397,#8423);
#5555=LINE('',#37399,#8424);
#5556=LINE('',#37401,#8425);
#5557=LINE('',#37403,#8426);
#5558=LINE('',#37405,#8427);
#5559=LINE('',#37407,#8428);
#5560=LINE('',#37409,#8429);
#5561=LINE('',#37411,#8430);
#5562=LINE('',#37413,#8431);
#5563=LINE('',#37415,#8432);
#5564=LINE('',#37417,#8433);
#5565=LINE('',#37419,#8434);
#5566=LINE('',#37421,#8435);
#5567=LINE('',#37423,#8436);
#5568=LINE('',#37425,#8437);
#5569=LINE('',#37427,#8438);
#5570=LINE('',#37428,#8439);
#5571=LINE('',#37430,#8440);
#5572=LINE('',#37432,#8441);
#5573=LINE('',#37434,#8442);
#5574=LINE('',#37436,#8443);
#5575=LINE('',#37438,#8444);
#5576=LINE('',#37440,#8445);
#5577=LINE('',#37442,#8446);
#5578=LINE('',#37444,#8447);
#5579=LINE('',#37446,#8448);
#5580=LINE('',#37448,#8449);
#5581=LINE('',#37450,#8450);
#5582=LINE('',#37452,#8451);
#5583=LINE('',#37454,#8452);
#5584=LINE('',#37456,#8453);
#5585=LINE('',#37458,#8454);
#5586=LINE('',#37460,#8455);
#5587=LINE('',#37462,#8456);
#5588=LINE('',#37464,#8457);
#5589=LINE('',#37465,#8458);
#5590=LINE('',#37470,#8459);
#5591=LINE('',#37471,#8460);
#5592=LINE('',#37472,#8461);
#5593=LINE('',#37475,#8462);
#5594=LINE('',#37477,#8463);
#5595=LINE('',#37478,#8464);
#5596=LINE('',#37481,#8465);
#5597=LINE('',#37482,#8466);
#5598=LINE('',#37483,#8467);
#5599=LINE('',#37486,#8468);
#5600=LINE('',#37488,#8469);
#5601=LINE('',#37489,#8470);
#5602=LINE('',#37492,#8471);
#5603=LINE('',#37493,#8472);
#5604=LINE('',#37494,#8473);
#5605=LINE('',#37497,#8474);
#5606=LINE('',#37499,#8475);
#5607=LINE('',#37500,#8476);
#5608=LINE('',#37503,#8477);
#5609=LINE('',#37504,#8478);
#5610=LINE('',#37505,#8479);
#5611=LINE('',#37508,#8480);
#5612=LINE('',#37510,#8481);
#5613=LINE('',#37511,#8482);
#5614=LINE('',#37514,#8483);
#5615=LINE('',#37515,#8484);
#5616=LINE('',#37516,#8485);
#5617=LINE('',#37519,#8486);
#5618=LINE('',#37521,#8487);
#5619=LINE('',#37522,#8488);
#5620=LINE('',#37525,#8489);
#5621=LINE('',#37526,#8490);
#5622=LINE('',#37527,#8491);
#5623=LINE('',#37530,#8492);
#5624=LINE('',#37532,#8493);
#5625=LINE('',#37533,#8494);
#5626=LINE('',#37536,#8495);
#5627=LINE('',#37537,#8496);
#5628=LINE('',#37538,#8497);
#5629=LINE('',#37541,#8498);
#5630=LINE('',#37543,#8499);
#5631=LINE('',#37544,#8500);
#5632=LINE('',#37547,#8501);
#5633=LINE('',#37548,#8502);
#5634=LINE('',#37549,#8503);
#5635=LINE('',#37552,#8504);
#5636=LINE('',#37554,#8505);
#5637=LINE('',#37555,#8506);
#5638=LINE('',#37558,#8507);
#5639=LINE('',#37559,#8508);
#5640=LINE('',#37560,#8509);
#5641=LINE('',#37563,#8510);
#5642=LINE('',#37565,#8511);
#5643=LINE('',#37566,#8512);
#5644=LINE('',#37569,#8513);
#5645=LINE('',#37570,#8514);
#5646=LINE('',#37571,#8515);
#5647=LINE('',#37574,#8516);
#5648=LINE('',#37576,#8517);
#5649=LINE('',#37577,#8518);
#5650=LINE('',#37580,#8519);
#5651=LINE('',#37581,#8520);
#5652=LINE('',#37582,#8521);
#5653=LINE('',#37585,#8522);
#5654=LINE('',#37587,#8523);
#5655=LINE('',#37588,#8524);
#5656=LINE('',#37591,#8525);
#5657=LINE('',#37592,#8526);
#5658=LINE('',#37593,#8527);
#5659=LINE('',#37599,#8528);
#5660=LINE('',#37601,#8529);
#5661=LINE('',#37602,#8530);
#5662=LINE('',#37605,#8531);
#5663=LINE('',#37607,#8532);
#5664=LINE('',#37608,#8533);
#5665=LINE('',#37611,#8534);
#5666=LINE('',#37613,#8535);
#5667=LINE('',#37614,#8536);
#5668=LINE('',#37617,#8537);
#5669=LINE('',#37620,#8538);
#5670=LINE('',#37621,#8539);
#5671=LINE('',#37623,#8540);
#5672=LINE('',#37626,#8541);
#5673=LINE('',#37628,#8542);
#5674=LINE('',#37630,#8543);
#5675=LINE('',#37632,#8544);
#5676=LINE('',#37634,#8545);
#5677=LINE('',#37636,#8546);
#5678=LINE('',#37638,#8547);
#5679=LINE('',#37640,#8548);
#5680=LINE('',#37642,#8549);
#5681=LINE('',#37644,#8550);
#5682=LINE('',#37646,#8551);
#5683=LINE('',#37648,#8552);
#5684=LINE('',#37650,#8553);
#5685=LINE('',#37652,#8554);
#5686=LINE('',#37654,#8555);
#5687=LINE('',#37657,#8556);
#5688=LINE('',#37659,#8557);
#5689=LINE('',#37661,#8558);
#5690=LINE('',#37664,#8559);
#5691=LINE('',#37666,#8560);
#5692=LINE('',#37668,#8561);
#5693=LINE('',#37670,#8562);
#5694=LINE('',#37672,#8563);
#5695=LINE('',#37674,#8564);
#5696=LINE('',#37676,#8565);
#5697=LINE('',#37678,#8566);
#5698=LINE('',#37680,#8567);
#5699=LINE('',#37682,#8568);
#5700=LINE('',#37684,#8569);
#5701=LINE('',#37686,#8570);
#5702=LINE('',#37688,#8571);
#5703=LINE('',#37690,#8572);
#5704=LINE('',#37692,#8573);
#5705=LINE('',#37695,#8574);
#5706=LINE('',#37697,#8575);
#5707=LINE('',#37699,#8576);
#5708=LINE('',#37702,#8577);
#5709=LINE('',#37704,#8578);
#5710=LINE('',#37706,#8579);
#5711=LINE('',#37708,#8580);
#5712=LINE('',#37710,#8581);
#5713=LINE('',#37712,#8582);
#5714=LINE('',#37714,#8583);
#5715=LINE('',#37716,#8584);
#5716=LINE('',#37718,#8585);
#5717=LINE('',#37720,#8586);
#5718=LINE('',#37722,#8587);
#5719=LINE('',#37724,#8588);
#5720=LINE('',#37726,#8589);
#5721=LINE('',#37728,#8590);
#5722=LINE('',#37730,#8591);
#5723=LINE('',#37733,#8592);
#5724=LINE('',#37735,#8593);
#5725=LINE('',#37737,#8594);
#5726=LINE('',#37740,#8595);
#5727=LINE('',#37742,#8596);
#5728=LINE('',#37744,#8597);
#5729=LINE('',#37746,#8598);
#5730=LINE('',#37748,#8599);
#5731=LINE('',#37750,#8600);
#5732=LINE('',#37752,#8601);
#5733=LINE('',#37754,#8602);
#5734=LINE('',#37756,#8603);
#5735=LINE('',#37758,#8604);
#5736=LINE('',#37760,#8605);
#5737=LINE('',#37762,#8606);
#5738=LINE('',#37764,#8607);
#5739=LINE('',#37766,#8608);
#5740=LINE('',#37768,#8609);
#5741=LINE('',#37771,#8610);
#5742=LINE('',#37773,#8611);
#5743=LINE('',#37775,#8612);
#5744=LINE('',#37778,#8613);
#5745=LINE('',#37780,#8614);
#5746=LINE('',#37782,#8615);
#5747=LINE('',#37784,#8616);
#5748=LINE('',#37786,#8617);
#5749=LINE('',#37788,#8618);
#5750=LINE('',#37790,#8619);
#5751=LINE('',#37792,#8620);
#5752=LINE('',#37794,#8621);
#5753=LINE('',#37796,#8622);
#5754=LINE('',#37798,#8623);
#5755=LINE('',#37800,#8624);
#5756=LINE('',#37802,#8625);
#5757=LINE('',#37804,#8626);
#5758=LINE('',#37806,#8627);
#5759=LINE('',#37809,#8628);
#5760=LINE('',#37811,#8629);
#5761=LINE('',#37813,#8630);
#5762=LINE('',#37816,#8631);
#5763=LINE('',#37818,#8632);
#5764=LINE('',#37820,#8633);
#5765=LINE('',#37822,#8634);
#5766=LINE('',#37824,#8635);
#5767=LINE('',#37826,#8636);
#5768=LINE('',#37828,#8637);
#5769=LINE('',#37830,#8638);
#5770=LINE('',#37832,#8639);
#5771=LINE('',#37834,#8640);
#5772=LINE('',#37836,#8641);
#5773=LINE('',#37838,#8642);
#5774=LINE('',#37840,#8643);
#5775=LINE('',#37842,#8644);
#5776=LINE('',#37844,#8645);
#5777=LINE('',#37847,#8646);
#5778=LINE('',#37849,#8647);
#5779=LINE('',#37851,#8648);
#5780=LINE('',#37854,#8649);
#5781=LINE('',#37856,#8650);
#5782=LINE('',#37858,#8651);
#5783=LINE('',#37860,#8652);
#5784=LINE('',#37862,#8653);
#5785=LINE('',#37864,#8654);
#5786=LINE('',#37866,#8655);
#5787=LINE('',#37868,#8656);
#5788=LINE('',#37870,#8657);
#5789=LINE('',#37872,#8658);
#5790=LINE('',#37874,#8659);
#5791=LINE('',#37876,#8660);
#5792=LINE('',#37878,#8661);
#5793=LINE('',#37880,#8662);
#5794=LINE('',#37882,#8663);
#5795=LINE('',#37885,#8664);
#5796=LINE('',#37887,#8665);
#5797=LINE('',#37889,#8666);
#5798=LINE('',#37892,#8667);
#5799=LINE('',#37894,#8668);
#5800=LINE('',#37896,#8669);
#5801=LINE('',#37898,#8670);
#5802=LINE('',#37900,#8671);
#5803=LINE('',#37902,#8672);
#5804=LINE('',#37904,#8673);
#5805=LINE('',#37906,#8674);
#5806=LINE('',#37908,#8675);
#5807=LINE('',#37910,#8676);
#5808=LINE('',#37912,#8677);
#5809=LINE('',#37914,#8678);
#5810=LINE('',#37916,#8679);
#5811=LINE('',#37918,#8680);
#5812=LINE('',#37920,#8681);
#5813=LINE('',#37923,#8682);
#5814=LINE('',#37925,#8683);
#5815=LINE('',#37927,#8684);
#5816=LINE('',#37930,#8685);
#5817=LINE('',#37932,#8686);
#5818=LINE('',#37934,#8687);
#5819=LINE('',#37936,#8688);
#5820=LINE('',#37938,#8689);
#5821=LINE('',#37940,#8690);
#5822=LINE('',#37942,#8691);
#5823=LINE('',#37944,#8692);
#5824=LINE('',#37946,#8693);
#5825=LINE('',#37948,#8694);
#5826=LINE('',#37950,#8695);
#5827=LINE('',#37952,#8696);
#5828=LINE('',#37954,#8697);
#5829=LINE('',#37956,#8698);
#5830=LINE('',#37958,#8699);
#5831=LINE('',#37961,#8700);
#5832=LINE('',#37963,#8701);
#5833=LINE('',#37965,#8702);
#5834=LINE('',#37968,#8703);
#5835=LINE('',#37970,#8704);
#5836=LINE('',#37972,#8705);
#5837=LINE('',#37974,#8706);
#5838=LINE('',#37976,#8707);
#5839=LINE('',#37978,#8708);
#5840=LINE('',#37980,#8709);
#5841=LINE('',#37982,#8710);
#5842=LINE('',#37984,#8711);
#5843=LINE('',#37986,#8712);
#5844=LINE('',#37988,#8713);
#5845=LINE('',#37990,#8714);
#5846=LINE('',#37992,#8715);
#5847=LINE('',#37994,#8716);
#5848=LINE('',#37996,#8717);
#5849=LINE('',#37999,#8718);
#5850=LINE('',#38001,#8719);
#5851=LINE('',#38003,#8720);
#5852=LINE('',#38006,#8721);
#5853=LINE('',#38008,#8722);
#5854=LINE('',#38010,#8723);
#5855=LINE('',#38012,#8724);
#5856=LINE('',#38014,#8725);
#5857=LINE('',#38016,#8726);
#5858=LINE('',#38018,#8727);
#5859=LINE('',#38020,#8728);
#5860=LINE('',#38022,#8729);
#5861=LINE('',#38024,#8730);
#5862=LINE('',#38026,#8731);
#5863=LINE('',#38028,#8732);
#5864=LINE('',#38030,#8733);
#5865=LINE('',#38032,#8734);
#5866=LINE('',#38034,#8735);
#5867=LINE('',#38037,#8736);
#5868=LINE('',#38039,#8737);
#5869=LINE('',#38041,#8738);
#5870=LINE('',#38044,#8739);
#5871=LINE('',#38046,#8740);
#5872=LINE('',#38048,#8741);
#5873=LINE('',#38050,#8742);
#5874=LINE('',#38052,#8743);
#5875=LINE('',#38054,#8744);
#5876=LINE('',#38056,#8745);
#5877=LINE('',#38058,#8746);
#5878=LINE('',#38060,#8747);
#5879=LINE('',#38062,#8748);
#5880=LINE('',#38064,#8749);
#5881=LINE('',#38066,#8750);
#5882=LINE('',#38068,#8751);
#5883=LINE('',#38070,#8752);
#5884=LINE('',#38072,#8753);
#5885=LINE('',#38077,#8754);
#5886=LINE('',#38085,#8755);
#5887=LINE('',#38089,#8756);
#5888=LINE('',#38094,#8757);
#7736=VECTOR('',#28464,10.);
#7737=VECTOR('',#28465,10.);
#7738=VECTOR('',#28466,10.);
#7739=VECTOR('',#28467,10.);
#7740=VECTOR('',#28468,10.);
#7741=VECTOR('',#28469,10.);
#7742=VECTOR('',#28472,10.);
#7743=VECTOR('',#28473,10.);
#7744=VECTOR('',#28474,10.);
#7745=VECTOR('',#28475,10.);
#7746=VECTOR('',#28476,10.);
#7747=VECTOR('',#28477,10.);
#7748=VECTOR('',#28478,10.);
#7749=VECTOR('',#28479,10.);
#7750=VECTOR('',#28480,10.);
#7751=VECTOR('',#28481,10.);
#7752=VECTOR('',#28482,10.);
#7753=VECTOR('',#28483,10.);
#7754=VECTOR('',#28484,10.);
#7755=VECTOR('',#28485,10.);
#7756=VECTOR('',#28486,10.);
#7757=VECTOR('',#28487,10.);
#7758=VECTOR('',#28488,10.);
#7759=VECTOR('',#28489,10.);
#7760=VECTOR('',#28490,10.);
#7761=VECTOR('',#28491,10.);
#7762=VECTOR('',#28492,10.);
#7763=VECTOR('',#28493,10.);
#7764=VECTOR('',#28494,10.);
#7765=VECTOR('',#28495,10.);
#7766=VECTOR('',#28496,10.);
#7767=VECTOR('',#28497,10.);
#7768=VECTOR('',#28498,10.);
#7769=VECTOR('',#28499,10.);
#7770=VECTOR('',#28500,10.);
#7771=VECTOR('',#28501,10.);
#7772=VECTOR('',#28502,10.);
#7773=VECTOR('',#28503,10.);
#7774=VECTOR('',#28504,10.);
#7775=VECTOR('',#28505,10.);
#7776=VECTOR('',#28506,10.);
#7777=VECTOR('',#28507,10.);
#7778=VECTOR('',#28508,10.);
#7779=VECTOR('',#28509,10.);
#7780=VECTOR('',#28510,10.);
#7781=VECTOR('',#28511,10.);
#7782=VECTOR('',#28512,10.);
#7783=VECTOR('',#28513,10.);
#7784=VECTOR('',#28514,10.);
#7785=VECTOR('',#28515,10.);
#7786=VECTOR('',#28516,10.);
#7787=VECTOR('',#28517,10.);
#7788=VECTOR('',#28518,10.);
#7789=VECTOR('',#28519,10.);
#7790=VECTOR('',#28520,10.);
#7791=VECTOR('',#28521,10.);
#7792=VECTOR('',#28522,10.);
#7793=VECTOR('',#28523,10.);
#7794=VECTOR('',#28524,10.);
#7795=VECTOR('',#28525,10.);
#7796=VECTOR('',#28526,10.);
#7797=VECTOR('',#28527,10.);
#7798=VECTOR('',#28528,10.);
#7799=VECTOR('',#28529,10.);
#7800=VECTOR('',#28530,10.);
#7801=VECTOR('',#28531,10.);
#7802=VECTOR('',#28532,10.);
#7803=VECTOR('',#28533,10.);
#7804=VECTOR('',#28534,10.);
#7805=VECTOR('',#28535,10.);
#7806=VECTOR('',#28536,10.);
#7807=VECTOR('',#28537,10.);
#7808=VECTOR('',#28538,10.);
#7809=VECTOR('',#28539,10.);
#7810=VECTOR('',#28540,10.);
#7811=VECTOR('',#28541,10.);
#7812=VECTOR('',#28542,10.);
#7813=VECTOR('',#28543,10.);
#7814=VECTOR('',#28544,10.);
#7815=VECTOR('',#28545,10.);
#7816=VECTOR('',#28546,10.);
#7817=VECTOR('',#28547,10.);
#7818=VECTOR('',#28548,10.);
#7819=VECTOR('',#28549,10.);
#7820=VECTOR('',#28550,10.);
#7821=VECTOR('',#28551,10.);
#7822=VECTOR('',#28552,10.);
#7823=VECTOR('',#28553,10.);
#7824=VECTOR('',#28554,10.);
#7825=VECTOR('',#28555,10.);
#7826=VECTOR('',#28556,10.);
#7827=VECTOR('',#28557,10.);
#7828=VECTOR('',#28558,10.);
#7829=VECTOR('',#28559,10.);
#7830=VECTOR('',#28560,10.);
#7831=VECTOR('',#28561,10.);
#7832=VECTOR('',#28562,10.);
#7833=VECTOR('',#28563,10.);
#7834=VECTOR('',#28564,10.);
#7835=VECTOR('',#28565,10.);
#7836=VECTOR('',#28566,10.);
#7837=VECTOR('',#28567,10.);
#7838=VECTOR('',#28568,10.);
#7839=VECTOR('',#28569,10.);
#7840=VECTOR('',#28570,10.);
#7841=VECTOR('',#28571,10.);
#7842=VECTOR('',#28572,10.);
#7843=VECTOR('',#28573,10.);
#7844=VECTOR('',#28574,10.);
#7845=VECTOR('',#28575,10.);
#7846=VECTOR('',#28576,10.);
#7847=VECTOR('',#28577,10.);
#7848=VECTOR('',#28578,10.);
#7849=VECTOR('',#28579,10.);
#7850=VECTOR('',#28580,10.);
#7851=VECTOR('',#28581,10.);
#7852=VECTOR('',#28582,10.);
#7853=VECTOR('',#28583,10.);
#7854=VECTOR('',#28584,10.);
#7855=VECTOR('',#28585,10.);
#7856=VECTOR('',#28586,10.);
#7857=VECTOR('',#28587,10.);
#7858=VECTOR('',#28588,10.);
#7859=VECTOR('',#28589,10.);
#7860=VECTOR('',#28590,10.);
#7861=VECTOR('',#28591,10.);
#7862=VECTOR('',#28592,10.);
#7863=VECTOR('',#28593,10.);
#7864=VECTOR('',#28594,10.);
#7865=VECTOR('',#28595,10.);
#7866=VECTOR('',#28596,10.);
#7867=VECTOR('',#28597,10.);
#7868=VECTOR('',#28598,10.);
#7869=VECTOR('',#28599,10.);
#7870=VECTOR('',#28600,10.);
#7871=VECTOR('',#28601,10.);
#7872=VECTOR('',#28602,10.);
#7873=VECTOR('',#28603,10.);
#7874=VECTOR('',#28604,10.);
#7875=VECTOR('',#28605,10.);
#7876=VECTOR('',#28606,10.);
#7877=VECTOR('',#28607,10.);
#7878=VECTOR('',#28608,10.);
#7879=VECTOR('',#28609,10.);
#7880=VECTOR('',#28610,10.);
#7881=VECTOR('',#28611,10.);
#7882=VECTOR('',#28612,10.);
#7883=VECTOR('',#28613,10.);
#7884=VECTOR('',#28614,10.);
#7885=VECTOR('',#28615,10.);
#7886=VECTOR('',#28616,10.);
#7887=VECTOR('',#28617,10.);
#7888=VECTOR('',#28618,10.);
#7889=VECTOR('',#28619,10.);
#7890=VECTOR('',#28620,10.);
#7891=VECTOR('',#28621,10.);
#7892=VECTOR('',#28622,10.);
#7893=VECTOR('',#28623,10.);
#7894=VECTOR('',#28624,10.);
#7895=VECTOR('',#28625,10.);
#7896=VECTOR('',#28626,10.);
#7897=VECTOR('',#28627,10.);
#7898=VECTOR('',#28628,10.);
#7899=VECTOR('',#28629,10.);
#7900=VECTOR('',#28630,10.);
#7901=VECTOR('',#28631,10.);
#7902=VECTOR('',#28632,10.);
#7903=VECTOR('',#28633,10.);
#7904=VECTOR('',#28634,10.);
#7905=VECTOR('',#28635,10.);
#7906=VECTOR('',#28636,10.);
#7907=VECTOR('',#28637,10.);
#7908=VECTOR('',#28638,10.);
#7909=VECTOR('',#28639,10.);
#7910=VECTOR('',#28640,10.);
#7911=VECTOR('',#28641,10.);
#7912=VECTOR('',#28642,10.);
#7913=VECTOR('',#28643,10.);
#7914=VECTOR('',#28644,10.);
#7915=VECTOR('',#28645,10.);
#7916=VECTOR('',#28646,10.);
#7917=VECTOR('',#28647,10.);
#7918=VECTOR('',#28648,10.);
#7919=VECTOR('',#28649,10.);
#7920=VECTOR('',#28650,10.);
#7921=VECTOR('',#28651,10.);
#7922=VECTOR('',#28652,10.);
#7923=VECTOR('',#28653,10.);
#7924=VECTOR('',#28654,10.);
#7925=VECTOR('',#28655,10.);
#7926=VECTOR('',#28656,10.);
#7927=VECTOR('',#28657,10.);
#7928=VECTOR('',#28658,10.);
#7929=VECTOR('',#28659,10.);
#7930=VECTOR('',#28660,10.);
#7931=VECTOR('',#28661,10.);
#7932=VECTOR('',#28662,10.);
#7933=VECTOR('',#28663,10.);
#7934=VECTOR('',#28664,10.);
#7935=VECTOR('',#28665,10.);
#7936=VECTOR('',#28666,10.);
#7937=VECTOR('',#28667,10.);
#7938=VECTOR('',#28668,10.);
#7939=VECTOR('',#28669,10.);
#7940=VECTOR('',#28670,10.);
#7941=VECTOR('',#28671,10.);
#7942=VECTOR('',#28672,10.);
#7943=VECTOR('',#28673,10.);
#7944=VECTOR('',#28674,10.);
#7945=VECTOR('',#28675,10.);
#7946=VECTOR('',#28676,10.);
#7947=VECTOR('',#28677,10.);
#7948=VECTOR('',#28678,10.);
#7949=VECTOR('',#28679,10.);
#7950=VECTOR('',#28680,10.);
#7951=VECTOR('',#28681,10.);
#7952=VECTOR('',#28682,10.);
#7953=VECTOR('',#28683,10.);
#7954=VECTOR('',#28684,10.);
#7955=VECTOR('',#28685,10.);
#7956=VECTOR('',#28686,10.);
#7957=VECTOR('',#28687,10.);
#7958=VECTOR('',#28688,10.);
#7959=VECTOR('',#28689,10.);
#7960=VECTOR('',#28690,10.);
#7961=VECTOR('',#28691,10.);
#7962=VECTOR('',#28692,10.);
#7963=VECTOR('',#28693,10.);
#7964=VECTOR('',#28694,10.);
#7965=VECTOR('',#28695,10.);
#7966=VECTOR('',#28696,10.);
#7967=VECTOR('',#28697,10.);
#7968=VECTOR('',#28698,10.);
#7969=VECTOR('',#28699,10.);
#7970=VECTOR('',#28700,10.);
#7971=VECTOR('',#28701,10.);
#7972=VECTOR('',#28702,10.);
#7973=VECTOR('',#28703,10.);
#7974=VECTOR('',#28704,10.);
#7975=VECTOR('',#28705,10.);
#7976=VECTOR('',#28706,10.);
#7977=VECTOR('',#28707,10.);
#7978=VECTOR('',#28708,10.);
#7979=VECTOR('',#28709,10.);
#7980=VECTOR('',#28710,10.);
#7981=VECTOR('',#28715,10.);
#7982=VECTOR('',#28716,10.);
#7983=VECTOR('',#28717,10.);
#7984=VECTOR('',#28718,10.);
#7985=VECTOR('',#28721,10.);
#7986=VECTOR('',#28722,10.);
#7987=VECTOR('',#28725,10.);
#7988=VECTOR('',#28726,10.);
#7989=VECTOR('',#28727,10.);
#7990=VECTOR('',#28728,10.);
#7991=VECTOR('',#28729,10.);
#7992=VECTOR('',#28732,10.);
#7993=VECTOR('',#28733,10.);
#7994=VECTOR('',#28734,10.);
#7995=VECTOR('',#28735,10.);
#7996=VECTOR('',#28738,10.);
#7997=VECTOR('',#28739,10.);
#7998=VECTOR('',#28742,10.);
#7999=VECTOR('',#28743,10.);
#8000=VECTOR('',#28744,10.);
#8001=VECTOR('',#28745,10.);
#8002=VECTOR('',#28746,10.);
#8003=VECTOR('',#28749,10.);
#8004=VECTOR('',#28750,10.);
#8005=VECTOR('',#28751,10.);
#8006=VECTOR('',#28752,10.);
#8007=VECTOR('',#28755,10.);
#8008=VECTOR('',#28756,10.);
#8009=VECTOR('',#28759,10.);
#8010=VECTOR('',#28760,10.);
#8011=VECTOR('',#28761,10.);
#8012=VECTOR('',#28762,10.);
#8013=VECTOR('',#28763,10.);
#8014=VECTOR('',#28766,10.);
#8015=VECTOR('',#28767,10.);
#8016=VECTOR('',#28768,10.);
#8017=VECTOR('',#28769,10.);
#8018=VECTOR('',#28772,10.);
#8019=VECTOR('',#28773,10.);
#8020=VECTOR('',#28776,10.);
#8021=VECTOR('',#28777,10.);
#8022=VECTOR('',#28778,10.);
#8023=VECTOR('',#28779,10.);
#8024=VECTOR('',#28780,10.);
#8025=VECTOR('',#28783,10.);
#8026=VECTOR('',#28784,10.);
#8027=VECTOR('',#28785,10.);
#8028=VECTOR('',#28786,10.);
#8029=VECTOR('',#28789,10.);
#8030=VECTOR('',#28790,10.);
#8031=VECTOR('',#28793,10.);
#8032=VECTOR('',#28794,10.);
#8033=VECTOR('',#28795,10.);
#8034=VECTOR('',#28796,10.);
#8035=VECTOR('',#28797,10.);
#8036=VECTOR('',#28800,10.);
#8037=VECTOR('',#28801,10.);
#8038=VECTOR('',#28802,10.);
#8039=VECTOR('',#28803,10.);
#8040=VECTOR('',#28806,10.);
#8041=VECTOR('',#28807,10.);
#8042=VECTOR('',#28810,10.);
#8043=VECTOR('',#28811,10.);
#8044=VECTOR('',#28812,10.);
#8045=VECTOR('',#28813,10.);
#8046=VECTOR('',#28814,10.);
#8047=VECTOR('',#28817,10.);
#8048=VECTOR('',#28818,10.);
#8049=VECTOR('',#28819,10.);
#8050=VECTOR('',#28820,10.);
#8051=VECTOR('',#28823,10.);
#8052=VECTOR('',#28824,10.);
#8053=VECTOR('',#28827,10.);
#8054=VECTOR('',#28828,10.);
#8055=VECTOR('',#28829,10.);
#8056=VECTOR('',#28830,10.);
#8057=VECTOR('',#28831,10.);
#8058=VECTOR('',#28834,10.);
#8059=VECTOR('',#28835,10.);
#8060=VECTOR('',#28836,10.);
#8061=VECTOR('',#28837,10.);
#8062=VECTOR('',#28840,10.);
#8063=VECTOR('',#28841,10.);
#8064=VECTOR('',#28844,10.);
#8065=VECTOR('',#28845,10.);
#8066=VECTOR('',#28846,10.);
#8067=VECTOR('',#28847,10.);
#8068=VECTOR('',#28848,10.);
#8069=VECTOR('',#28851,10.);
#8070=VECTOR('',#28852,10.);
#8071=VECTOR('',#28853,10.);
#8072=VECTOR('',#28854,10.);
#8073=VECTOR('',#28857,10.);
#8074=VECTOR('',#28858,10.);
#8075=VECTOR('',#28861,10.);
#8076=VECTOR('',#28862,10.);
#8077=VECTOR('',#28863,10.);
#8078=VECTOR('',#28864,10.);
#8079=VECTOR('',#28865,10.);
#8080=VECTOR('',#28868,10.);
#8081=VECTOR('',#28869,10.);
#8082=VECTOR('',#28870,10.);
#8083=VECTOR('',#28871,10.);
#8084=VECTOR('',#28874,10.);
#8085=VECTOR('',#28875,10.);
#8086=VECTOR('',#28878,10.);
#8087=VECTOR('',#28879,10.);
#8088=VECTOR('',#28880,10.);
#8089=VECTOR('',#28881,10.);
#8090=VECTOR('',#28882,10.);
#8091=VECTOR('',#28885,10.);
#8092=VECTOR('',#28886,10.);
#8093=VECTOR('',#28887,10.);
#8094=VECTOR('',#28888,10.);
#8095=VECTOR('',#28891,10.);
#8096=VECTOR('',#28892,10.);
#8097=VECTOR('',#28895,10.);
#8098=VECTOR('',#28896,10.);
#8099=VECTOR('',#28897,10.);
#8100=VECTOR('',#28898,10.);
#8101=VECTOR('',#28899,10.);
#8102=VECTOR('',#28902,10.);
#8103=VECTOR('',#28903,10.);
#8104=VECTOR('',#28904,10.);
#8105=VECTOR('',#28905,10.);
#8106=VECTOR('',#28908,10.);
#8107=VECTOR('',#28909,10.);
#8108=VECTOR('',#28912,10.);
#8109=VECTOR('',#28913,10.);
#8110=VECTOR('',#28914,10.);
#8111=VECTOR('',#28915,10.);
#8112=VECTOR('',#28916,10.);
#8113=VECTOR('',#28919,10.);
#8114=VECTOR('',#28920,10.);
#8115=VECTOR('',#28921,10.);
#8116=VECTOR('',#28924,10.);
#8117=VECTOR('',#28925,10.);
#8118=VECTOR('',#28928,10.);
#8119=VECTOR('',#28929,10.);
#8120=VECTOR('',#28930,10.);
#8121=VECTOR('',#28931,10.);
#8122=VECTOR('',#28932,10.);
#8123=VECTOR('',#28935,10.);
#8124=VECTOR('',#28936,10.);
#8125=VECTOR('',#28937,10.);
#8126=VECTOR('',#28940,10.);
#8127=VECTOR('',#28941,10.);
#8128=VECTOR('',#28944,10.);
#8129=VECTOR('',#28945,10.);
#8130=VECTOR('',#28946,10.);
#8131=VECTOR('',#28947,10.);
#8132=VECTOR('',#28948,10.);
#8133=VECTOR('',#28951,10.);
#8134=VECTOR('',#28952,10.);
#8135=VECTOR('',#28953,10.);
#8136=VECTOR('',#28956,10.);
#8137=VECTOR('',#28957,10.);
#8138=VECTOR('',#28960,10.);
#8139=VECTOR('',#28961,10.);
#8140=VECTOR('',#28962,10.);
#8141=VECTOR('',#28963,10.);
#8142=VECTOR('',#28964,10.);
#8143=VECTOR('',#28967,10.);
#8144=VECTOR('',#28968,10.);
#8145=VECTOR('',#28969,10.);
#8146=VECTOR('',#28972,10.);
#8147=VECTOR('',#28973,10.);
#8148=VECTOR('',#28976,10.);
#8149=VECTOR('',#28977,10.);
#8150=VECTOR('',#28978,10.);
#8151=VECTOR('',#28979,10.);
#8152=VECTOR('',#28980,10.);
#8153=VECTOR('',#28983,10.);
#8154=VECTOR('',#28984,10.);
#8155=VECTOR('',#28985,10.);
#8156=VECTOR('',#28988,10.);
#8157=VECTOR('',#28989,10.);
#8158=VECTOR('',#28992,10.);
#8159=VECTOR('',#28993,10.);
#8160=VECTOR('',#28994,10.);
#8161=VECTOR('',#28995,10.);
#8162=VECTOR('',#28996,10.);
#8163=VECTOR('',#28999,10.);
#8164=VECTOR('',#29000,10.);
#8165=VECTOR('',#29001,10.);
#8166=VECTOR('',#29004,10.);
#8167=VECTOR('',#29005,10.);
#8168=VECTOR('',#29008,10.);
#8169=VECTOR('',#29009,10.);
#8170=VECTOR('',#29010,10.);
#8171=VECTOR('',#29011,10.);
#8172=VECTOR('',#29012,10.);
#8173=VECTOR('',#29015,10.);
#8174=VECTOR('',#29016,10.);
#8175=VECTOR('',#29017,10.);
#8176=VECTOR('',#29020,10.);
#8177=VECTOR('',#29021,10.);
#8178=VECTOR('',#29024,10.);
#8179=VECTOR('',#29025,10.);
#8180=VECTOR('',#29026,10.);
#8181=VECTOR('',#29027,10.);
#8182=VECTOR('',#29028,10.);
#8183=VECTOR('',#29031,10.);
#8184=VECTOR('',#29032,10.);
#8185=VECTOR('',#29033,10.);
#8186=VECTOR('',#29036,10.);
#8187=VECTOR('',#29037,10.);
#8188=VECTOR('',#29040,10.);
#8189=VECTOR('',#29041,10.);
#8190=VECTOR('',#29042,10.);
#8191=VECTOR('',#29043,10.);
#8192=VECTOR('',#29044,10.);
#8193=VECTOR('',#29047,10.);
#8194=VECTOR('',#29048,10.);
#8195=VECTOR('',#29049,10.);
#8196=VECTOR('',#29052,10.);
#8197=VECTOR('',#29053,10.);
#8198=VECTOR('',#29056,10.);
#8199=VECTOR('',#29057,10.);
#8200=VECTOR('',#29058,10.);
#8201=VECTOR('',#29059,10.);
#8202=VECTOR('',#29060,10.);
#8203=VECTOR('',#29063,10.);
#8204=VECTOR('',#29064,10.);
#8205=VECTOR('',#29065,10.);
#8206=VECTOR('',#29068,10.);
#8207=VECTOR('',#29069,10.);
#8208=VECTOR('',#29072,10.);
#8209=VECTOR('',#29073,10.);
#8210=VECTOR('',#29074,10.);
#8211=VECTOR('',#29075,10.);
#8212=VECTOR('',#29076,10.);
#8213=VECTOR('',#29079,10.);
#8214=VECTOR('',#29080,10.);
#8215=VECTOR('',#29081,10.);
#8216=VECTOR('',#29084,10.);
#8217=VECTOR('',#29085,10.);
#8218=VECTOR('',#29088,10.);
#8219=VECTOR('',#29089,10.);
#8220=VECTOR('',#29090,10.);
#8221=VECTOR('',#29091,10.);
#8222=VECTOR('',#29092,10.);
#8223=VECTOR('',#29095,10.);
#8224=VECTOR('',#29096,10.);
#8225=VECTOR('',#29097,10.);
#8226=VECTOR('',#29100,10.);
#8227=VECTOR('',#29101,10.);
#8228=VECTOR('',#29104,10.);
#8229=VECTOR('',#29105,10.);
#8230=VECTOR('',#29106,10.);
#8231=VECTOR('',#29107,10.);
#8232=VECTOR('',#29110,10.);
#8233=VECTOR('',#29111,10.);
#8234=VECTOR('',#29112,10.);
#8235=VECTOR('',#29113,10.);
#8236=VECTOR('',#29114,10.);
#8237=VECTOR('',#29115,10.);
#8238=VECTOR('',#29116,10.);
#8239=VECTOR('',#29117,10.);
#8240=VECTOR('',#29118,10.);
#8241=VECTOR('',#29119,10.);
#8242=VECTOR('',#29120,10.);
#8243=VECTOR('',#29121,10.);
#8244=VECTOR('',#29122,10.);
#8245=VECTOR('',#29123,10.);
#8246=VECTOR('',#29124,10.);
#8247=VECTOR('',#29125,10.);
#8248=VECTOR('',#29126,10.);
#8249=VECTOR('',#29127,10.);
#8250=VECTOR('',#29128,10.);
#8251=VECTOR('',#29129,10.);
#8252=VECTOR('',#29130,10.);
#8253=VECTOR('',#29131,10.);
#8254=VECTOR('',#29132,10.);
#8255=VECTOR('',#29133,10.);
#8256=VECTOR('',#29134,10.);
#8257=VECTOR('',#29135,10.);
#8258=VECTOR('',#29136,10.);
#8259=VECTOR('',#29137,10.);
#8260=VECTOR('',#29138,10.);
#8261=VECTOR('',#29139,10.);
#8262=VECTOR('',#29140,10.);
#8263=VECTOR('',#29141,10.);
#8264=VECTOR('',#29142,10.);
#8265=VECTOR('',#29143,10.);
#8266=VECTOR('',#29144,10.);
#8267=VECTOR('',#29145,10.);
#8268=VECTOR('',#29146,10.);
#8269=VECTOR('',#29147,10.);
#8270=VECTOR('',#29148,10.);
#8271=VECTOR('',#29149,10.);
#8272=VECTOR('',#29150,10.);
#8273=VECTOR('',#29151,10.);
#8274=VECTOR('',#29152,10.);
#8275=VECTOR('',#29153,10.);
#8276=VECTOR('',#29154,10.);
#8277=VECTOR('',#29155,10.);
#8278=VECTOR('',#29156,10.);
#8279=VECTOR('',#29157,10.);
#8280=VECTOR('',#29158,10.);
#8281=VECTOR('',#29159,10.);
#8282=VECTOR('',#29160,10.);
#8283=VECTOR('',#29161,10.);
#8284=VECTOR('',#29162,10.);
#8285=VECTOR('',#29163,10.);
#8286=VECTOR('',#29164,10.);
#8287=VECTOR('',#29165,10.);
#8288=VECTOR('',#29166,10.);
#8289=VECTOR('',#29167,10.);
#8290=VECTOR('',#29168,10.);
#8291=VECTOR('',#29169,10.);
#8292=VECTOR('',#29170,10.);
#8293=VECTOR('',#29171,10.);
#8294=VECTOR('',#29172,10.);
#8295=VECTOR('',#29173,10.);
#8296=VECTOR('',#29174,10.);
#8297=VECTOR('',#29175,10.);
#8298=VECTOR('',#29176,10.);
#8299=VECTOR('',#29177,10.);
#8300=VECTOR('',#29178,10.);
#8301=VECTOR('',#29179,10.);
#8302=VECTOR('',#29180,10.);
#8303=VECTOR('',#29181,10.);
#8304=VECTOR('',#29182,10.);
#8305=VECTOR('',#29183,10.);
#8306=VECTOR('',#29184,10.);
#8307=VECTOR('',#29185,10.);
#8308=VECTOR('',#29186,10.);
#8309=VECTOR('',#29187,10.);
#8310=VECTOR('',#29188,10.);
#8311=VECTOR('',#29189,10.);
#8312=VECTOR('',#29190,10.);
#8313=VECTOR('',#29191,10.);
#8314=VECTOR('',#29192,10.);
#8315=VECTOR('',#29193,10.);
#8316=VECTOR('',#29194,10.);
#8317=VECTOR('',#29195,10.);
#8318=VECTOR('',#29196,10.);
#8319=VECTOR('',#29197,10.);
#8320=VECTOR('',#29198,10.);
#8321=VECTOR('',#29199,10.);
#8322=VECTOR('',#29200,10.);
#8323=VECTOR('',#29201,10.);
#8324=VECTOR('',#29202,10.);
#8325=VECTOR('',#29203,10.);
#8326=VECTOR('',#29204,10.);
#8327=VECTOR('',#29205,10.);
#8328=VECTOR('',#29206,10.);
#8329=VECTOR('',#29207,10.);
#8330=VECTOR('',#29208,10.);
#8331=VECTOR('',#29209,10.);
#8332=VECTOR('',#29210,10.);
#8333=VECTOR('',#29211,10.);
#8334=VECTOR('',#29212,10.);
#8335=VECTOR('',#29213,10.);
#8336=VECTOR('',#29214,10.);
#8337=VECTOR('',#29215,10.);
#8338=VECTOR('',#29216,10.);
#8339=VECTOR('',#29217,10.);
#8340=VECTOR('',#29218,10.);
#8341=VECTOR('',#29219,10.);
#8342=VECTOR('',#29220,10.);
#8343=VECTOR('',#29221,10.);
#8344=VECTOR('',#29222,10.);
#8345=VECTOR('',#29223,10.);
#8346=VECTOR('',#29224,10.);
#8347=VECTOR('',#29225,10.);
#8348=VECTOR('',#29226,10.);
#8349=VECTOR('',#29227,10.);
#8350=VECTOR('',#29228,10.);
#8351=VECTOR('',#29229,10.);
#8352=VECTOR('',#29230,10.);
#8353=VECTOR('',#29231,10.);
#8354=VECTOR('',#29232,10.);
#8355=VECTOR('',#29233,10.);
#8356=VECTOR('',#29234,10.);
#8357=VECTOR('',#29235,10.);
#8358=VECTOR('',#29236,10.);
#8359=VECTOR('',#29237,10.);
#8360=VECTOR('',#29238,10.);
#8361=VECTOR('',#29239,10.);
#8362=VECTOR('',#29240,10.);
#8363=VECTOR('',#29241,10.);
#8364=VECTOR('',#29242,10.);
#8365=VECTOR('',#29243,10.);
#8366=VECTOR('',#29244,10.);
#8367=VECTOR('',#29245,10.);
#8368=VECTOR('',#29246,10.);
#8369=VECTOR('',#29247,10.);
#8370=VECTOR('',#29248,10.);
#8371=VECTOR('',#29249,10.);
#8372=VECTOR('',#29250,10.);
#8373=VECTOR('',#29251,10.);
#8374=VECTOR('',#29252,10.);
#8375=VECTOR('',#29253,10.);
#8376=VECTOR('',#29254,10.);
#8377=VECTOR('',#29255,10.);
#8378=VECTOR('',#29256,10.);
#8379=VECTOR('',#29257,10.);
#8380=VECTOR('',#29258,10.);
#8381=VECTOR('',#29259,10.);
#8382=VECTOR('',#29260,10.);
#8383=VECTOR('',#29261,10.);
#8384=VECTOR('',#29262,10.);
#8385=VECTOR('',#29263,10.);
#8386=VECTOR('',#29264,10.);
#8387=VECTOR('',#29265,10.);
#8388=VECTOR('',#29266,10.);
#8389=VECTOR('',#29267,10.);
#8390=VECTOR('',#29268,10.);
#8391=VECTOR('',#29269,10.);
#8392=VECTOR('',#29270,10.);
#8393=VECTOR('',#29271,10.);
#8394=VECTOR('',#29272,10.);
#8395=VECTOR('',#29273,10.);
#8396=VECTOR('',#29274,10.);
#8397=VECTOR('',#29275,10.);
#8398=VECTOR('',#29276,10.);
#8399=VECTOR('',#29277,10.);
#8400=VECTOR('',#29278,10.);
#8401=VECTOR('',#29279,10.);
#8402=VECTOR('',#29280,10.);
#8403=VECTOR('',#29281,10.);
#8404=VECTOR('',#29282,10.);
#8405=VECTOR('',#29283,10.);
#8406=VECTOR('',#29284,10.);
#8407=VECTOR('',#29285,10.);
#8408=VECTOR('',#29286,10.);
#8409=VECTOR('',#29287,10.);
#8410=VECTOR('',#29288,10.);
#8411=VECTOR('',#29289,10.);
#8412=VECTOR('',#29290,10.);
#8413=VECTOR('',#29291,10.);
#8414=VECTOR('',#29292,10.);
#8415=VECTOR('',#29293,10.);
#8416=VECTOR('',#29294,10.);
#8417=VECTOR('',#29295,10.);
#8418=VECTOR('',#29296,10.);
#8419=VECTOR('',#29297,10.);
#8420=VECTOR('',#29298,10.);
#8421=VECTOR('',#29299,10.);
#8422=VECTOR('',#29300,10.);
#8423=VECTOR('',#29301,10.);
#8424=VECTOR('',#29302,10.);
#8425=VECTOR('',#29303,10.);
#8426=VECTOR('',#29304,10.);
#8427=VECTOR('',#29305,10.);
#8428=VECTOR('',#29306,10.);
#8429=VECTOR('',#29307,10.);
#8430=VECTOR('',#29308,10.);
#8431=VECTOR('',#29309,10.);
#8432=VECTOR('',#29310,10.);
#8433=VECTOR('',#29311,10.);
#8434=VECTOR('',#29312,10.);
#8435=VECTOR('',#29313,10.);
#8436=VECTOR('',#29314,10.);
#8437=VECTOR('',#29315,10.);
#8438=VECTOR('',#29316,10.);
#8439=VECTOR('',#29317,10.);
#8440=VECTOR('',#29318,10.);
#8441=VECTOR('',#29319,10.);
#8442=VECTOR('',#29320,10.);
#8443=VECTOR('',#29321,10.);
#8444=VECTOR('',#29322,10.);
#8445=VECTOR('',#29323,10.);
#8446=VECTOR('',#29324,10.);
#8447=VECTOR('',#29325,10.);
#8448=VECTOR('',#29326,10.);
#8449=VECTOR('',#29327,10.);
#8450=VECTOR('',#29328,10.);
#8451=VECTOR('',#29329,10.);
#8452=VECTOR('',#29330,10.);
#8453=VECTOR('',#29331,10.);
#8454=VECTOR('',#29332,10.);
#8455=VECTOR('',#29333,10.);
#8456=VECTOR('',#29334,10.);
#8457=VECTOR('',#29335,10.);
#8458=VECTOR('',#29336,10.);
#8459=VECTOR('',#29341,10.);
#8460=VECTOR('',#29342,10.);
#8461=VECTOR('',#29343,10.);
#8462=VECTOR('',#29346,10.);
#8463=VECTOR('',#29347,10.);
#8464=VECTOR('',#29348,10.);
#8465=VECTOR('',#29351,10.);
#8466=VECTOR('',#29352,10.);
#8467=VECTOR('',#29353,10.);
#8468=VECTOR('',#29356,10.);
#8469=VECTOR('',#29357,10.);
#8470=VECTOR('',#29358,10.);
#8471=VECTOR('',#29361,10.);
#8472=VECTOR('',#29362,10.);
#8473=VECTOR('',#29363,10.);
#8474=VECTOR('',#29366,10.);
#8475=VECTOR('',#29367,10.);
#8476=VECTOR('',#29368,10.);
#8477=VECTOR('',#29371,10.);
#8478=VECTOR('',#29372,10.);
#8479=VECTOR('',#29373,10.);
#8480=VECTOR('',#29376,10.);
#8481=VECTOR('',#29377,10.);
#8482=VECTOR('',#29378,10.);
#8483=VECTOR('',#29381,10.);
#8484=VECTOR('',#29382,10.);
#8485=VECTOR('',#29383,10.);
#8486=VECTOR('',#29386,10.);
#8487=VECTOR('',#29387,10.);
#8488=VECTOR('',#29388,10.);
#8489=VECTOR('',#29391,10.);
#8490=VECTOR('',#29392,10.);
#8491=VECTOR('',#29393,10.);
#8492=VECTOR('',#29396,10.);
#8493=VECTOR('',#29397,10.);
#8494=VECTOR('',#29398,10.);
#8495=VECTOR('',#29401,10.);
#8496=VECTOR('',#29402,10.);
#8497=VECTOR('',#29403,10.);
#8498=VECTOR('',#29406,10.);
#8499=VECTOR('',#29407,10.);
#8500=VECTOR('',#29408,10.);
#8501=VECTOR('',#29411,10.);
#8502=VECTOR('',#29412,10.);
#8503=VECTOR('',#29413,10.);
#8504=VECTOR('',#29416,10.);
#8505=VECTOR('',#29417,10.);
#8506=VECTOR('',#29418,10.);
#8507=VECTOR('',#29421,10.);
#8508=VECTOR('',#29422,10.);
#8509=VECTOR('',#29423,10.);
#8510=VECTOR('',#29426,10.);
#8511=VECTOR('',#29427,10.);
#8512=VECTOR('',#29428,10.);
#8513=VECTOR('',#29431,10.);
#8514=VECTOR('',#29432,10.);
#8515=VECTOR('',#29433,10.);
#8516=VECTOR('',#29436,10.);
#8517=VECTOR('',#29437,10.);
#8518=VECTOR('',#29438,10.);
#8519=VECTOR('',#29441,10.);
#8520=VECTOR('',#29442,10.);
#8521=VECTOR('',#29443,10.);
#8522=VECTOR('',#29446,10.);
#8523=VECTOR('',#29447,10.);
#8524=VECTOR('',#29448,10.);
#8525=VECTOR('',#29451,10.);
#8526=VECTOR('',#29452,10.);
#8527=VECTOR('',#29453,10.);
#8528=VECTOR('',#29458,10.);
#8529=VECTOR('',#29459,10.);
#8530=VECTOR('',#29460,10.);
#8531=VECTOR('',#29463,10.);
#8532=VECTOR('',#29464,10.);
#8533=VECTOR('',#29465,10.);
#8534=VECTOR('',#29468,10.);
#8535=VECTOR('',#29469,10.);
#8536=VECTOR('',#29470,10.);
#8537=VECTOR('',#29475,10.);
#8538=VECTOR('',#29480,10.);
#8539=VECTOR('',#29481,10.);
#8540=VECTOR('',#29484,10.);
#8541=VECTOR('',#29489,10.);
#8542=VECTOR('',#29492,10.);
#8543=VECTOR('',#29495,10.);
#8544=VECTOR('',#29498,10.);
#8545=VECTOR('',#29501,10.);
#8546=VECTOR('',#29504,10.);
#8547=VECTOR('',#29507,10.);
#8548=VECTOR('',#29510,10.);
#8549=VECTOR('',#29513,10.);
#8550=VECTOR('',#29516,10.);
#8551=VECTOR('',#29519,10.);
#8552=VECTOR('',#29522,10.);
#8553=VECTOR('',#29525,10.);
#8554=VECTOR('',#29528,10.);
#8555=VECTOR('',#29531,10.);
#8556=VECTOR('',#29536,10.);
#8557=VECTOR('',#29539,10.);
#8558=VECTOR('',#29542,10.);
#8559=VECTOR('',#29547,10.);
#8560=VECTOR('',#29550,10.);
#8561=VECTOR('',#29553,10.);
#8562=VECTOR('',#29556,10.);
#8563=VECTOR('',#29559,10.);
#8564=VECTOR('',#29562,10.);
#8565=VECTOR('',#29565,10.);
#8566=VECTOR('',#29568,10.);
#8567=VECTOR('',#29571,10.);
#8568=VECTOR('',#29574,10.);
#8569=VECTOR('',#29577,10.);
#8570=VECTOR('',#29580,10.);
#8571=VECTOR('',#29583,10.);
#8572=VECTOR('',#29586,10.);
#8573=VECTOR('',#29589,10.);
#8574=VECTOR('',#29594,10.);
#8575=VECTOR('',#29597,10.);
#8576=VECTOR('',#29600,10.);
#8577=VECTOR('',#29605,10.);
#8578=VECTOR('',#29608,10.);
#8579=VECTOR('',#29611,10.);
#8580=VECTOR('',#29614,10.);
#8581=VECTOR('',#29617,10.);
#8582=VECTOR('',#29620,10.);
#8583=VECTOR('',#29623,10.);
#8584=VECTOR('',#29626,10.);
#8585=VECTOR('',#29629,10.);
#8586=VECTOR('',#29632,10.);
#8587=VECTOR('',#29635,10.);
#8588=VECTOR('',#29638,10.);
#8589=VECTOR('',#29641,10.);
#8590=VECTOR('',#29644,10.);
#8591=VECTOR('',#29647,10.);
#8592=VECTOR('',#29652,10.);
#8593=VECTOR('',#29655,10.);
#8594=VECTOR('',#29658,10.);
#8595=VECTOR('',#29663,10.);
#8596=VECTOR('',#29666,10.);
#8597=VECTOR('',#29669,10.);
#8598=VECTOR('',#29672,10.);
#8599=VECTOR('',#29675,10.);
#8600=VECTOR('',#29678,10.);
#8601=VECTOR('',#29681,10.);
#8602=VECTOR('',#29684,10.);
#8603=VECTOR('',#29687,10.);
#8604=VECTOR('',#29690,10.);
#8605=VECTOR('',#29693,10.);
#8606=VECTOR('',#29696,10.);
#8607=VECTOR('',#29699,10.);
#8608=VECTOR('',#29702,10.);
#8609=VECTOR('',#29705,10.);
#8610=VECTOR('',#29710,10.);
#8611=VECTOR('',#29713,10.);
#8612=VECTOR('',#29716,10.);
#8613=VECTOR('',#29721,10.);
#8614=VECTOR('',#29724,10.);
#8615=VECTOR('',#29727,10.);
#8616=VECTOR('',#29730,10.);
#8617=VECTOR('',#29733,10.);
#8618=VECTOR('',#29736,10.);
#8619=VECTOR('',#29739,10.);
#8620=VECTOR('',#29742,10.);
#8621=VECTOR('',#29745,10.);
#8622=VECTOR('',#29748,10.);
#8623=VECTOR('',#29751,10.);
#8624=VECTOR('',#29754,10.);
#8625=VECTOR('',#29757,10.);
#8626=VECTOR('',#29760,10.);
#8627=VECTOR('',#29763,10.);
#8628=VECTOR('',#29768,10.);
#8629=VECTOR('',#29771,10.);
#8630=VECTOR('',#29774,10.);
#8631=VECTOR('',#29779,10.);
#8632=VECTOR('',#29782,10.);
#8633=VECTOR('',#29785,10.);
#8634=VECTOR('',#29788,10.);
#8635=VECTOR('',#29791,10.);
#8636=VECTOR('',#29794,10.);
#8637=VECTOR('',#29797,10.);
#8638=VECTOR('',#29800,10.);
#8639=VECTOR('',#29803,10.);
#8640=VECTOR('',#29806,10.);
#8641=VECTOR('',#29809,10.);
#8642=VECTOR('',#29812,10.);
#8643=VECTOR('',#29815,10.);
#8644=VECTOR('',#29818,10.);
#8645=VECTOR('',#29821,10.);
#8646=VECTOR('',#29826,10.);
#8647=VECTOR('',#29829,10.);
#8648=VECTOR('',#29832,10.);
#8649=VECTOR('',#29837,10.);
#8650=VECTOR('',#29840,10.);
#8651=VECTOR('',#29843,10.);
#8652=VECTOR('',#29846,10.);
#8653=VECTOR('',#29849,10.);
#8654=VECTOR('',#29852,10.);
#8655=VECTOR('',#29855,10.);
#8656=VECTOR('',#29858,10.);
#8657=VECTOR('',#29861,10.);
#8658=VECTOR('',#29864,10.);
#8659=VECTOR('',#29867,10.);
#8660=VECTOR('',#29870,10.);
#8661=VECTOR('',#29873,10.);
#8662=VECTOR('',#29876,10.);
#8663=VECTOR('',#29879,10.);
#8664=VECTOR('',#29884,10.);
#8665=VECTOR('',#29887,10.);
#8666=VECTOR('',#29890,10.);
#8667=VECTOR('',#29895,10.);
#8668=VECTOR('',#29898,10.);
#8669=VECTOR('',#29901,10.);
#8670=VECTOR('',#29904,10.);
#8671=VECTOR('',#29907,10.);
#8672=VECTOR('',#29910,10.);
#8673=VECTOR('',#29913,10.);
#8674=VECTOR('',#29916,10.);
#8675=VECTOR('',#29919,10.);
#8676=VECTOR('',#29922,10.);
#8677=VECTOR('',#29925,10.);
#8678=VECTOR('',#29928,10.);
#8679=VECTOR('',#29931,10.);
#8680=VECTOR('',#29934,10.);
#8681=VECTOR('',#29937,10.);
#8682=VECTOR('',#29942,10.);
#8683=VECTOR('',#29945,10.);
#8684=VECTOR('',#29948,10.);
#8685=VECTOR('',#29953,10.);
#8686=VECTOR('',#29956,10.);
#8687=VECTOR('',#29959,10.);
#8688=VECTOR('',#29962,10.);
#8689=VECTOR('',#29965,10.);
#8690=VECTOR('',#29968,10.);
#8691=VECTOR('',#29971,10.);
#8692=VECTOR('',#29974,10.);
#8693=VECTOR('',#29977,10.);
#8694=VECTOR('',#29980,10.);
#8695=VECTOR('',#29983,10.);
#8696=VECTOR('',#29986,10.);
#8697=VECTOR('',#29989,10.);
#8698=VECTOR('',#29992,10.);
#8699=VECTOR('',#29995,10.);
#8700=VECTOR('',#30000,10.);
#8701=VECTOR('',#30003,10.);
#8702=VECTOR('',#30006,10.);
#8703=VECTOR('',#30011,10.);
#8704=VECTOR('',#30014,10.);
#8705=VECTOR('',#30017,10.);
#8706=VECTOR('',#30020,10.);
#8707=VECTOR('',#30023,10.);
#8708=VECTOR('',#30026,10.);
#8709=VECTOR('',#30029,10.);
#8710=VECTOR('',#30032,10.);
#8711=VECTOR('',#30035,10.);
#8712=VECTOR('',#30038,10.);
#8713=VECTOR('',#30041,10.);
#8714=VECTOR('',#30044,10.);
#8715=VECTOR('',#30047,10.);
#8716=VECTOR('',#30050,10.);
#8717=VECTOR('',#30053,10.);
#8718=VECTOR('',#30058,10.);
#8719=VECTOR('',#30061,10.);
#8720=VECTOR('',#30064,10.);
#8721=VECTOR('',#30069,10.);
#8722=VECTOR('',#30072,10.);
#8723=VECTOR('',#30075,10.);
#8724=VECTOR('',#30078,10.);
#8725=VECTOR('',#30081,10.);
#8726=VECTOR('',#30084,10.);
#8727=VECTOR('',#30087,10.);
#8728=VECTOR('',#30090,10.);
#8729=VECTOR('',#30093,10.);
#8730=VECTOR('',#30096,10.);
#8731=VECTOR('',#30099,10.);
#8732=VECTOR('',#30102,10.);
#8733=VECTOR('',#30105,10.);
#8734=VECTOR('',#30108,10.);
#8735=VECTOR('',#30111,10.);
#8736=VECTOR('',#30116,10.);
#8737=VECTOR('',#30119,10.);
#8738=VECTOR('',#30122,10.);
#8739=VECTOR('',#30127,10.);
#8740=VECTOR('',#30130,10.);
#8741=VECTOR('',#30133,10.);
#8742=VECTOR('',#30136,10.);
#8743=VECTOR('',#30139,10.);
#8744=VECTOR('',#30142,10.);
#8745=VECTOR('',#30145,10.);
#8746=VECTOR('',#30148,10.);
#8747=VECTOR('',#30151,10.);
#8748=VECTOR('',#30154,10.);
#8749=VECTOR('',#30157,10.);
#8750=VECTOR('',#30160,10.);
#8751=VECTOR('',#30163,10.);
#8752=VECTOR('',#30166,10.);
#8753=VECTOR('',#30169,10.);
#8754=VECTOR('',#30176,8.5);
#8755=VECTOR('',#30187,7.69);
#8756=VECTOR('',#30192,7.94);
#8757=VECTOR('',#30199,8.5);
#10568=CIRCLE('',#25706,8.5);
#10569=CIRCLE('',#25780,8.5);
#10570=CIRCLE('',#25805,7.94);
#10571=CIRCLE('',#25809,7.94);
#10572=CIRCLE('',#26052,8.5);
#10573=CIRCLE('',#26054,7.44);
#10574=CIRCLE('',#26056,7.94);
#10575=CIRCLE('',#26058,7.94);
#10576=CIRCLE('',#26061,8.5);
#11157=VERTEX_POINT('',#36029);
#11158=VERTEX_POINT('',#36030);
#11159=VERTEX_POINT('',#36032);
#11160=VERTEX_POINT('',#36034);
#11161=VERTEX_POINT('',#36036);
#11162=VERTEX_POINT('',#36038);
#11163=VERTEX_POINT('',#36042);
#11164=VERTEX_POINT('',#36044);
#11165=VERTEX_POINT('',#36046);
#11166=VERTEX_POINT('',#36048);
#11167=VERTEX_POINT('',#36050);
#11168=VERTEX_POINT('',#36052);
#11169=VERTEX_POINT('',#36054);
#11170=VERTEX_POINT('',#36056);
#11171=VERTEX_POINT('',#36058);
#11172=VERTEX_POINT('',#36060);
#11173=VERTEX_POINT('',#36062);
#11174=VERTEX_POINT('',#36064);
#11175=VERTEX_POINT('',#36066);
#11176=VERTEX_POINT('',#36068);
#11177=VERTEX_POINT('',#36070);
#11178=VERTEX_POINT('',#36072);
#11179=VERTEX_POINT('',#36074);
#11180=VERTEX_POINT('',#36076);
#11181=VERTEX_POINT('',#36078);
#11182=VERTEX_POINT('',#36080);
#11183=VERTEX_POINT('',#36082);
#11184=VERTEX_POINT('',#36084);
#11185=VERTEX_POINT('',#36086);
#11186=VERTEX_POINT('',#36088);
#11187=VERTEX_POINT('',#36090);
#11188=VERTEX_POINT('',#36092);
#11189=VERTEX_POINT('',#36094);
#11190=VERTEX_POINT('',#36096);
#11191=VERTEX_POINT('',#36098);
#11192=VERTEX_POINT('',#36100);
#11193=VERTEX_POINT('',#36102);
#11194=VERTEX_POINT('',#36104);
#11195=VERTEX_POINT('',#36106);
#11196=VERTEX_POINT('',#36108);
#11197=VERTEX_POINT('',#36110);
#11198=VERTEX_POINT('',#36112);
#11199=VERTEX_POINT('',#36114);
#11200=VERTEX_POINT('',#36116);
#11201=VERTEX_POINT('',#36118);
#11202=VERTEX_POINT('',#36120);
#11203=VERTEX_POINT('',#36122);
#11204=VERTEX_POINT('',#36124);
#11205=VERTEX_POINT('',#36126);
#11206=VERTEX_POINT('',#36128);
#11207=VERTEX_POINT('',#36130);
#11208=VERTEX_POINT('',#36132);
#11209=VERTEX_POINT('',#36134);
#11210=VERTEX_POINT('',#36136);
#11211=VERTEX_POINT('',#36138);
#11212=VERTEX_POINT('',#36140);
#11213=VERTEX_POINT('',#36142);
#11214=VERTEX_POINT('',#36144);
#11215=VERTEX_POINT('',#36146);
#11216=VERTEX_POINT('',#36148);
#11217=VERTEX_POINT('',#36150);
#11218=VERTEX_POINT('',#36152);
#11219=VERTEX_POINT('',#36154);
#11220=VERTEX_POINT('',#36156);
#11221=VERTEX_POINT('',#36158);
#11222=VERTEX_POINT('',#36160);
#11223=VERTEX_POINT('',#36162);
#11224=VERTEX_POINT('',#36164);
#11225=VERTEX_POINT('',#36166);
#11226=VERTEX_POINT('',#36168);
#11227=VERTEX_POINT('',#36170);
#11228=VERTEX_POINT('',#36172);
#11229=VERTEX_POINT('',#36174);
#11230=VERTEX_POINT('',#36176);
#11231=VERTEX_POINT('',#36178);
#11232=VERTEX_POINT('',#36180);
#11233=VERTEX_POINT('',#36182);
#11234=VERTEX_POINT('',#36184);
#11235=VERTEX_POINT('',#36186);
#11236=VERTEX_POINT('',#36188);
#11237=VERTEX_POINT('',#36190);
#11238=VERTEX_POINT('',#36192);
#11239=VERTEX_POINT('',#36194);
#11240=VERTEX_POINT('',#36196);
#11241=VERTEX_POINT('',#36198);
#11242=VERTEX_POINT('',#36200);
#11243=VERTEX_POINT('',#36202);
#11244=VERTEX_POINT('',#36204);
#11245=VERTEX_POINT('',#36206);
#11246=VERTEX_POINT('',#36208);
#11247=VERTEX_POINT('',#36210);
#11248=VERTEX_POINT('',#36212);
#11249=VERTEX_POINT('',#36214);
#11250=VERTEX_POINT('',#36216);
#11251=VERTEX_POINT('',#36218);
#11252=VERTEX_POINT('',#36220);
#11253=VERTEX_POINT('',#36222);
#11254=VERTEX_POINT('',#36224);
#11255=VERTEX_POINT('',#36226);
#11256=VERTEX_POINT('',#36228);
#11257=VERTEX_POINT('',#36230);
#11258=VERTEX_POINT('',#36232);
#11259=VERTEX_POINT('',#36234);
#11260=VERTEX_POINT('',#36236);
#11261=VERTEX_POINT('',#36238);
#11262=VERTEX_POINT('',#36240);
#11263=VERTEX_POINT('',#36242);
#11264=VERTEX_POINT('',#36244);
#11265=VERTEX_POINT('',#36246);
#11266=VERTEX_POINT('',#36248);
#11267=VERTEX_POINT('',#36250);
#11268=VERTEX_POINT('',#36252);
#11269=VERTEX_POINT('',#36254);
#11270=VERTEX_POINT('',#36256);
#11271=VERTEX_POINT('',#36258);
#11272=VERTEX_POINT('',#36260);
#11273=VERTEX_POINT('',#36262);
#11274=VERTEX_POINT('',#36264);
#11275=VERTEX_POINT('',#36266);
#11276=VERTEX_POINT('',#36268);
#11277=VERTEX_POINT('',#36270);
#11278=VERTEX_POINT('',#36272);
#11279=VERTEX_POINT('',#36274);
#11280=VERTEX_POINT('',#36276);
#11281=VERTEX_POINT('',#36278);
#11282=VERTEX_POINT('',#36280);
#11283=VERTEX_POINT('',#36282);
#11284=VERTEX_POINT('',#36284);
#11285=VERTEX_POINT('',#36286);
#11286=VERTEX_POINT('',#36288);
#11287=VERTEX_POINT('',#36290);
#11288=VERTEX_POINT('',#36292);
#11289=VERTEX_POINT('',#36294);
#11290=VERTEX_POINT('',#36296);
#11291=VERTEX_POINT('',#36298);
#11292=VERTEX_POINT('',#36300);
#11293=VERTEX_POINT('',#36302);
#11294=VERTEX_POINT('',#36304);
#11295=VERTEX_POINT('',#36306);
#11296=VERTEX_POINT('',#36308);
#11297=VERTEX_POINT('',#36310);
#11298=VERTEX_POINT('',#36312);
#11299=VERTEX_POINT('',#36314);
#11300=VERTEX_POINT('',#36316);
#11301=VERTEX_POINT('',#36318);
#11302=VERTEX_POINT('',#36320);
#11303=VERTEX_POINT('',#36322);
#11304=VERTEX_POINT('',#36324);
#11305=VERTEX_POINT('',#36326);
#11306=VERTEX_POINT('',#36328);
#11307=VERTEX_POINT('',#36330);
#11308=VERTEX_POINT('',#36332);
#11309=VERTEX_POINT('',#36334);
#11310=VERTEX_POINT('',#36336);
#11311=VERTEX_POINT('',#36338);
#11312=VERTEX_POINT('',#36340);
#11313=VERTEX_POINT('',#36342);
#11314=VERTEX_POINT('',#36344);
#11315=VERTEX_POINT('',#36346);
#11316=VERTEX_POINT('',#36348);
#11317=VERTEX_POINT('',#36350);
#11318=VERTEX_POINT('',#36352);
#11319=VERTEX_POINT('',#36354);
#11320=VERTEX_POINT('',#36356);
#11321=VERTEX_POINT('',#36358);
#11322=VERTEX_POINT('',#36360);
#11323=VERTEX_POINT('',#36362);
#11324=VERTEX_POINT('',#36364);
#11325=VERTEX_POINT('',#36366);
#11326=VERTEX_POINT('',#36368);
#11327=VERTEX_POINT('',#36370);
#11328=VERTEX_POINT('',#36372);
#11329=VERTEX_POINT('',#36374);
#11330=VERTEX_POINT('',#36376);
#11331=VERTEX_POINT('',#36378);
#11332=VERTEX_POINT('',#36380);
#11333=VERTEX_POINT('',#36382);
#11334=VERTEX_POINT('',#36384);
#11335=VERTEX_POINT('',#36386);
#11336=VERTEX_POINT('',#36388);
#11337=VERTEX_POINT('',#36390);
#11338=VERTEX_POINT('',#36392);
#11339=VERTEX_POINT('',#36394);
#11340=VERTEX_POINT('',#36396);
#11341=VERTEX_POINT('',#36398);
#11342=VERTEX_POINT('',#36400);
#11343=VERTEX_POINT('',#36402);
#11344=VERTEX_POINT('',#36404);
#11345=VERTEX_POINT('',#36406);
#11346=VERTEX_POINT('',#36408);
#11347=VERTEX_POINT('',#36410);
#11348=VERTEX_POINT('',#36412);
#11349=VERTEX_POINT('',#36414);
#11350=VERTEX_POINT('',#36416);
#11351=VERTEX_POINT('',#36418);
#11352=VERTEX_POINT('',#36420);
#11353=VERTEX_POINT('',#36422);
#11354=VERTEX_POINT('',#36424);
#11355=VERTEX_POINT('',#36426);
#11356=VERTEX_POINT('',#36428);
#11357=VERTEX_POINT('',#36430);
#11358=VERTEX_POINT('',#36432);
#11359=VERTEX_POINT('',#36434);
#11360=VERTEX_POINT('',#36436);
#11361=VERTEX_POINT('',#36438);
#11362=VERTEX_POINT('',#36440);
#11363=VERTEX_POINT('',#36442);
#11364=VERTEX_POINT('',#36444);
#11365=VERTEX_POINT('',#36446);
#11366=VERTEX_POINT('',#36448);
#11367=VERTEX_POINT('',#36450);
#11368=VERTEX_POINT('',#36452);
#11369=VERTEX_POINT('',#36454);
#11370=VERTEX_POINT('',#36456);
#11371=VERTEX_POINT('',#36458);
#11372=VERTEX_POINT('',#36460);
#11373=VERTEX_POINT('',#36462);
#11374=VERTEX_POINT('',#36464);
#11375=VERTEX_POINT('',#36466);
#11376=VERTEX_POINT('',#36468);
#11377=VERTEX_POINT('',#36470);
#11378=VERTEX_POINT('',#36472);
#11379=VERTEX_POINT('',#36474);
#11380=VERTEX_POINT('',#36476);
#11381=VERTEX_POINT('',#36478);
#11382=VERTEX_POINT('',#36480);
#11383=VERTEX_POINT('',#36482);
#11384=VERTEX_POINT('',#36484);
#11385=VERTEX_POINT('',#36486);
#11386=VERTEX_POINT('',#36488);
#11387=VERTEX_POINT('',#36490);
#11388=VERTEX_POINT('',#36492);
#11389=VERTEX_POINT('',#36494);
#11390=VERTEX_POINT('',#36496);
#11391=VERTEX_POINT('',#36498);
#11392=VERTEX_POINT('',#36500);
#11393=VERTEX_POINT('',#36502);
#11394=VERTEX_POINT('',#36504);
#11395=VERTEX_POINT('',#36506);
#11396=VERTEX_POINT('',#36508);
#11397=VERTEX_POINT('',#36510);
#11398=VERTEX_POINT('',#36512);
#11399=VERTEX_POINT('',#36514);
#11400=VERTEX_POINT('',#36516);
#11401=VERTEX_POINT('',#36519);
#11402=VERTEX_POINT('',#36522);
#11403=VERTEX_POINT('',#36524);
#11404=VERTEX_POINT('',#36526);
#11405=VERTEX_POINT('',#36530);
#11406=VERTEX_POINT('',#36534);
#11407=VERTEX_POINT('',#36536);
#11408=VERTEX_POINT('',#36538);
#11409=VERTEX_POINT('',#36540);
#11410=VERTEX_POINT('',#36544);
#11411=VERTEX_POINT('',#36546);
#11412=VERTEX_POINT('',#36548);
#11413=VERTEX_POINT('',#36552);
#11414=VERTEX_POINT('',#36556);
#11415=VERTEX_POINT('',#36558);
#11416=VERTEX_POINT('',#36560);
#11417=VERTEX_POINT('',#36562);
#11418=VERTEX_POINT('',#36566);
#11419=VERTEX_POINT('',#36568);
#11420=VERTEX_POINT('',#36570);
#11421=VERTEX_POINT('',#36574);
#11422=VERTEX_POINT('',#36578);
#11423=VERTEX_POINT('',#36580);
#11424=VERTEX_POINT('',#36582);
#11425=VERTEX_POINT('',#36584);
#11426=VERTEX_POINT('',#36588);
#11427=VERTEX_POINT('',#36590);
#11428=VERTEX_POINT('',#36592);
#11429=VERTEX_POINT('',#36596);
#11430=VERTEX_POINT('',#36600);
#11431=VERTEX_POINT('',#36602);
#11432=VERTEX_POINT('',#36604);
#11433=VERTEX_POINT('',#36606);
#11434=VERTEX_POINT('',#36610);
#11435=VERTEX_POINT('',#36612);
#11436=VERTEX_POINT('',#36614);
#11437=VERTEX_POINT('',#36618);
#11438=VERTEX_POINT('',#36622);
#11439=VERTEX_POINT('',#36624);
#11440=VERTEX_POINT('',#36626);
#11441=VERTEX_POINT('',#36628);
#11442=VERTEX_POINT('',#36632);
#11443=VERTEX_POINT('',#36634);
#11444=VERTEX_POINT('',#36636);
#11445=VERTEX_POINT('',#36640);
#11446=VERTEX_POINT('',#36644);
#11447=VERTEX_POINT('',#36646);
#11448=VERTEX_POINT('',#36648);
#11449=VERTEX_POINT('',#36650);
#11450=VERTEX_POINT('',#36654);
#11451=VERTEX_POINT('',#36656);
#11452=VERTEX_POINT('',#36658);
#11453=VERTEX_POINT('',#36662);
#11454=VERTEX_POINT('',#36666);
#11455=VERTEX_POINT('',#36668);
#11456=VERTEX_POINT('',#36670);
#11457=VERTEX_POINT('',#36672);
#11458=VERTEX_POINT('',#36676);
#11459=VERTEX_POINT('',#36678);
#11460=VERTEX_POINT('',#36680);
#11461=VERTEX_POINT('',#36684);
#11462=VERTEX_POINT('',#36688);
#11463=VERTEX_POINT('',#36690);
#11464=VERTEX_POINT('',#36692);
#11465=VERTEX_POINT('',#36694);
#11466=VERTEX_POINT('',#36698);
#11467=VERTEX_POINT('',#36700);
#11468=VERTEX_POINT('',#36702);
#11469=VERTEX_POINT('',#36706);
#11470=VERTEX_POINT('',#36710);
#11471=VERTEX_POINT('',#36712);
#11472=VERTEX_POINT('',#36714);
#11473=VERTEX_POINT('',#36716);
#11474=VERTEX_POINT('',#36720);
#11475=VERTEX_POINT('',#36722);
#11476=VERTEX_POINT('',#36724);
#11477=VERTEX_POINT('',#36728);
#11478=VERTEX_POINT('',#36732);
#11479=VERTEX_POINT('',#36734);
#11480=VERTEX_POINT('',#36736);
#11481=VERTEX_POINT('',#36738);
#11482=VERTEX_POINT('',#36742);
#11483=VERTEX_POINT('',#36744);
#11484=VERTEX_POINT('',#36746);
#11485=VERTEX_POINT('',#36750);
#11486=VERTEX_POINT('',#36754);
#11487=VERTEX_POINT('',#36756);
#11488=VERTEX_POINT('',#36758);
#11489=VERTEX_POINT('',#36760);
#11490=VERTEX_POINT('',#36764);
#11491=VERTEX_POINT('',#36766);
#11492=VERTEX_POINT('',#36768);
#11493=VERTEX_POINT('',#36772);
#11494=VERTEX_POINT('',#36776);
#11495=VERTEX_POINT('',#36777);
#11496=VERTEX_POINT('',#36779);
#11497=VERTEX_POINT('',#36782);
#11498=VERTEX_POINT('',#36786);
#11499=VERTEX_POINT('',#36788);
#11500=VERTEX_POINT('',#36792);
#11501=VERTEX_POINT('',#36796);
#11502=VERTEX_POINT('',#36797);
#11503=VERTEX_POINT('',#36799);
#11504=VERTEX_POINT('',#36802);
#11505=VERTEX_POINT('',#36806);
#11506=VERTEX_POINT('',#36808);
#11507=VERTEX_POINT('',#36812);
#11508=VERTEX_POINT('',#36816);
#11509=VERTEX_POINT('',#36817);
#11510=VERTEX_POINT('',#36819);
#11511=VERTEX_POINT('',#36822);
#11512=VERTEX_POINT('',#36826);
#11513=VERTEX_POINT('',#36828);
#11514=VERTEX_POINT('',#36832);
#11515=VERTEX_POINT('',#36836);
#11516=VERTEX_POINT('',#36837);
#11517=VERTEX_POINT('',#36839);
#11518=VERTEX_POINT('',#36842);
#11519=VERTEX_POINT('',#36846);
#11520=VERTEX_POINT('',#36848);
#11521=VERTEX_POINT('',#36852);
#11522=VERTEX_POINT('',#36856);
#11523=VERTEX_POINT('',#36857);
#11524=VERTEX_POINT('',#36859);
#11525=VERTEX_POINT('',#36862);
#11526=VERTEX_POINT('',#36866);
#11527=VERTEX_POINT('',#36868);
#11528=VERTEX_POINT('',#36872);
#11529=VERTEX_POINT('',#36876);
#11530=VERTEX_POINT('',#36877);
#11531=VERTEX_POINT('',#36879);
#11532=VERTEX_POINT('',#36882);
#11533=VERTEX_POINT('',#36886);
#11534=VERTEX_POINT('',#36888);
#11535=VERTEX_POINT('',#36892);
#11536=VERTEX_POINT('',#36896);
#11537=VERTEX_POINT('',#36897);
#11538=VERTEX_POINT('',#36899);
#11539=VERTEX_POINT('',#36902);
#11540=VERTEX_POINT('',#36906);
#11541=VERTEX_POINT('',#36908);
#11542=VERTEX_POINT('',#36912);
#11543=VERTEX_POINT('',#36916);
#11544=VERTEX_POINT('',#36917);
#11545=VERTEX_POINT('',#36919);
#11546=VERTEX_POINT('',#36922);
#11547=VERTEX_POINT('',#36926);
#11548=VERTEX_POINT('',#36928);
#11549=VERTEX_POINT('',#36932);
#11550=VERTEX_POINT('',#36936);
#11551=VERTEX_POINT('',#36937);
#11552=VERTEX_POINT('',#36939);
#11553=VERTEX_POINT('',#36942);
#11554=VERTEX_POINT('',#36946);
#11555=VERTEX_POINT('',#36948);
#11556=VERTEX_POINT('',#36952);
#11557=VERTEX_POINT('',#36956);
#11558=VERTEX_POINT('',#36957);
#11559=VERTEX_POINT('',#36959);
#11560=VERTEX_POINT('',#36962);
#11561=VERTEX_POINT('',#36966);
#11562=VERTEX_POINT('',#36968);
#11563=VERTEX_POINT('',#36972);
#11564=VERTEX_POINT('',#36976);
#11565=VERTEX_POINT('',#36977);
#11566=VERTEX_POINT('',#36979);
#11567=VERTEX_POINT('',#36982);
#11568=VERTEX_POINT('',#36986);
#11569=VERTEX_POINT('',#36988);
#11570=VERTEX_POINT('',#36992);
#11571=VERTEX_POINT('',#36996);
#11572=VERTEX_POINT('',#36997);
#11573=VERTEX_POINT('',#36999);
#11574=VERTEX_POINT('',#37002);
#11575=VERTEX_POINT('',#37006);
#11576=VERTEX_POINT('',#37008);
#11577=VERTEX_POINT('',#37012);
#11578=VERTEX_POINT('',#37016);
#11579=VERTEX_POINT('',#37018);
#11580=VERTEX_POINT('',#37020);
#11581=VERTEX_POINT('',#37024);
#11582=VERTEX_POINT('',#37026);
#11583=VERTEX_POINT('',#37028);
#11584=VERTEX_POINT('',#37030);
#11585=VERTEX_POINT('',#37032);
#11586=VERTEX_POINT('',#37034);
#11587=VERTEX_POINT('',#37036);
#11588=VERTEX_POINT('',#37038);
#11589=VERTEX_POINT('',#37040);
#11590=VERTEX_POINT('',#37042);
#11591=VERTEX_POINT('',#37044);
#11592=VERTEX_POINT('',#37046);
#11593=VERTEX_POINT('',#37048);
#11594=VERTEX_POINT('',#37050);
#11595=VERTEX_POINT('',#37052);
#11596=VERTEX_POINT('',#37054);
#11597=VERTEX_POINT('',#37056);
#11598=VERTEX_POINT('',#37059);
#11599=VERTEX_POINT('',#37061);
#11600=VERTEX_POINT('',#37063);
#11601=VERTEX_POINT('',#37065);
#11602=VERTEX_POINT('',#37067);
#11603=VERTEX_POINT('',#37069);
#11604=VERTEX_POINT('',#37071);
#11605=VERTEX_POINT('',#37073);
#11606=VERTEX_POINT('',#37075);
#11607=VERTEX_POINT('',#37077);
#11608=VERTEX_POINT('',#37079);
#11609=VERTEX_POINT('',#37081);
#11610=VERTEX_POINT('',#37083);
#11611=VERTEX_POINT('',#37085);
#11612=VERTEX_POINT('',#37087);
#11613=VERTEX_POINT('',#37089);
#11614=VERTEX_POINT('',#37091);
#11615=VERTEX_POINT('',#37093);
#11616=VERTEX_POINT('',#37096);
#11617=VERTEX_POINT('',#37098);
#11618=VERTEX_POINT('',#37100);
#11619=VERTEX_POINT('',#37102);
#11620=VERTEX_POINT('',#37104);
#11621=VERTEX_POINT('',#37106);
#11622=VERTEX_POINT('',#37108);
#11623=VERTEX_POINT('',#37110);
#11624=VERTEX_POINT('',#37112);
#11625=VERTEX_POINT('',#37114);
#11626=VERTEX_POINT('',#37116);
#11627=VERTEX_POINT('',#37118);
#11628=VERTEX_POINT('',#37120);
#11629=VERTEX_POINT('',#37122);
#11630=VERTEX_POINT('',#37124);
#11631=VERTEX_POINT('',#37126);
#11632=VERTEX_POINT('',#37128);
#11633=VERTEX_POINT('',#37130);
#11634=VERTEX_POINT('',#37133);
#11635=VERTEX_POINT('',#37135);
#11636=VERTEX_POINT('',#37137);
#11637=VERTEX_POINT('',#37139);
#11638=VERTEX_POINT('',#37141);
#11639=VERTEX_POINT('',#37143);
#11640=VERTEX_POINT('',#37145);
#11641=VERTEX_POINT('',#37147);
#11642=VERTEX_POINT('',#37149);
#11643=VERTEX_POINT('',#37151);
#11644=VERTEX_POINT('',#37153);
#11645=VERTEX_POINT('',#37155);
#11646=VERTEX_POINT('',#37157);
#11647=VERTEX_POINT('',#37159);
#11648=VERTEX_POINT('',#37161);
#11649=VERTEX_POINT('',#37163);
#11650=VERTEX_POINT('',#37165);
#11651=VERTEX_POINT('',#37167);
#11652=VERTEX_POINT('',#37170);
#11653=VERTEX_POINT('',#37172);
#11654=VERTEX_POINT('',#37174);
#11655=VERTEX_POINT('',#37176);
#11656=VERTEX_POINT('',#37178);
#11657=VERTEX_POINT('',#37180);
#11658=VERTEX_POINT('',#37182);
#11659=VERTEX_POINT('',#37184);
#11660=VERTEX_POINT('',#37186);
#11661=VERTEX_POINT('',#37188);
#11662=VERTEX_POINT('',#37190);
#11663=VERTEX_POINT('',#37192);
#11664=VERTEX_POINT('',#37194);
#11665=VERTEX_POINT('',#37196);
#11666=VERTEX_POINT('',#37198);
#11667=VERTEX_POINT('',#37200);
#11668=VERTEX_POINT('',#37202);
#11669=VERTEX_POINT('',#37204);
#11670=VERTEX_POINT('',#37207);
#11671=VERTEX_POINT('',#37209);
#11672=VERTEX_POINT('',#37211);
#11673=VERTEX_POINT('',#37213);
#11674=VERTEX_POINT('',#37215);
#11675=VERTEX_POINT('',#37217);
#11676=VERTEX_POINT('',#37219);
#11677=VERTEX_POINT('',#37221);
#11678=VERTEX_POINT('',#37223);
#11679=VERTEX_POINT('',#37225);
#11680=VERTEX_POINT('',#37227);
#11681=VERTEX_POINT('',#37229);
#11682=VERTEX_POINT('',#37231);
#11683=VERTEX_POINT('',#37233);
#11684=VERTEX_POINT('',#37235);
#11685=VERTEX_POINT('',#37237);
#11686=VERTEX_POINT('',#37239);
#11687=VERTEX_POINT('',#37241);
#11688=VERTEX_POINT('',#37244);
#11689=VERTEX_POINT('',#37246);
#11690=VERTEX_POINT('',#37248);
#11691=VERTEX_POINT('',#37250);
#11692=VERTEX_POINT('',#37252);
#11693=VERTEX_POINT('',#37254);
#11694=VERTEX_POINT('',#37256);
#11695=VERTEX_POINT('',#37258);
#11696=VERTEX_POINT('',#37260);
#11697=VERTEX_POINT('',#37262);
#11698=VERTEX_POINT('',#37264);
#11699=VERTEX_POINT('',#37266);
#11700=VERTEX_POINT('',#37268);
#11701=VERTEX_POINT('',#37270);
#11702=VERTEX_POINT('',#37272);
#11703=VERTEX_POINT('',#37274);
#11704=VERTEX_POINT('',#37276);
#11705=VERTEX_POINT('',#37278);
#11706=VERTEX_POINT('',#37281);
#11707=VERTEX_POINT('',#37283);
#11708=VERTEX_POINT('',#37285);
#11709=VERTEX_POINT('',#37287);
#11710=VERTEX_POINT('',#37289);
#11711=VERTEX_POINT('',#37291);
#11712=VERTEX_POINT('',#37293);
#11713=VERTEX_POINT('',#37295);
#11714=VERTEX_POINT('',#37297);
#11715=VERTEX_POINT('',#37299);
#11716=VERTEX_POINT('',#37301);
#11717=VERTEX_POINT('',#37303);
#11718=VERTEX_POINT('',#37305);
#11719=VERTEX_POINT('',#37307);
#11720=VERTEX_POINT('',#37309);
#11721=VERTEX_POINT('',#37311);
#11722=VERTEX_POINT('',#37313);
#11723=VERTEX_POINT('',#37315);
#11724=VERTEX_POINT('',#37318);
#11725=VERTEX_POINT('',#37320);
#11726=VERTEX_POINT('',#37322);
#11727=VERTEX_POINT('',#37324);
#11728=VERTEX_POINT('',#37326);
#11729=VERTEX_POINT('',#37328);
#11730=VERTEX_POINT('',#37330);
#11731=VERTEX_POINT('',#37332);
#11732=VERTEX_POINT('',#37334);
#11733=VERTEX_POINT('',#37336);
#11734=VERTEX_POINT('',#37338);
#11735=VERTEX_POINT('',#37340);
#11736=VERTEX_POINT('',#37342);
#11737=VERTEX_POINT('',#37344);
#11738=VERTEX_POINT('',#37346);
#11739=VERTEX_POINT('',#37348);
#11740=VERTEX_POINT('',#37350);
#11741=VERTEX_POINT('',#37352);
#11742=VERTEX_POINT('',#37355);
#11743=VERTEX_POINT('',#37357);
#11744=VERTEX_POINT('',#37359);
#11745=VERTEX_POINT('',#37361);
#11746=VERTEX_POINT('',#37363);
#11747=VERTEX_POINT('',#37365);
#11748=VERTEX_POINT('',#37367);
#11749=VERTEX_POINT('',#37369);
#11750=VERTEX_POINT('',#37371);
#11751=VERTEX_POINT('',#37373);
#11752=VERTEX_POINT('',#37375);
#11753=VERTEX_POINT('',#37377);
#11754=VERTEX_POINT('',#37379);
#11755=VERTEX_POINT('',#37381);
#11756=VERTEX_POINT('',#37383);
#11757=VERTEX_POINT('',#37385);
#11758=VERTEX_POINT('',#37387);
#11759=VERTEX_POINT('',#37389);
#11760=VERTEX_POINT('',#37392);
#11761=VERTEX_POINT('',#37394);
#11762=VERTEX_POINT('',#37396);
#11763=VERTEX_POINT('',#37398);
#11764=VERTEX_POINT('',#37400);
#11765=VERTEX_POINT('',#37402);
#11766=VERTEX_POINT('',#37404);
#11767=VERTEX_POINT('',#37406);
#11768=VERTEX_POINT('',#37408);
#11769=VERTEX_POINT('',#37410);
#11770=VERTEX_POINT('',#37412);
#11771=VERTEX_POINT('',#37414);
#11772=VERTEX_POINT('',#37416);
#11773=VERTEX_POINT('',#37418);
#11774=VERTEX_POINT('',#37420);
#11775=VERTEX_POINT('',#37422);
#11776=VERTEX_POINT('',#37424);
#11777=VERTEX_POINT('',#37426);
#11778=VERTEX_POINT('',#37429);
#11779=VERTEX_POINT('',#37431);
#11780=VERTEX_POINT('',#37433);
#11781=VERTEX_POINT('',#37435);
#11782=VERTEX_POINT('',#37437);
#11783=VERTEX_POINT('',#37439);
#11784=VERTEX_POINT('',#37441);
#11785=VERTEX_POINT('',#37443);
#11786=VERTEX_POINT('',#37445);
#11787=VERTEX_POINT('',#37447);
#11788=VERTEX_POINT('',#37449);
#11789=VERTEX_POINT('',#37451);
#11790=VERTEX_POINT('',#37453);
#11791=VERTEX_POINT('',#37455);
#11792=VERTEX_POINT('',#37457);
#11793=VERTEX_POINT('',#37459);
#11794=VERTEX_POINT('',#37461);
#11795=VERTEX_POINT('',#37463);
#11796=VERTEX_POINT('',#37466);
#11797=VERTEX_POINT('',#37469);
#11798=VERTEX_POINT('',#37474);
#11799=VERTEX_POINT('',#37476);
#11800=VERTEX_POINT('',#37480);
#11801=VERTEX_POINT('',#37485);
#11802=VERTEX_POINT('',#37487);
#11803=VERTEX_POINT('',#37491);
#11804=VERTEX_POINT('',#37496);
#11805=VERTEX_POINT('',#37498);
#11806=VERTEX_POINT('',#37502);
#11807=VERTEX_POINT('',#37507);
#11808=VERTEX_POINT('',#37509);
#11809=VERTEX_POINT('',#37513);
#11810=VERTEX_POINT('',#37518);
#11811=VERTEX_POINT('',#37520);
#11812=VERTEX_POINT('',#37524);
#11813=VERTEX_POINT('',#37529);
#11814=VERTEX_POINT('',#37531);
#11815=VERTEX_POINT('',#37535);
#11816=VERTEX_POINT('',#37540);
#11817=VERTEX_POINT('',#37542);
#11818=VERTEX_POINT('',#37546);
#11819=VERTEX_POINT('',#37551);
#11820=VERTEX_POINT('',#37553);
#11821=VERTEX_POINT('',#37557);
#11822=VERTEX_POINT('',#37562);
#11823=VERTEX_POINT('',#37564);
#11824=VERTEX_POINT('',#37568);
#11825=VERTEX_POINT('',#37573);
#11826=VERTEX_POINT('',#37575);
#11827=VERTEX_POINT('',#37579);
#11828=VERTEX_POINT('',#37584);
#11829=VERTEX_POINT('',#37586);
#11830=VERTEX_POINT('',#37590);
#11831=VERTEX_POINT('',#37595);
#11832=VERTEX_POINT('',#37596);
#11833=VERTEX_POINT('',#37598);
#11834=VERTEX_POINT('',#37600);
#11835=VERTEX_POINT('',#37604);
#11836=VERTEX_POINT('',#37606);
#11837=VERTEX_POINT('',#37610);
#11838=VERTEX_POINT('',#37612);
#11839=VERTEX_POINT('',#38076);
#11840=VERTEX_POINT('',#38080);
#11841=VERTEX_POINT('',#38083);
#11842=VERTEX_POINT('',#38087);
#11843=VERTEX_POINT('',#38092);
#13716=EDGE_CURVE('',#11157,#11158,#4867,.T.);
#13717=EDGE_CURVE('',#11158,#11159,#4868,.T.);
#13718=EDGE_CURVE('',#11159,#11160,#4869,.F.);
#13719=EDGE_CURVE('',#11160,#11161,#4870,.T.);
#13720=EDGE_CURVE('',#11161,#11162,#4871,.T.);
#13721=EDGE_CURVE('',#11162,#11157,#4872,.T.);
#13722=EDGE_CURVE('',#11163,#11159,#4873,.T.);
#13723=EDGE_CURVE('',#11158,#11164,#4874,.T.);
#13724=EDGE_CURVE('',#11164,#11165,#4875,.T.);
#13725=EDGE_CURVE('',#11165,#11166,#4876,.T.);
#13726=EDGE_CURVE('',#11166,#11167,#4877,.T.);
#13727=EDGE_CURVE('',#11167,#11168,#4878,.T.);
#13728=EDGE_CURVE('',#11168,#11169,#4879,.T.);
#13729=EDGE_CURVE('',#11169,#11170,#4880,.T.);
#13730=EDGE_CURVE('',#11170,#11171,#4881,.T.);
#13731=EDGE_CURVE('',#11171,#11172,#4882,.T.);
#13732=EDGE_CURVE('',#11172,#11173,#4883,.T.);
#13733=EDGE_CURVE('',#11173,#11174,#4884,.T.);
#13734=EDGE_CURVE('',#11174,#11175,#4885,.T.);
#13735=EDGE_CURVE('',#11175,#11176,#4886,.T.);
#13736=EDGE_CURVE('',#11176,#11177,#4887,.T.);
#13737=EDGE_CURVE('',#11177,#11178,#4888,.T.);
#13738=EDGE_CURVE('',#11178,#11179,#4889,.T.);
#13739=EDGE_CURVE('',#11180,#11179,#4890,.T.);
#13740=EDGE_CURVE('',#11180,#11181,#4891,.T.);
#13741=EDGE_CURVE('',#11181,#11182,#4892,.T.);
#13742=EDGE_CURVE('',#11183,#11182,#4893,.T.);
#13743=EDGE_CURVE('',#11183,#11184,#4894,.T.);
#13744=EDGE_CURVE('',#11184,#11185,#4895,.T.);
#13745=EDGE_CURVE('',#11185,#11186,#4896,.T.);
#13746=EDGE_CURVE('',#11186,#11187,#4897,.T.);
#13747=EDGE_CURVE('',#11187,#11188,#4898,.T.);
#13748=EDGE_CURVE('',#11188,#11189,#4899,.T.);
#13749=EDGE_CURVE('',#11189,#11190,#4900,.T.);
#13750=EDGE_CURVE('',#11190,#11191,#4901,.T.);
#13751=EDGE_CURVE('',#11191,#11192,#4902,.T.);
#13752=EDGE_CURVE('',#11192,#11193,#4903,.T.);
#13753=EDGE_CURVE('',#11193,#11194,#4904,.T.);
#13754=EDGE_CURVE('',#11194,#11195,#4905,.T.);
#13755=EDGE_CURVE('',#11195,#11196,#4906,.T.);
#13756=EDGE_CURVE('',#11196,#11197,#4907,.T.);
#13757=EDGE_CURVE('',#11197,#11198,#4908,.T.);
#13758=EDGE_CURVE('',#11198,#11199,#4909,.T.);
#13759=EDGE_CURVE('',#11200,#11199,#4910,.T.);
#13760=EDGE_CURVE('',#11200,#11201,#4911,.T.);
#13761=EDGE_CURVE('',#11201,#11202,#4912,.T.);
#13762=EDGE_CURVE('',#11203,#11202,#4913,.T.);
#13763=EDGE_CURVE('',#11203,#11204,#4914,.T.);
#13764=EDGE_CURVE('',#11204,#11205,#4915,.T.);
#13765=EDGE_CURVE('',#11205,#11206,#4916,.T.);
#13766=EDGE_CURVE('',#11206,#11207,#4917,.T.);
#13767=EDGE_CURVE('',#11207,#11208,#4918,.T.);
#13768=EDGE_CURVE('',#11208,#11209,#4919,.T.);
#13769=EDGE_CURVE('',#11209,#11210,#4920,.T.);
#13770=EDGE_CURVE('',#11210,#11211,#4921,.T.);
#13771=EDGE_CURVE('',#11211,#11212,#4922,.T.);
#13772=EDGE_CURVE('',#11212,#11213,#4923,.T.);
#13773=EDGE_CURVE('',#11213,#11214,#4924,.T.);
#13774=EDGE_CURVE('',#11214,#11215,#4925,.T.);
#13775=EDGE_CURVE('',#11215,#11216,#4926,.T.);
#13776=EDGE_CURVE('',#11216,#11217,#4927,.T.);
#13777=EDGE_CURVE('',#11217,#11218,#4928,.T.);
#13778=EDGE_CURVE('',#11218,#11219,#4929,.T.);
#13779=EDGE_CURVE('',#11220,#11219,#4930,.T.);
#13780=EDGE_CURVE('',#11220,#11221,#4931,.T.);
#13781=EDGE_CURVE('',#11221,#11222,#4932,.T.);
#13782=EDGE_CURVE('',#11223,#11222,#4933,.T.);
#13783=EDGE_CURVE('',#11223,#11224,#4934,.T.);
#13784=EDGE_CURVE('',#11224,#11225,#4935,.T.);
#13785=EDGE_CURVE('',#11225,#11226,#4936,.T.);
#13786=EDGE_CURVE('',#11226,#11227,#4937,.T.);
#13787=EDGE_CURVE('',#11227,#11228,#4938,.T.);
#13788=EDGE_CURVE('',#11228,#11229,#4939,.T.);
#13789=EDGE_CURVE('',#11229,#11230,#4940,.T.);
#13790=EDGE_CURVE('',#11230,#11231,#4941,.T.);
#13791=EDGE_CURVE('',#11231,#11232,#4942,.T.);
#13792=EDGE_CURVE('',#11232,#11233,#4943,.T.);
#13793=EDGE_CURVE('',#11233,#11234,#4944,.T.);
#13794=EDGE_CURVE('',#11234,#11235,#4945,.T.);
#13795=EDGE_CURVE('',#11235,#11236,#4946,.T.);
#13796=EDGE_CURVE('',#11236,#11237,#4947,.T.);
#13797=EDGE_CURVE('',#11237,#11238,#4948,.T.);
#13798=EDGE_CURVE('',#11238,#11239,#4949,.T.);
#13799=EDGE_CURVE('',#11240,#11239,#4950,.T.);
#13800=EDGE_CURVE('',#11240,#11241,#4951,.T.);
#13801=EDGE_CURVE('',#11241,#11242,#4952,.T.);
#13802=EDGE_CURVE('',#11243,#11242,#4953,.T.);
#13803=EDGE_CURVE('',#11243,#11244,#4954,.T.);
#13804=EDGE_CURVE('',#11244,#11245,#4955,.T.);
#13805=EDGE_CURVE('',#11245,#11246,#4956,.T.);
#13806=EDGE_CURVE('',#11246,#11247,#4957,.T.);
#13807=EDGE_CURVE('',#11247,#11248,#4958,.T.);
#13808=EDGE_CURVE('',#11248,#11249,#4959,.T.);
#13809=EDGE_CURVE('',#11249,#11250,#4960,.T.);
#13810=EDGE_CURVE('',#11250,#11251,#4961,.T.);
#13811=EDGE_CURVE('',#11251,#11252,#4962,.T.);
#13812=EDGE_CURVE('',#11252,#11253,#4963,.T.);
#13813=EDGE_CURVE('',#11253,#11254,#4964,.T.);
#13814=EDGE_CURVE('',#11254,#11255,#4965,.T.);
#13815=EDGE_CURVE('',#11255,#11256,#4966,.T.);
#13816=EDGE_CURVE('',#11256,#11257,#4967,.T.);
#13817=EDGE_CURVE('',#11257,#11258,#4968,.T.);
#13818=EDGE_CURVE('',#11258,#11259,#4969,.T.);
#13819=EDGE_CURVE('',#11260,#11259,#4970,.T.);
#13820=EDGE_CURVE('',#11260,#11261,#4971,.T.);
#13821=EDGE_CURVE('',#11261,#11262,#4972,.T.);
#13822=EDGE_CURVE('',#11263,#11262,#4973,.T.);
#13823=EDGE_CURVE('',#11263,#11264,#4974,.T.);
#13824=EDGE_CURVE('',#11264,#11265,#4975,.T.);
#13825=EDGE_CURVE('',#11265,#11266,#4976,.T.);
#13826=EDGE_CURVE('',#11266,#11267,#4977,.T.);
#13827=EDGE_CURVE('',#11267,#11268,#4978,.T.);
#13828=EDGE_CURVE('',#11268,#11269,#4979,.T.);
#13829=EDGE_CURVE('',#11269,#11270,#4980,.T.);
#13830=EDGE_CURVE('',#11270,#11271,#4981,.T.);
#13831=EDGE_CURVE('',#11271,#11272,#4982,.T.);
#13832=EDGE_CURVE('',#11272,#11273,#4983,.T.);
#13833=EDGE_CURVE('',#11273,#11274,#4984,.T.);
#13834=EDGE_CURVE('',#11274,#11275,#4985,.T.);
#13835=EDGE_CURVE('',#11275,#11276,#4986,.T.);
#13836=EDGE_CURVE('',#11276,#11277,#4987,.T.);
#13837=EDGE_CURVE('',#11277,#11278,#4988,.T.);
#13838=EDGE_CURVE('',#11278,#11279,#4989,.T.);
#13839=EDGE_CURVE('',#11280,#11279,#4990,.T.);
#13840=EDGE_CURVE('',#11280,#11281,#4991,.T.);
#13841=EDGE_CURVE('',#11281,#11282,#4992,.T.);
#13842=EDGE_CURVE('',#11283,#11282,#4993,.T.);
#13843=EDGE_CURVE('',#11283,#11284,#4994,.T.);
#13844=EDGE_CURVE('',#11284,#11285,#4995,.T.);
#13845=EDGE_CURVE('',#11285,#11286,#4996,.T.);
#13846=EDGE_CURVE('',#11286,#11287,#4997,.T.);
#13847=EDGE_CURVE('',#11287,#11288,#4998,.T.);
#13848=EDGE_CURVE('',#11288,#11289,#4999,.T.);
#13849=EDGE_CURVE('',#11289,#11290,#5000,.T.);
#13850=EDGE_CURVE('',#11290,#11291,#5001,.T.);
#13851=EDGE_CURVE('',#11291,#11292,#5002,.T.);
#13852=EDGE_CURVE('',#11292,#11293,#5003,.T.);
#13853=EDGE_CURVE('',#11293,#11294,#5004,.T.);
#13854=EDGE_CURVE('',#11294,#11295,#5005,.T.);
#13855=EDGE_CURVE('',#11295,#11296,#5006,.T.);
#13856=EDGE_CURVE('',#11296,#11297,#5007,.T.);
#13857=EDGE_CURVE('',#11297,#11298,#5008,.T.);
#13858=EDGE_CURVE('',#11298,#11299,#5009,.T.);
#13859=EDGE_CURVE('',#11300,#11299,#5010,.T.);
#13860=EDGE_CURVE('',#11300,#11301,#5011,.T.);
#13861=EDGE_CURVE('',#11301,#11302,#5012,.T.);
#13862=EDGE_CURVE('',#11303,#11302,#5013,.T.);
#13863=EDGE_CURVE('',#11303,#11304,#5014,.T.);
#13864=EDGE_CURVE('',#11304,#11305,#5015,.T.);
#13865=EDGE_CURVE('',#11305,#11306,#5016,.T.);
#13866=EDGE_CURVE('',#11306,#11307,#5017,.T.);
#13867=EDGE_CURVE('',#11307,#11308,#5018,.T.);
#13868=EDGE_CURVE('',#11308,#11309,#5019,.T.);
#13869=EDGE_CURVE('',#11309,#11310,#5020,.T.);
#13870=EDGE_CURVE('',#11310,#11311,#5021,.T.);
#13871=EDGE_CURVE('',#11311,#11312,#5022,.T.);
#13872=EDGE_CURVE('',#11312,#11313,#5023,.T.);
#13873=EDGE_CURVE('',#11313,#11314,#5024,.T.);
#13874=EDGE_CURVE('',#11314,#11315,#5025,.T.);
#13875=EDGE_CURVE('',#11315,#11316,#5026,.T.);
#13876=EDGE_CURVE('',#11316,#11317,#5027,.T.);
#13877=EDGE_CURVE('',#11317,#11318,#5028,.T.);
#13878=EDGE_CURVE('',#11318,#11319,#5029,.T.);
#13879=EDGE_CURVE('',#11320,#11319,#5030,.T.);
#13880=EDGE_CURVE('',#11320,#11321,#5031,.T.);
#13881=EDGE_CURVE('',#11321,#11322,#5032,.T.);
#13882=EDGE_CURVE('',#11323,#11322,#5033,.T.);
#13883=EDGE_CURVE('',#11323,#11324,#5034,.T.);
#13884=EDGE_CURVE('',#11324,#11325,#5035,.T.);
#13885=EDGE_CURVE('',#11325,#11326,#5036,.T.);
#13886=EDGE_CURVE('',#11326,#11327,#5037,.T.);
#13887=EDGE_CURVE('',#11327,#11328,#5038,.T.);
#13888=EDGE_CURVE('',#11328,#11329,#5039,.T.);
#13889=EDGE_CURVE('',#11329,#11330,#5040,.T.);
#13890=EDGE_CURVE('',#11330,#11331,#5041,.T.);
#13891=EDGE_CURVE('',#11331,#11332,#5042,.T.);
#13892=EDGE_CURVE('',#11332,#11333,#5043,.T.);
#13893=EDGE_CURVE('',#11333,#11334,#5044,.T.);
#13894=EDGE_CURVE('',#11334,#11335,#5045,.T.);
#13895=EDGE_CURVE('',#11335,#11336,#5046,.T.);
#13896=EDGE_CURVE('',#11336,#11337,#5047,.T.);
#13897=EDGE_CURVE('',#11337,#11338,#5048,.T.);
#13898=EDGE_CURVE('',#11338,#11339,#5049,.T.);
#13899=EDGE_CURVE('',#11340,#11339,#5050,.T.);
#13900=EDGE_CURVE('',#11340,#11341,#5051,.T.);
#13901=EDGE_CURVE('',#11341,#11342,#5052,.T.);
#13902=EDGE_CURVE('',#11343,#11342,#5053,.T.);
#13903=EDGE_CURVE('',#11343,#11344,#5054,.T.);
#13904=EDGE_CURVE('',#11344,#11345,#5055,.T.);
#13905=EDGE_CURVE('',#11345,#11346,#5056,.T.);
#13906=EDGE_CURVE('',#11346,#11347,#5057,.T.);
#13907=EDGE_CURVE('',#11347,#11348,#5058,.T.);
#13908=EDGE_CURVE('',#11348,#11349,#5059,.T.);
#13909=EDGE_CURVE('',#11349,#11350,#5060,.T.);
#13910=EDGE_CURVE('',#11350,#11351,#5061,.T.);
#13911=EDGE_CURVE('',#11351,#11352,#5062,.T.);
#13912=EDGE_CURVE('',#11352,#11353,#5063,.T.);
#13913=EDGE_CURVE('',#11353,#11354,#5064,.T.);
#13914=EDGE_CURVE('',#11354,#11355,#5065,.T.);
#13915=EDGE_CURVE('',#11355,#11356,#5066,.T.);
#13916=EDGE_CURVE('',#11356,#11357,#5067,.T.);
#13917=EDGE_CURVE('',#11357,#11358,#5068,.T.);
#13918=EDGE_CURVE('',#11358,#11359,#5069,.T.);
#13919=EDGE_CURVE('',#11360,#11359,#5070,.T.);
#13920=EDGE_CURVE('',#11360,#11361,#5071,.T.);
#13921=EDGE_CURVE('',#11361,#11362,#5072,.T.);
#13922=EDGE_CURVE('',#11363,#11362,#5073,.T.);
#13923=EDGE_CURVE('',#11363,#11364,#5074,.T.);
#13924=EDGE_CURVE('',#11364,#11365,#5075,.T.);
#13925=EDGE_CURVE('',#11365,#11366,#5076,.T.);
#13926=EDGE_CURVE('',#11366,#11367,#5077,.T.);
#13927=EDGE_CURVE('',#11367,#11368,#5078,.T.);
#13928=EDGE_CURVE('',#11368,#11369,#5079,.T.);
#13929=EDGE_CURVE('',#11369,#11370,#5080,.T.);
#13930=EDGE_CURVE('',#11370,#11371,#5081,.T.);
#13931=EDGE_CURVE('',#11371,#11372,#5082,.T.);
#13932=EDGE_CURVE('',#11372,#11373,#5083,.T.);
#13933=EDGE_CURVE('',#11373,#11374,#5084,.T.);
#13934=EDGE_CURVE('',#11374,#11375,#5085,.T.);
#13935=EDGE_CURVE('',#11375,#11376,#5086,.T.);
#13936=EDGE_CURVE('',#11376,#11377,#5087,.T.);
#13937=EDGE_CURVE('',#11377,#11378,#5088,.T.);
#13938=EDGE_CURVE('',#11378,#11379,#5089,.T.);
#13939=EDGE_CURVE('',#11380,#11379,#5090,.T.);
#13940=EDGE_CURVE('',#11380,#11381,#5091,.T.);
#13941=EDGE_CURVE('',#11381,#11382,#5092,.T.);
#13942=EDGE_CURVE('',#11383,#11382,#5093,.T.);
#13943=EDGE_CURVE('',#11383,#11384,#5094,.T.);
#13944=EDGE_CURVE('',#11384,#11385,#5095,.T.);
#13945=EDGE_CURVE('',#11385,#11386,#5096,.T.);
#13946=EDGE_CURVE('',#11386,#11387,#5097,.T.);
#13947=EDGE_CURVE('',#11387,#11388,#5098,.T.);
#13948=EDGE_CURVE('',#11388,#11389,#5099,.T.);
#13949=EDGE_CURVE('',#11389,#11390,#5100,.T.);
#13950=EDGE_CURVE('',#11390,#11391,#5101,.T.);
#13951=EDGE_CURVE('',#11391,#11392,#5102,.T.);
#13952=EDGE_CURVE('',#11392,#11393,#5103,.T.);
#13953=EDGE_CURVE('',#11393,#11394,#5104,.T.);
#13954=EDGE_CURVE('',#11394,#11395,#5105,.T.);
#13955=EDGE_CURVE('',#11395,#11396,#5106,.T.);
#13956=EDGE_CURVE('',#11396,#11397,#5107,.T.);
#13957=EDGE_CURVE('',#11397,#11398,#5108,.T.);
#13958=EDGE_CURVE('',#11398,#11399,#5109,.T.);
#13959=EDGE_CURVE('',#11400,#11399,#5110,.T.);
#13960=EDGE_CURVE('',#11400,#11163,#5111,.T.);
#13961=EDGE_CURVE('',#11401,#11401,#10568,.T.);
#13962=EDGE_CURVE('',#11157,#11402,#5112,.T.);
#13963=EDGE_CURVE('',#11403,#11402,#5113,.T.);
#13964=EDGE_CURVE('',#11404,#11403,#5114,.T.);
#13965=EDGE_CURVE('',#11164,#11404,#5115,.T.);
#13966=EDGE_CURVE('',#11162,#11405,#5116,.T.);
#13967=EDGE_CURVE('',#11402,#11405,#5117,.T.);
#13968=EDGE_CURVE('',#11406,#11383,#5118,.T.);
#13969=EDGE_CURVE('',#11382,#11407,#5119,.F.);
#13970=EDGE_CURVE('',#11407,#11408,#5120,.T.);
#13971=EDGE_CURVE('',#11408,#11409,#5121,.T.);
#13972=EDGE_CURVE('',#11409,#11406,#5122,.T.);
#13973=EDGE_CURVE('',#11406,#11410,#5123,.T.);
#13974=EDGE_CURVE('',#11411,#11410,#5124,.T.);
#13975=EDGE_CURVE('',#11412,#11411,#5125,.T.);
#13976=EDGE_CURVE('',#11384,#11412,#5126,.T.);
#13977=EDGE_CURVE('',#11409,#11413,#5127,.T.);
#13978=EDGE_CURVE('',#11410,#11413,#5128,.T.);
#13979=EDGE_CURVE('',#11414,#11363,#5129,.T.);
#13980=EDGE_CURVE('',#11362,#11415,#5130,.F.);
#13981=EDGE_CURVE('',#11415,#11416,#5131,.T.);
#13982=EDGE_CURVE('',#11416,#11417,#5132,.T.);
#13983=EDGE_CURVE('',#11417,#11414,#5133,.T.);
#13984=EDGE_CURVE('',#11414,#11418,#5134,.T.);
#13985=EDGE_CURVE('',#11419,#11418,#5135,.T.);
#13986=EDGE_CURVE('',#11420,#11419,#5136,.T.);
#13987=EDGE_CURVE('',#11364,#11420,#5137,.T.);
#13988=EDGE_CURVE('',#11417,#11421,#5138,.T.);
#13989=EDGE_CURVE('',#11418,#11421,#5139,.T.);
#13990=EDGE_CURVE('',#11422,#11343,#5140,.T.);
#13991=EDGE_CURVE('',#11342,#11423,#5141,.F.);
#13992=EDGE_CURVE('',#11423,#11424,#5142,.T.);
#13993=EDGE_CURVE('',#11424,#11425,#5143,.T.);
#13994=EDGE_CURVE('',#11425,#11422,#5144,.T.);
#13995=EDGE_CURVE('',#11422,#11426,#5145,.T.);
#13996=EDGE_CURVE('',#11427,#11426,#5146,.T.);
#13997=EDGE_CURVE('',#11428,#11427,#5147,.T.);
#13998=EDGE_CURVE('',#11344,#11428,#5148,.T.);
#13999=EDGE_CURVE('',#11425,#11429,#5149,.T.);
#14000=EDGE_CURVE('',#11426,#11429,#5150,.T.);
#14001=EDGE_CURVE('',#11430,#11323,#5151,.T.);
#14002=EDGE_CURVE('',#11322,#11431,#5152,.F.);
#14003=EDGE_CURVE('',#11431,#11432,#5153,.T.);
#14004=EDGE_CURVE('',#11432,#11433,#5154,.T.);
#14005=EDGE_CURVE('',#11433,#11430,#5155,.T.);
#14006=EDGE_CURVE('',#11430,#11434,#5156,.T.);
#14007=EDGE_CURVE('',#11435,#11434,#5157,.T.);
#14008=EDGE_CURVE('',#11436,#11435,#5158,.T.);
#14009=EDGE_CURVE('',#11324,#11436,#5159,.T.);
#14010=EDGE_CURVE('',#11433,#11437,#5160,.T.);
#14011=EDGE_CURVE('',#11434,#11437,#5161,.T.);
#14012=EDGE_CURVE('',#11438,#11303,#5162,.T.);
#14013=EDGE_CURVE('',#11302,#11439,#5163,.F.);
#14014=EDGE_CURVE('',#11439,#11440,#5164,.T.);
#14015=EDGE_CURVE('',#11440,#11441,#5165,.T.);
#14016=EDGE_CURVE('',#11441,#11438,#5166,.T.);
#14017=EDGE_CURVE('',#11438,#11442,#5167,.T.);
#14018=EDGE_CURVE('',#11443,#11442,#5168,.T.);
#14019=EDGE_CURVE('',#11444,#11443,#5169,.T.);
#14020=EDGE_CURVE('',#11304,#11444,#5170,.T.);
#14021=EDGE_CURVE('',#11441,#11445,#5171,.T.);
#14022=EDGE_CURVE('',#11442,#11445,#5172,.T.);
#14023=EDGE_CURVE('',#11446,#11283,#5173,.T.);
#14024=EDGE_CURVE('',#11282,#11447,#5174,.F.);
#14025=EDGE_CURVE('',#11447,#11448,#5175,.T.);
#14026=EDGE_CURVE('',#11448,#11449,#5176,.T.);
#14027=EDGE_CURVE('',#11449,#11446,#5177,.T.);
#14028=EDGE_CURVE('',#11446,#11450,#5178,.T.);
#14029=EDGE_CURVE('',#11451,#11450,#5179,.T.);
#14030=EDGE_CURVE('',#11452,#11451,#5180,.T.);
#14031=EDGE_CURVE('',#11284,#11452,#5181,.T.);
#14032=EDGE_CURVE('',#11449,#11453,#5182,.T.);
#14033=EDGE_CURVE('',#11450,#11453,#5183,.T.);
#14034=EDGE_CURVE('',#11454,#11263,#5184,.T.);
#14035=EDGE_CURVE('',#11262,#11455,#5185,.F.);
#14036=EDGE_CURVE('',#11455,#11456,#5186,.T.);
#14037=EDGE_CURVE('',#11456,#11457,#5187,.T.);
#14038=EDGE_CURVE('',#11457,#11454,#5188,.T.);
#14039=EDGE_CURVE('',#11454,#11458,#5189,.T.);
#14040=EDGE_CURVE('',#11459,#11458,#5190,.T.);
#14041=EDGE_CURVE('',#11460,#11459,#5191,.T.);
#14042=EDGE_CURVE('',#11264,#11460,#5192,.T.);
#14043=EDGE_CURVE('',#11457,#11461,#5193,.T.);
#14044=EDGE_CURVE('',#11458,#11461,#5194,.T.);
#14045=EDGE_CURVE('',#11462,#11243,#5195,.T.);
#14046=EDGE_CURVE('',#11242,#11463,#5196,.F.);
#14047=EDGE_CURVE('',#11463,#11464,#5197,.T.);
#14048=EDGE_CURVE('',#11464,#11465,#5198,.T.);
#14049=EDGE_CURVE('',#11465,#11462,#5199,.T.);
#14050=EDGE_CURVE('',#11462,#11466,#5200,.T.);
#14051=EDGE_CURVE('',#11467,#11466,#5201,.T.);
#14052=EDGE_CURVE('',#11468,#11467,#5202,.T.);
#14053=EDGE_CURVE('',#11244,#11468,#5203,.T.);
#14054=EDGE_CURVE('',#11465,#11469,#5204,.T.);
#14055=EDGE_CURVE('',#11466,#11469,#5205,.T.);
#14056=EDGE_CURVE('',#11470,#11223,#5206,.T.);
#14057=EDGE_CURVE('',#11222,#11471,#5207,.F.);
#14058=EDGE_CURVE('',#11471,#11472,#5208,.T.);
#14059=EDGE_CURVE('',#11472,#11473,#5209,.T.);
#14060=EDGE_CURVE('',#11473,#11470,#5210,.T.);
#14061=EDGE_CURVE('',#11470,#11474,#5211,.T.);
#14062=EDGE_CURVE('',#11475,#11474,#5212,.T.);
#14063=EDGE_CURVE('',#11476,#11475,#5213,.T.);
#14064=EDGE_CURVE('',#11224,#11476,#5214,.T.);
#14065=EDGE_CURVE('',#11473,#11477,#5215,.T.);
#14066=EDGE_CURVE('',#11474,#11477,#5216,.T.);
#14067=EDGE_CURVE('',#11478,#11203,#5217,.T.);
#14068=EDGE_CURVE('',#11202,#11479,#5218,.F.);
#14069=EDGE_CURVE('',#11479,#11480,#5219,.T.);
#14070=EDGE_CURVE('',#11480,#11481,#5220,.T.);
#14071=EDGE_CURVE('',#11481,#11478,#5221,.T.);
#14072=EDGE_CURVE('',#11478,#11482,#5222,.T.);
#14073=EDGE_CURVE('',#11483,#11482,#5223,.T.);
#14074=EDGE_CURVE('',#11484,#11483,#5224,.T.);
#14075=EDGE_CURVE('',#11204,#11484,#5225,.T.);
#14076=EDGE_CURVE('',#11481,#11485,#5226,.T.);
#14077=EDGE_CURVE('',#11482,#11485,#5227,.T.);
#14078=EDGE_CURVE('',#11486,#11183,#5228,.T.);
#14079=EDGE_CURVE('',#11182,#11487,#5229,.F.);
#14080=EDGE_CURVE('',#11487,#11488,#5230,.T.);
#14081=EDGE_CURVE('',#11488,#11489,#5231,.T.);
#14082=EDGE_CURVE('',#11489,#11486,#5232,.T.);
#14083=EDGE_CURVE('',#11486,#11490,#5233,.T.);
#14084=EDGE_CURVE('',#11491,#11490,#5234,.T.);
#14085=EDGE_CURVE('',#11492,#11491,#5235,.T.);
#14086=EDGE_CURVE('',#11184,#11492,#5236,.T.);
#14087=EDGE_CURVE('',#11489,#11493,#5237,.T.);
#14088=EDGE_CURVE('',#11490,#11493,#5238,.T.);
#14089=EDGE_CURVE('',#11494,#11495,#5239,.T.);
#14090=EDGE_CURVE('',#11495,#11496,#5240,.T.);
#14091=EDGE_CURVE('',#11496,#11180,#5241,.F.);
#14092=EDGE_CURVE('',#11179,#11497,#5242,.T.);
#14093=EDGE_CURVE('',#11497,#11494,#5243,.T.);
#14094=EDGE_CURVE('',#11495,#11498,#5244,.T.);
#14095=EDGE_CURVE('',#11499,#11498,#5245,.T.);
#14096=EDGE_CURVE('',#11496,#11499,#5246,.T.);
#14097=EDGE_CURVE('',#11494,#11500,#5247,.T.);
#14098=EDGE_CURVE('',#11498,#11500,#5248,.T.);
#14099=EDGE_CURVE('',#11501,#11502,#5249,.T.);
#14100=EDGE_CURVE('',#11502,#11503,#5250,.T.);
#14101=EDGE_CURVE('',#11503,#11400,#5251,.F.);
#14102=EDGE_CURVE('',#11399,#11504,#5252,.T.);
#14103=EDGE_CURVE('',#11504,#11501,#5253,.T.);
#14104=EDGE_CURVE('',#11502,#11505,#5254,.T.);
#14105=EDGE_CURVE('',#11506,#11505,#5255,.T.);
#14106=EDGE_CURVE('',#11503,#11506,#5256,.T.);
#14107=EDGE_CURVE('',#11501,#11507,#5257,.T.);
#14108=EDGE_CURVE('',#11505,#11507,#5258,.T.);
#14109=EDGE_CURVE('',#11508,#11509,#5259,.T.);
#14110=EDGE_CURVE('',#11509,#11510,#5260,.T.);
#14111=EDGE_CURVE('',#11510,#11380,#5261,.F.);
#14112=EDGE_CURVE('',#11379,#11511,#5262,.T.);
#14113=EDGE_CURVE('',#11511,#11508,#5263,.T.);
#14114=EDGE_CURVE('',#11509,#11512,#5264,.T.);
#14115=EDGE_CURVE('',#11513,#11512,#5265,.T.);
#14116=EDGE_CURVE('',#11510,#11513,#5266,.T.);
#14117=EDGE_CURVE('',#11508,#11514,#5267,.T.);
#14118=EDGE_CURVE('',#11512,#11514,#5268,.T.);
#14119=EDGE_CURVE('',#11515,#11516,#5269,.T.);
#14120=EDGE_CURVE('',#11516,#11517,#5270,.T.);
#14121=EDGE_CURVE('',#11517,#11360,#5271,.F.);
#14122=EDGE_CURVE('',#11359,#11518,#5272,.T.);
#14123=EDGE_CURVE('',#11518,#11515,#5273,.T.);
#14124=EDGE_CURVE('',#11516,#11519,#5274,.T.);
#14125=EDGE_CURVE('',#11520,#11519,#5275,.T.);
#14126=EDGE_CURVE('',#11517,#11520,#5276,.T.);
#14127=EDGE_CURVE('',#11515,#11521,#5277,.T.);
#14128=EDGE_CURVE('',#11519,#11521,#5278,.T.);
#14129=EDGE_CURVE('',#11522,#11523,#5279,.T.);
#14130=EDGE_CURVE('',#11523,#11524,#5280,.T.);
#14131=EDGE_CURVE('',#11524,#11340,#5281,.F.);
#14132=EDGE_CURVE('',#11339,#11525,#5282,.T.);
#14133=EDGE_CURVE('',#11525,#11522,#5283,.T.);
#14134=EDGE_CURVE('',#11523,#11526,#5284,.T.);
#14135=EDGE_CURVE('',#11527,#11526,#5285,.T.);
#14136=EDGE_CURVE('',#11524,#11527,#5286,.T.);
#14137=EDGE_CURVE('',#11522,#11528,#5287,.T.);
#14138=EDGE_CURVE('',#11526,#11528,#5288,.T.);
#14139=EDGE_CURVE('',#11529,#11530,#5289,.T.);
#14140=EDGE_CURVE('',#11530,#11531,#5290,.T.);
#14141=EDGE_CURVE('',#11531,#11320,#5291,.F.);
#14142=EDGE_CURVE('',#11319,#11532,#5292,.T.);
#14143=EDGE_CURVE('',#11532,#11529,#5293,.T.);
#14144=EDGE_CURVE('',#11530,#11533,#5294,.T.);
#14145=EDGE_CURVE('',#11534,#11533,#5295,.T.);
#14146=EDGE_CURVE('',#11531,#11534,#5296,.T.);
#14147=EDGE_CURVE('',#11529,#11535,#5297,.T.);
#14148=EDGE_CURVE('',#11533,#11535,#5298,.T.);
#14149=EDGE_CURVE('',#11536,#11537,#5299,.T.);
#14150=EDGE_CURVE('',#11537,#11538,#5300,.T.);
#14151=EDGE_CURVE('',#11538,#11300,#5301,.F.);
#14152=EDGE_CURVE('',#11299,#11539,#5302,.T.);
#14153=EDGE_CURVE('',#11539,#11536,#5303,.T.);
#14154=EDGE_CURVE('',#11537,#11540,#5304,.T.);
#14155=EDGE_CURVE('',#11541,#11540,#5305,.T.);
#14156=EDGE_CURVE('',#11538,#11541,#5306,.T.);
#14157=EDGE_CURVE('',#11536,#11542,#5307,.T.);
#14158=EDGE_CURVE('',#11540,#11542,#5308,.T.);
#14159=EDGE_CURVE('',#11543,#11544,#5309,.T.);
#14160=EDGE_CURVE('',#11544,#11545,#5310,.T.);
#14161=EDGE_CURVE('',#11545,#11280,#5311,.F.);
#14162=EDGE_CURVE('',#11279,#11546,#5312,.T.);
#14163=EDGE_CURVE('',#11546,#11543,#5313,.T.);
#14164=EDGE_CURVE('',#11544,#11547,#5314,.T.);
#14165=EDGE_CURVE('',#11548,#11547,#5315,.T.);
#14166=EDGE_CURVE('',#11545,#11548,#5316,.T.);
#14167=EDGE_CURVE('',#11543,#11549,#5317,.T.);
#14168=EDGE_CURVE('',#11547,#11549,#5318,.T.);
#14169=EDGE_CURVE('',#11550,#11551,#5319,.T.);
#14170=EDGE_CURVE('',#11551,#11552,#5320,.T.);
#14171=EDGE_CURVE('',#11552,#11260,#5321,.F.);
#14172=EDGE_CURVE('',#11259,#11553,#5322,.T.);
#14173=EDGE_CURVE('',#11553,#11550,#5323,.T.);
#14174=EDGE_CURVE('',#11551,#11554,#5324,.T.);
#14175=EDGE_CURVE('',#11555,#11554,#5325,.T.);
#14176=EDGE_CURVE('',#11552,#11555,#5326,.T.);
#14177=EDGE_CURVE('',#11550,#11556,#5327,.T.);
#14178=EDGE_CURVE('',#11554,#11556,#5328,.T.);
#14179=EDGE_CURVE('',#11557,#11558,#5329,.T.);
#14180=EDGE_CURVE('',#11558,#11559,#5330,.T.);
#14181=EDGE_CURVE('',#11559,#11240,#5331,.F.);
#14182=EDGE_CURVE('',#11239,#11560,#5332,.T.);
#14183=EDGE_CURVE('',#11560,#11557,#5333,.T.);
#14184=EDGE_CURVE('',#11558,#11561,#5334,.T.);
#14185=EDGE_CURVE('',#11562,#11561,#5335,.T.);
#14186=EDGE_CURVE('',#11559,#11562,#5336,.T.);
#14187=EDGE_CURVE('',#11557,#11563,#5337,.T.);
#14188=EDGE_CURVE('',#11561,#11563,#5338,.T.);
#14189=EDGE_CURVE('',#11564,#11565,#5339,.T.);
#14190=EDGE_CURVE('',#11565,#11566,#5340,.T.);
#14191=EDGE_CURVE('',#11566,#11220,#5341,.F.);
#14192=EDGE_CURVE('',#11219,#11567,#5342,.T.);
#14193=EDGE_CURVE('',#11567,#11564,#5343,.T.);
#14194=EDGE_CURVE('',#11565,#11568,#5344,.T.);
#14195=EDGE_CURVE('',#11569,#11568,#5345,.T.);
#14196=EDGE_CURVE('',#11566,#11569,#5346,.T.);
#14197=EDGE_CURVE('',#11564,#11570,#5347,.T.);
#14198=EDGE_CURVE('',#11568,#11570,#5348,.T.);
#14199=EDGE_CURVE('',#11571,#11572,#5349,.T.);
#14200=EDGE_CURVE('',#11572,#11573,#5350,.T.);
#14201=EDGE_CURVE('',#11573,#11200,#5351,.F.);
#14202=EDGE_CURVE('',#11199,#11574,#5352,.T.);
#14203=EDGE_CURVE('',#11574,#11571,#5353,.T.);
#14204=EDGE_CURVE('',#11572,#11575,#5354,.T.);
#14205=EDGE_CURVE('',#11576,#11575,#5355,.T.);
#14206=EDGE_CURVE('',#11573,#11576,#5356,.T.);
#14207=EDGE_CURVE('',#11571,#11577,#5357,.T.);
#14208=EDGE_CURVE('',#11575,#11577,#5358,.T.);
#14209=EDGE_CURVE('',#11493,#11578,#5359,.T.);
#14210=EDGE_CURVE('',#11578,#11579,#5360,.T.);
#14211=EDGE_CURVE('',#11579,#11580,#5361,.F.);
#14212=EDGE_CURVE('',#11580,#11491,#5362,.T.);
#14213=EDGE_CURVE('',#11580,#11581,#5363,.T.);
#14214=EDGE_CURVE('',#11581,#11582,#5364,.T.);
#14215=EDGE_CURVE('',#11583,#11582,#5365,.T.);
#14216=EDGE_CURVE('',#11583,#11584,#5366,.T.);
#14217=EDGE_CURVE('',#11584,#11585,#5367,.T.);
#14218=EDGE_CURVE('',#11585,#11586,#5368,.T.);
#14219=EDGE_CURVE('',#11586,#11587,#5369,.T.);
#14220=EDGE_CURVE('',#11587,#11588,#5370,.T.);
#14221=EDGE_CURVE('',#11588,#11589,#5371,.T.);
#14222=EDGE_CURVE('',#11589,#11590,#5372,.T.);
#14223=EDGE_CURVE('',#11590,#11591,#5373,.T.);
#14224=EDGE_CURVE('',#11591,#11592,#5374,.T.);
#14225=EDGE_CURVE('',#11592,#11593,#5375,.T.);
#14226=EDGE_CURVE('',#11593,#11594,#5376,.T.);
#14227=EDGE_CURVE('',#11594,#11595,#5377,.T.);
#14228=EDGE_CURVE('',#11595,#11596,#5378,.T.);
#14229=EDGE_CURVE('',#11596,#11597,#5379,.T.);
#14230=EDGE_CURVE('',#11597,#11404,#5380,.T.);
#14231=EDGE_CURVE('',#11598,#11403,#5381,.T.);
#14232=EDGE_CURVE('',#11598,#11599,#5382,.T.);
#14233=EDGE_CURVE('',#11599,#11600,#5383,.T.);
#14234=EDGE_CURVE('',#11601,#11600,#5384,.T.);
#14235=EDGE_CURVE('',#11601,#11602,#5385,.T.);
#14236=EDGE_CURVE('',#11602,#11603,#5386,.T.);
#14237=EDGE_CURVE('',#11603,#11604,#5387,.T.);
#14238=EDGE_CURVE('',#11604,#11605,#5388,.T.);
#14239=EDGE_CURVE('',#11605,#11606,#5389,.T.);
#14240=EDGE_CURVE('',#11606,#11607,#5390,.T.);
#14241=EDGE_CURVE('',#11607,#11608,#5391,.T.);
#14242=EDGE_CURVE('',#11608,#11609,#5392,.T.);
#14243=EDGE_CURVE('',#11609,#11610,#5393,.T.);
#14244=EDGE_CURVE('',#11610,#11611,#5394,.T.);
#14245=EDGE_CURVE('',#11611,#11612,#5395,.T.);
#14246=EDGE_CURVE('',#11612,#11613,#5396,.T.);
#14247=EDGE_CURVE('',#11613,#11614,#5397,.T.);
#14248=EDGE_CURVE('',#11614,#11615,#5398,.T.);
#14249=EDGE_CURVE('',#11615,#11412,#5399,.T.);
#14250=EDGE_CURVE('',#11616,#11411,#5400,.T.);
#14251=EDGE_CURVE('',#11616,#11617,#5401,.T.);
#14252=EDGE_CURVE('',#11617,#11618,#5402,.T.);
#14253=EDGE_CURVE('',#11619,#11618,#5403,.T.);
#14254=EDGE_CURVE('',#11619,#11620,#5404,.T.);
#14255=EDGE_CURVE('',#11620,#11621,#5405,.T.);
#14256=EDGE_CURVE('',#11621,#11622,#5406,.T.);
#14257=EDGE_CURVE('',#11622,#11623,#5407,.T.);
#14258=EDGE_CURVE('',#11623,#11624,#5408,.T.);
#14259=EDGE_CURVE('',#11624,#11625,#5409,.T.);
#14260=EDGE_CURVE('',#11625,#11626,#5410,.T.);
#14261=EDGE_CURVE('',#11626,#11627,#5411,.T.);
#14262=EDGE_CURVE('',#11627,#11628,#5412,.T.);
#14263=EDGE_CURVE('',#11628,#11629,#5413,.T.);
#14264=EDGE_CURVE('',#11629,#11630,#5414,.T.);
#14265=EDGE_CURVE('',#11630,#11631,#5415,.T.);
#14266=EDGE_CURVE('',#11631,#11632,#5416,.T.);
#14267=EDGE_CURVE('',#11632,#11633,#5417,.T.);
#14268=EDGE_CURVE('',#11633,#11420,#5418,.T.);
#14269=EDGE_CURVE('',#11634,#11419,#5419,.T.);
#14270=EDGE_CURVE('',#11634,#11635,#5420,.T.);
#14271=EDGE_CURVE('',#11635,#11636,#5421,.T.);
#14272=EDGE_CURVE('',#11637,#11636,#5422,.T.);
#14273=EDGE_CURVE('',#11637,#11638,#5423,.T.);
#14274=EDGE_CURVE('',#11638,#11639,#5424,.T.);
#14275=EDGE_CURVE('',#11639,#11640,#5425,.T.);
#14276=EDGE_CURVE('',#11640,#11641,#5426,.T.);
#14277=EDGE_CURVE('',#11641,#11642,#5427,.T.);
#14278=EDGE_CURVE('',#11642,#11643,#5428,.T.);
#14279=EDGE_CURVE('',#11643,#11644,#5429,.T.);
#14280=EDGE_CURVE('',#11644,#11645,#5430,.T.);
#14281=EDGE_CURVE('',#11645,#11646,#5431,.T.);
#14282=EDGE_CURVE('',#11646,#11647,#5432,.T.);
#14283=EDGE_CURVE('',#11647,#11648,#5433,.T.);
#14284=EDGE_CURVE('',#11648,#11649,#5434,.T.);
#14285=EDGE_CURVE('',#11649,#11650,#5435,.T.);
#14286=EDGE_CURVE('',#11650,#11651,#5436,.T.);
#14287=EDGE_CURVE('',#11651,#11428,#5437,.T.);
#14288=EDGE_CURVE('',#11652,#11427,#5438,.T.);
#14289=EDGE_CURVE('',#11652,#11653,#5439,.T.);
#14290=EDGE_CURVE('',#11653,#11654,#5440,.T.);
#14291=EDGE_CURVE('',#11655,#11654,#5441,.T.);
#14292=EDGE_CURVE('',#11655,#11656,#5442,.T.);
#14293=EDGE_CURVE('',#11656,#11657,#5443,.T.);
#14294=EDGE_CURVE('',#11657,#11658,#5444,.T.);
#14295=EDGE_CURVE('',#11658,#11659,#5445,.T.);
#14296=EDGE_CURVE('',#11659,#11660,#5446,.T.);
#14297=EDGE_CURVE('',#11660,#11661,#5447,.T.);
#14298=EDGE_CURVE('',#11661,#11662,#5448,.T.);
#14299=EDGE_CURVE('',#11662,#11663,#5449,.T.);
#14300=EDGE_CURVE('',#11663,#11664,#5450,.T.);
#14301=EDGE_CURVE('',#11664,#11665,#5451,.T.);
#14302=EDGE_CURVE('',#11665,#11666,#5452,.T.);
#14303=EDGE_CURVE('',#11666,#11667,#5453,.T.);
#14304=EDGE_CURVE('',#11667,#11668,#5454,.T.);
#14305=EDGE_CURVE('',#11668,#11669,#5455,.T.);
#14306=EDGE_CURVE('',#11669,#11436,#5456,.T.);
#14307=EDGE_CURVE('',#11670,#11435,#5457,.T.);
#14308=EDGE_CURVE('',#11670,#11671,#5458,.T.);
#14309=EDGE_CURVE('',#11671,#11672,#5459,.T.);
#14310=EDGE_CURVE('',#11673,#11672,#5460,.T.);
#14311=EDGE_CURVE('',#11673,#11674,#5461,.T.);
#14312=EDGE_CURVE('',#11674,#11675,#5462,.T.);
#14313=EDGE_CURVE('',#11675,#11676,#5463,.T.);
#14314=EDGE_CURVE('',#11676,#11677,#5464,.T.);
#14315=EDGE_CURVE('',#11677,#11678,#5465,.T.);
#14316=EDGE_CURVE('',#11678,#11679,#5466,.T.);
#14317=EDGE_CURVE('',#11679,#11680,#5467,.T.);
#14318=EDGE_CURVE('',#11680,#11681,#5468,.T.);
#14319=EDGE_CURVE('',#11681,#11682,#5469,.T.);
#14320=EDGE_CURVE('',#11682,#11683,#5470,.T.);
#14321=EDGE_CURVE('',#11683,#11684,#5471,.T.);
#14322=EDGE_CURVE('',#11684,#11685,#5472,.T.);
#14323=EDGE_CURVE('',#11685,#11686,#5473,.T.);
#14324=EDGE_CURVE('',#11686,#11687,#5474,.T.);
#14325=EDGE_CURVE('',#11687,#11444,#5475,.T.);
#14326=EDGE_CURVE('',#11688,#11443,#5476,.T.);
#14327=EDGE_CURVE('',#11688,#11689,#5477,.T.);
#14328=EDGE_CURVE('',#11689,#11690,#5478,.T.);
#14329=EDGE_CURVE('',#11691,#11690,#5479,.T.);
#14330=EDGE_CURVE('',#11691,#11692,#5480,.T.);
#14331=EDGE_CURVE('',#11692,#11693,#5481,.T.);
#14332=EDGE_CURVE('',#11693,#11694,#5482,.T.);
#14333=EDGE_CURVE('',#11694,#11695,#5483,.T.);
#14334=EDGE_CURVE('',#11695,#11696,#5484,.T.);
#14335=EDGE_CURVE('',#11696,#11697,#5485,.T.);
#14336=EDGE_CURVE('',#11697,#11698,#5486,.T.);
#14337=EDGE_CURVE('',#11698,#11699,#5487,.T.);
#14338=EDGE_CURVE('',#11699,#11700,#5488,.T.);
#14339=EDGE_CURVE('',#11700,#11701,#5489,.T.);
#14340=EDGE_CURVE('',#11701,#11702,#5490,.T.);
#14341=EDGE_CURVE('',#11702,#11703,#5491,.T.);
#14342=EDGE_CURVE('',#11703,#11704,#5492,.T.);
#14343=EDGE_CURVE('',#11704,#11705,#5493,.T.);
#14344=EDGE_CURVE('',#11705,#11452,#5494,.T.);
#14345=EDGE_CURVE('',#11706,#11451,#5495,.T.);
#14346=EDGE_CURVE('',#11706,#11707,#5496,.T.);
#14347=EDGE_CURVE('',#11707,#11708,#5497,.T.);
#14348=EDGE_CURVE('',#11709,#11708,#5498,.T.);
#14349=EDGE_CURVE('',#11709,#11710,#5499,.T.);
#14350=EDGE_CURVE('',#11710,#11711,#5500,.T.);
#14351=EDGE_CURVE('',#11711,#11712,#5501,.T.);
#14352=EDGE_CURVE('',#11712,#11713,#5502,.T.);
#14353=EDGE_CURVE('',#11713,#11714,#5503,.T.);
#14354=EDGE_CURVE('',#11714,#11715,#5504,.T.);
#14355=EDGE_CURVE('',#11715,#11716,#5505,.T.);
#14356=EDGE_CURVE('',#11716,#11717,#5506,.T.);
#14357=EDGE_CURVE('',#11717,#11718,#5507,.T.);
#14358=EDGE_CURVE('',#11718,#11719,#5508,.T.);
#14359=EDGE_CURVE('',#11719,#11720,#5509,.T.);
#14360=EDGE_CURVE('',#11720,#11721,#5510,.T.);
#14361=EDGE_CURVE('',#11721,#11722,#5511,.T.);
#14362=EDGE_CURVE('',#11722,#11723,#5512,.T.);
#14363=EDGE_CURVE('',#11723,#11460,#5513,.T.);
#14364=EDGE_CURVE('',#11724,#11459,#5514,.T.);
#14365=EDGE_CURVE('',#11724,#11725,#5515,.T.);
#14366=EDGE_CURVE('',#11725,#11726,#5516,.T.);
#14367=EDGE_CURVE('',#11727,#11726,#5517,.T.);
#14368=EDGE_CURVE('',#11727,#11728,#5518,.T.);
#14369=EDGE_CURVE('',#11728,#11729,#5519,.T.);
#14370=EDGE_CURVE('',#11729,#11730,#5520,.T.);
#14371=EDGE_CURVE('',#11730,#11731,#5521,.T.);
#14372=EDGE_CURVE('',#11731,#11732,#5522,.T.);
#14373=EDGE_CURVE('',#11732,#11733,#5523,.T.);
#14374=EDGE_CURVE('',#11733,#11734,#5524,.T.);
#14375=EDGE_CURVE('',#11734,#11735,#5525,.T.);
#14376=EDGE_CURVE('',#11735,#11736,#5526,.T.);
#14377=EDGE_CURVE('',#11736,#11737,#5527,.T.);
#14378=EDGE_CURVE('',#11737,#11738,#5528,.T.);
#14379=EDGE_CURVE('',#11738,#11739,#5529,.T.);
#14380=EDGE_CURVE('',#11739,#11740,#5530,.T.);
#14381=EDGE_CURVE('',#11740,#11741,#5531,.T.);
#14382=EDGE_CURVE('',#11741,#11468,#5532,.T.);
#14383=EDGE_CURVE('',#11742,#11467,#5533,.T.);
#14384=EDGE_CURVE('',#11742,#11743,#5534,.T.);
#14385=EDGE_CURVE('',#11743,#11744,#5535,.T.);
#14386=EDGE_CURVE('',#11745,#11744,#5536,.T.);
#14387=EDGE_CURVE('',#11745,#11746,#5537,.T.);
#14388=EDGE_CURVE('',#11746,#11747,#5538,.T.);
#14389=EDGE_CURVE('',#11747,#11748,#5539,.T.);
#14390=EDGE_CURVE('',#11748,#11749,#5540,.T.);
#14391=EDGE_CURVE('',#11749,#11750,#5541,.T.);
#14392=EDGE_CURVE('',#11750,#11751,#5542,.T.);
#14393=EDGE_CURVE('',#11751,#11752,#5543,.T.);
#14394=EDGE_CURVE('',#11752,#11753,#5544,.T.);
#14395=EDGE_CURVE('',#11753,#11754,#5545,.T.);
#14396=EDGE_CURVE('',#11754,#11755,#5546,.T.);
#14397=EDGE_CURVE('',#11755,#11756,#5547,.T.);
#14398=EDGE_CURVE('',#11756,#11757,#5548,.T.);
#14399=EDGE_CURVE('',#11757,#11758,#5549,.T.);
#14400=EDGE_CURVE('',#11758,#11759,#5550,.T.);
#14401=EDGE_CURVE('',#11759,#11476,#5551,.T.);
#14402=EDGE_CURVE('',#11760,#11475,#5552,.T.);
#14403=EDGE_CURVE('',#11760,#11761,#5553,.T.);
#14404=EDGE_CURVE('',#11761,#11762,#5554,.T.);
#14405=EDGE_CURVE('',#11763,#11762,#5555,.T.);
#14406=EDGE_CURVE('',#11763,#11764,#5556,.T.);
#14407=EDGE_CURVE('',#11764,#11765,#5557,.T.);
#14408=EDGE_CURVE('',#11765,#11766,#5558,.T.);
#14409=EDGE_CURVE('',#11766,#11767,#5559,.T.);
#14410=EDGE_CURVE('',#11767,#11768,#5560,.T.);
#14411=EDGE_CURVE('',#11768,#11769,#5561,.T.);
#14412=EDGE_CURVE('',#11769,#11770,#5562,.T.);
#14413=EDGE_CURVE('',#11770,#11771,#5563,.T.);
#14414=EDGE_CURVE('',#11771,#11772,#5564,.T.);
#14415=EDGE_CURVE('',#11772,#11773,#5565,.T.);
#14416=EDGE_CURVE('',#11773,#11774,#5566,.T.);
#14417=EDGE_CURVE('',#11774,#11775,#5567,.T.);
#14418=EDGE_CURVE('',#11775,#11776,#5568,.T.);
#14419=EDGE_CURVE('',#11776,#11777,#5569,.T.);
#14420=EDGE_CURVE('',#11777,#11484,#5570,.T.);
#14421=EDGE_CURVE('',#11778,#11483,#5571,.T.);
#14422=EDGE_CURVE('',#11778,#11779,#5572,.T.);
#14423=EDGE_CURVE('',#11779,#11780,#5573,.T.);
#14424=EDGE_CURVE('',#11781,#11780,#5574,.T.);
#14425=EDGE_CURVE('',#11781,#11782,#5575,.T.);
#14426=EDGE_CURVE('',#11782,#11783,#5576,.T.);
#14427=EDGE_CURVE('',#11783,#11784,#5577,.T.);
#14428=EDGE_CURVE('',#11784,#11785,#5578,.T.);
#14429=EDGE_CURVE('',#11785,#11786,#5579,.T.);
#14430=EDGE_CURVE('',#11786,#11787,#5580,.T.);
#14431=EDGE_CURVE('',#11787,#11788,#5581,.T.);
#14432=EDGE_CURVE('',#11788,#11789,#5582,.T.);
#14433=EDGE_CURVE('',#11789,#11790,#5583,.T.);
#14434=EDGE_CURVE('',#11790,#11791,#5584,.T.);
#14435=EDGE_CURVE('',#11791,#11792,#5585,.T.);
#14436=EDGE_CURVE('',#11792,#11793,#5586,.T.);
#14437=EDGE_CURVE('',#11793,#11794,#5587,.T.);
#14438=EDGE_CURVE('',#11794,#11795,#5588,.T.);
#14439=EDGE_CURVE('',#11795,#11492,#5589,.T.);
#14440=EDGE_CURVE('',#11796,#11796,#10569,.T.);
#14441=EDGE_CURVE('',#11797,#11781,#5590,.T.);
#14442=EDGE_CURVE('',#11780,#11576,#5591,.F.);
#14443=EDGE_CURVE('',#11577,#11797,#5592,.T.);
#14444=EDGE_CURVE('',#11485,#11798,#5593,.T.);
#14445=EDGE_CURVE('',#11798,#11799,#5594,.T.);
#14446=EDGE_CURVE('',#11799,#11778,#5595,.F.);
#14447=EDGE_CURVE('',#11800,#11763,#5596,.T.);
#14448=EDGE_CURVE('',#11762,#11569,#5597,.F.);
#14449=EDGE_CURVE('',#11570,#11800,#5598,.T.);
#14450=EDGE_CURVE('',#11477,#11801,#5599,.T.);
#14451=EDGE_CURVE('',#11801,#11802,#5600,.T.);
#14452=EDGE_CURVE('',#11802,#11760,#5601,.F.);
#14453=EDGE_CURVE('',#11803,#11745,#5602,.T.);
#14454=EDGE_CURVE('',#11744,#11562,#5603,.F.);
#14455=EDGE_CURVE('',#11563,#11803,#5604,.T.);
#14456=EDGE_CURVE('',#11469,#11804,#5605,.T.);
#14457=EDGE_CURVE('',#11804,#11805,#5606,.T.);
#14458=EDGE_CURVE('',#11805,#11742,#5607,.F.);
#14459=EDGE_CURVE('',#11806,#11727,#5608,.T.);
#14460=EDGE_CURVE('',#11726,#11555,#5609,.F.);
#14461=EDGE_CURVE('',#11556,#11806,#5610,.T.);
#14462=EDGE_CURVE('',#11461,#11807,#5611,.T.);
#14463=EDGE_CURVE('',#11807,#11808,#5612,.T.);
#14464=EDGE_CURVE('',#11808,#11724,#5613,.F.);
#14465=EDGE_CURVE('',#11809,#11709,#5614,.T.);
#14466=EDGE_CURVE('',#11708,#11548,#5615,.F.);
#14467=EDGE_CURVE('',#11549,#11809,#5616,.T.);
#14468=EDGE_CURVE('',#11453,#11810,#5617,.T.);
#14469=EDGE_CURVE('',#11810,#11811,#5618,.T.);
#14470=EDGE_CURVE('',#11811,#11706,#5619,.F.);
#14471=EDGE_CURVE('',#11812,#11691,#5620,.T.);
#14472=EDGE_CURVE('',#11690,#11541,#5621,.F.);
#14473=EDGE_CURVE('',#11542,#11812,#5622,.T.);
#14474=EDGE_CURVE('',#11445,#11813,#5623,.T.);
#14475=EDGE_CURVE('',#11813,#11814,#5624,.T.);
#14476=EDGE_CURVE('',#11814,#11688,#5625,.F.);
#14477=EDGE_CURVE('',#11815,#11673,#5626,.T.);
#14478=EDGE_CURVE('',#11672,#11534,#5627,.F.);
#14479=EDGE_CURVE('',#11535,#11815,#5628,.T.);
#14480=EDGE_CURVE('',#11437,#11816,#5629,.T.);
#14481=EDGE_CURVE('',#11816,#11817,#5630,.T.);
#14482=EDGE_CURVE('',#11817,#11670,#5631,.F.);
#14483=EDGE_CURVE('',#11818,#11655,#5632,.T.);
#14484=EDGE_CURVE('',#11654,#11527,#5633,.F.);
#14485=EDGE_CURVE('',#11528,#11818,#5634,.T.);
#14486=EDGE_CURVE('',#11429,#11819,#5635,.T.);
#14487=EDGE_CURVE('',#11819,#11820,#5636,.T.);
#14488=EDGE_CURVE('',#11820,#11652,#5637,.F.);
#14489=EDGE_CURVE('',#11821,#11637,#5638,.T.);
#14490=EDGE_CURVE('',#11636,#11520,#5639,.F.);
#14491=EDGE_CURVE('',#11521,#11821,#5640,.T.);
#14492=EDGE_CURVE('',#11421,#11822,#5641,.T.);
#14493=EDGE_CURVE('',#11822,#11823,#5642,.T.);
#14494=EDGE_CURVE('',#11823,#11634,#5643,.F.);
#14495=EDGE_CURVE('',#11824,#11619,#5644,.T.);
#14496=EDGE_CURVE('',#11618,#11513,#5645,.F.);
#14497=EDGE_CURVE('',#11514,#11824,#5646,.T.);
#14498=EDGE_CURVE('',#11413,#11825,#5647,.T.);
#14499=EDGE_CURVE('',#11825,#11826,#5648,.T.);
#14500=EDGE_CURVE('',#11826,#11616,#5649,.F.);
#14501=EDGE_CURVE('',#11827,#11601,#5650,.T.);
#14502=EDGE_CURVE('',#11600,#11506,#5651,.F.);
#14503=EDGE_CURVE('',#11507,#11827,#5652,.T.);
#14504=EDGE_CURVE('',#11405,#11828,#5653,.T.);
#14505=EDGE_CURVE('',#11828,#11829,#5654,.T.);
#14506=EDGE_CURVE('',#11829,#11598,#5655,.F.);
#14507=EDGE_CURVE('',#11830,#11583,#5656,.T.);
#14508=EDGE_CURVE('',#11582,#11499,#5657,.F.);
#14509=EDGE_CURVE('',#11500,#11830,#5658,.T.);
#14510=EDGE_CURVE('',#11831,#11832,#10570,.T.);
#14511=EDGE_CURVE('',#11831,#11833,#5659,.T.);
#14512=EDGE_CURVE('',#11833,#11834,#5660,.T.);
#14513=EDGE_CURVE('',#11832,#11834,#5661,.T.);
#14514=EDGE_CURVE('',#11832,#11835,#5662,.T.);
#14515=EDGE_CURVE('',#11834,#11836,#5663,.T.);
#14516=EDGE_CURVE('',#11835,#11836,#5664,.T.);
#14517=EDGE_CURVE('',#11837,#11831,#5665,.T.);
#14518=EDGE_CURVE('',#11837,#11838,#5666,.T.);
#14519=EDGE_CURVE('',#11838,#11833,#5667,.T.);
#14520=EDGE_CURVE('',#11835,#11837,#10571,.T.);
#14521=EDGE_CURVE('',#11836,#11838,#5668,.T.);
#14522=EDGE_CURVE('',#11181,#11581,#5669,.T.);
#14523=EDGE_CURVE('',#11487,#11579,#5670,.T.);
#14524=EDGE_CURVE('',#11488,#11578,#5671,.T.);
#14525=EDGE_CURVE('',#11185,#11795,#5672,.T.);
#14526=EDGE_CURVE('',#11186,#11794,#5673,.T.);
#14527=EDGE_CURVE('',#11187,#11793,#5674,.T.);
#14528=EDGE_CURVE('',#11188,#11792,#5675,.T.);
#14529=EDGE_CURVE('',#11189,#11791,#5676,.T.);
#14530=EDGE_CURVE('',#11190,#11790,#5677,.T.);
#14531=EDGE_CURVE('',#11191,#11789,#5678,.T.);
#14532=EDGE_CURVE('',#11192,#11788,#5679,.T.);
#14533=EDGE_CURVE('',#11193,#11787,#5680,.T.);
#14534=EDGE_CURVE('',#11194,#11786,#5681,.T.);
#14535=EDGE_CURVE('',#11195,#11785,#5682,.T.);
#14536=EDGE_CURVE('',#11196,#11784,#5683,.T.);
#14537=EDGE_CURVE('',#11197,#11783,#5684,.T.);
#14538=EDGE_CURVE('',#11198,#11782,#5685,.T.);
#14539=EDGE_CURVE('',#11574,#11797,#5686,.T.);
#14540=EDGE_CURVE('',#11201,#11779,#5687,.T.);
#14541=EDGE_CURVE('',#11479,#11799,#5688,.T.);
#14542=EDGE_CURVE('',#11480,#11798,#5689,.T.);
#14543=EDGE_CURVE('',#11205,#11777,#5690,.T.);
#14544=EDGE_CURVE('',#11206,#11776,#5691,.T.);
#14545=EDGE_CURVE('',#11207,#11775,#5692,.T.);
#14546=EDGE_CURVE('',#11208,#11774,#5693,.T.);
#14547=EDGE_CURVE('',#11209,#11773,#5694,.T.);
#14548=EDGE_CURVE('',#11210,#11772,#5695,.T.);
#14549=EDGE_CURVE('',#11211,#11771,#5696,.T.);
#14550=EDGE_CURVE('',#11212,#11770,#5697,.T.);
#14551=EDGE_CURVE('',#11213,#11769,#5698,.T.);
#14552=EDGE_CURVE('',#11214,#11768,#5699,.T.);
#14553=EDGE_CURVE('',#11215,#11767,#5700,.T.);
#14554=EDGE_CURVE('',#11216,#11766,#5701,.T.);
#14555=EDGE_CURVE('',#11217,#11765,#5702,.T.);
#14556=EDGE_CURVE('',#11218,#11764,#5703,.T.);
#14557=EDGE_CURVE('',#11567,#11800,#5704,.T.);
#14558=EDGE_CURVE('',#11221,#11761,#5705,.T.);
#14559=EDGE_CURVE('',#11471,#11802,#5706,.T.);
#14560=EDGE_CURVE('',#11472,#11801,#5707,.T.);
#14561=EDGE_CURVE('',#11225,#11759,#5708,.T.);
#14562=EDGE_CURVE('',#11226,#11758,#5709,.T.);
#14563=EDGE_CURVE('',#11227,#11757,#5710,.T.);
#14564=EDGE_CURVE('',#11228,#11756,#5711,.T.);
#14565=EDGE_CURVE('',#11229,#11755,#5712,.T.);
#14566=EDGE_CURVE('',#11230,#11754,#5713,.T.);
#14567=EDGE_CURVE('',#11231,#11753,#5714,.T.);
#14568=EDGE_CURVE('',#11232,#11752,#5715,.T.);
#14569=EDGE_CURVE('',#11233,#11751,#5716,.T.);
#14570=EDGE_CURVE('',#11234,#11750,#5717,.T.);
#14571=EDGE_CURVE('',#11235,#11749,#5718,.T.);
#14572=EDGE_CURVE('',#11236,#11748,#5719,.T.);
#14573=EDGE_CURVE('',#11237,#11747,#5720,.T.);
#14574=EDGE_CURVE('',#11238,#11746,#5721,.T.);
#14575=EDGE_CURVE('',#11560,#11803,#5722,.T.);
#14576=EDGE_CURVE('',#11241,#11743,#5723,.T.);
#14577=EDGE_CURVE('',#11463,#11805,#5724,.T.);
#14578=EDGE_CURVE('',#11464,#11804,#5725,.T.);
#14579=EDGE_CURVE('',#11245,#11741,#5726,.T.);
#14580=EDGE_CURVE('',#11246,#11740,#5727,.T.);
#14581=EDGE_CURVE('',#11247,#11739,#5728,.T.);
#14582=EDGE_CURVE('',#11248,#11738,#5729,.T.);
#14583=EDGE_CURVE('',#11249,#11737,#5730,.T.);
#14584=EDGE_CURVE('',#11250,#11736,#5731,.T.);
#14585=EDGE_CURVE('',#11251,#11735,#5732,.T.);
#14586=EDGE_CURVE('',#11252,#11734,#5733,.T.);
#14587=EDGE_CURVE('',#11253,#11733,#5734,.T.);
#14588=EDGE_CURVE('',#11254,#11732,#5735,.T.);
#14589=EDGE_CURVE('',#11255,#11731,#5736,.T.);
#14590=EDGE_CURVE('',#11256,#11730,#5737,.T.);
#14591=EDGE_CURVE('',#11257,#11729,#5738,.T.);
#14592=EDGE_CURVE('',#11258,#11728,#5739,.T.);
#14593=EDGE_CURVE('',#11553,#11806,#5740,.T.);
#14594=EDGE_CURVE('',#11261,#11725,#5741,.T.);
#14595=EDGE_CURVE('',#11455,#11808,#5742,.T.);
#14596=EDGE_CURVE('',#11456,#11807,#5743,.T.);
#14597=EDGE_CURVE('',#11265,#11723,#5744,.T.);
#14598=EDGE_CURVE('',#11266,#11722,#5745,.T.);
#14599=EDGE_CURVE('',#11267,#11721,#5746,.T.);
#14600=EDGE_CURVE('',#11268,#11720,#5747,.T.);
#14601=EDGE_CURVE('',#11269,#11719,#5748,.T.);
#14602=EDGE_CURVE('',#11270,#11718,#5749,.T.);
#14603=EDGE_CURVE('',#11271,#11717,#5750,.T.);
#14604=EDGE_CURVE('',#11272,#11716,#5751,.T.);
#14605=EDGE_CURVE('',#11273,#11715,#5752,.T.);
#14606=EDGE_CURVE('',#11274,#11714,#5753,.T.);
#14607=EDGE_CURVE('',#11275,#11713,#5754,.T.);
#14608=EDGE_CURVE('',#11276,#11712,#5755,.T.);
#14609=EDGE_CURVE('',#11277,#11711,#5756,.T.);
#14610=EDGE_CURVE('',#11278,#11710,#5757,.T.);
#14611=EDGE_CURVE('',#11546,#11809,#5758,.T.);
#14612=EDGE_CURVE('',#11281,#11707,#5759,.T.);
#14613=EDGE_CURVE('',#11447,#11811,#5760,.T.);
#14614=EDGE_CURVE('',#11448,#11810,#5761,.T.);
#14615=EDGE_CURVE('',#11285,#11705,#5762,.T.);
#14616=EDGE_CURVE('',#11286,#11704,#5763,.T.);
#14617=EDGE_CURVE('',#11287,#11703,#5764,.T.);
#14618=EDGE_CURVE('',#11288,#11702,#5765,.T.);
#14619=EDGE_CURVE('',#11289,#11701,#5766,.T.);
#14620=EDGE_CURVE('',#11290,#11700,#5767,.T.);
#14621=EDGE_CURVE('',#11291,#11699,#5768,.T.);
#14622=EDGE_CURVE('',#11292,#11698,#5769,.T.);
#14623=EDGE_CURVE('',#11293,#11697,#5770,.T.);
#14624=EDGE_CURVE('',#11294,#11696,#5771,.T.);
#14625=EDGE_CURVE('',#11295,#11695,#5772,.T.);
#14626=EDGE_CURVE('',#11296,#11694,#5773,.T.);
#14627=EDGE_CURVE('',#11297,#11693,#5774,.T.);
#14628=EDGE_CURVE('',#11298,#11692,#5775,.T.);
#14629=EDGE_CURVE('',#11539,#11812,#5776,.T.);
#14630=EDGE_CURVE('',#11301,#11689,#5777,.T.);
#14631=EDGE_CURVE('',#11439,#11814,#5778,.T.);
#14632=EDGE_CURVE('',#11440,#11813,#5779,.T.);
#14633=EDGE_CURVE('',#11305,#11687,#5780,.T.);
#14634=EDGE_CURVE('',#11306,#11686,#5781,.T.);
#14635=EDGE_CURVE('',#11307,#11685,#5782,.T.);
#14636=EDGE_CURVE('',#11308,#11684,#5783,.T.);
#14637=EDGE_CURVE('',#11309,#11683,#5784,.T.);
#14638=EDGE_CURVE('',#11310,#11682,#5785,.T.);
#14639=EDGE_CURVE('',#11311,#11681,#5786,.T.);
#14640=EDGE_CURVE('',#11312,#11680,#5787,.T.);
#14641=EDGE_CURVE('',#11313,#11679,#5788,.T.);
#14642=EDGE_CURVE('',#11314,#11678,#5789,.T.);
#14643=EDGE_CURVE('',#11315,#11677,#5790,.T.);
#14644=EDGE_CURVE('',#11316,#11676,#5791,.T.);
#14645=EDGE_CURVE('',#11317,#11675,#5792,.T.);
#14646=EDGE_CURVE('',#11318,#11674,#5793,.T.);
#14647=EDGE_CURVE('',#11532,#11815,#5794,.T.);
#14648=EDGE_CURVE('',#11321,#11671,#5795,.T.);
#14649=EDGE_CURVE('',#11431,#11817,#5796,.T.);
#14650=EDGE_CURVE('',#11432,#11816,#5797,.T.);
#14651=EDGE_CURVE('',#11325,#11669,#5798,.T.);
#14652=EDGE_CURVE('',#11326,#11668,#5799,.T.);
#14653=EDGE_CURVE('',#11327,#11667,#5800,.T.);
#14654=EDGE_CURVE('',#11328,#11666,#5801,.T.);
#14655=EDGE_CURVE('',#11329,#11665,#5802,.T.);
#14656=EDGE_CURVE('',#11330,#11664,#5803,.T.);
#14657=EDGE_CURVE('',#11331,#11663,#5804,.T.);
#14658=EDGE_CURVE('',#11332,#11662,#5805,.T.);
#14659=EDGE_CURVE('',#11333,#11661,#5806,.T.);
#14660=EDGE_CURVE('',#11334,#11660,#5807,.T.);
#14661=EDGE_CURVE('',#11335,#11659,#5808,.T.);
#14662=EDGE_CURVE('',#11336,#11658,#5809,.T.);
#14663=EDGE_CURVE('',#11337,#11657,#5810,.T.);
#14664=EDGE_CURVE('',#11338,#11656,#5811,.T.);
#14665=EDGE_CURVE('',#11525,#11818,#5812,.T.);
#14666=EDGE_CURVE('',#11341,#11653,#5813,.T.);
#14667=EDGE_CURVE('',#11423,#11820,#5814,.T.);
#14668=EDGE_CURVE('',#11424,#11819,#5815,.T.);
#14669=EDGE_CURVE('',#11345,#11651,#5816,.T.);
#14670=EDGE_CURVE('',#11346,#11650,#5817,.T.);
#14671=EDGE_CURVE('',#11347,#11649,#5818,.T.);
#14672=EDGE_CURVE('',#11348,#11648,#5819,.T.);
#14673=EDGE_CURVE('',#11349,#11647,#5820,.T.);
#14674=EDGE_CURVE('',#11350,#11646,#5821,.T.);
#14675=EDGE_CURVE('',#11351,#11645,#5822,.T.);
#14676=EDGE_CURVE('',#11352,#11644,#5823,.T.);
#14677=EDGE_CURVE('',#11353,#11643,#5824,.T.);
#14678=EDGE_CURVE('',#11354,#11642,#5825,.T.);
#14679=EDGE_CURVE('',#11355,#11641,#5826,.T.);
#14680=EDGE_CURVE('',#11356,#11640,#5827,.T.);
#14681=EDGE_CURVE('',#11357,#11639,#5828,.T.);
#14682=EDGE_CURVE('',#11358,#11638,#5829,.T.);
#14683=EDGE_CURVE('',#11518,#11821,#5830,.T.);
#14684=EDGE_CURVE('',#11361,#11635,#5831,.T.);
#14685=EDGE_CURVE('',#11415,#11823,#5832,.T.);
#14686=EDGE_CURVE('',#11416,#11822,#5833,.T.);
#14687=EDGE_CURVE('',#11365,#11633,#5834,.T.);
#14688=EDGE_CURVE('',#11366,#11632,#5835,.T.);
#14689=EDGE_CURVE('',#11367,#11631,#5836,.T.);
#14690=EDGE_CURVE('',#11368,#11630,#5837,.T.);
#14691=EDGE_CURVE('',#11369,#11629,#5838,.T.);
#14692=EDGE_CURVE('',#11370,#11628,#5839,.T.);
#14693=EDGE_CURVE('',#11371,#11627,#5840,.T.);
#14694=EDGE_CURVE('',#11372,#11626,#5841,.T.);
#14695=EDGE_CURVE('',#11373,#11625,#5842,.T.);
#14696=EDGE_CURVE('',#11374,#11624,#5843,.T.);
#14697=EDGE_CURVE('',#11375,#11623,#5844,.T.);
#14698=EDGE_CURVE('',#11376,#11622,#5845,.T.);
#14699=EDGE_CURVE('',#11377,#11621,#5846,.T.);
#14700=EDGE_CURVE('',#11378,#11620,#5847,.T.);
#14701=EDGE_CURVE('',#11511,#11824,#5848,.T.);
#14702=EDGE_CURVE('',#11381,#11617,#5849,.T.);
#14703=EDGE_CURVE('',#11407,#11826,#5850,.T.);
#14704=EDGE_CURVE('',#11408,#11825,#5851,.T.);
#14705=EDGE_CURVE('',#11385,#11615,#5852,.T.);
#14706=EDGE_CURVE('',#11386,#11614,#5853,.T.);
#14707=EDGE_CURVE('',#11387,#11613,#5854,.T.);
#14708=EDGE_CURVE('',#11388,#11612,#5855,.T.);
#14709=EDGE_CURVE('',#11389,#11611,#5856,.T.);
#14710=EDGE_CURVE('',#11390,#11610,#5857,.T.);
#14711=EDGE_CURVE('',#11391,#11609,#5858,.T.);
#14712=EDGE_CURVE('',#11392,#11608,#5859,.T.);
#14713=EDGE_CURVE('',#11393,#11607,#5860,.T.);
#14714=EDGE_CURVE('',#11394,#11606,#5861,.T.);
#14715=EDGE_CURVE('',#11395,#11605,#5862,.T.);
#14716=EDGE_CURVE('',#11396,#11604,#5863,.T.);
#14717=EDGE_CURVE('',#11397,#11603,#5864,.T.);
#14718=EDGE_CURVE('',#11398,#11602,#5865,.T.);
#14719=EDGE_CURVE('',#11504,#11827,#5866,.T.);
#14720=EDGE_CURVE('',#11163,#11599,#5867,.T.);
#14721=EDGE_CURVE('',#11160,#11829,#5868,.T.);
#14722=EDGE_CURVE('',#11161,#11828,#5869,.T.);
#14723=EDGE_CURVE('',#11165,#11597,#5870,.T.);
#14724=EDGE_CURVE('',#11166,#11596,#5871,.T.);
#14725=EDGE_CURVE('',#11167,#11595,#5872,.T.);
#14726=EDGE_CURVE('',#11168,#11594,#5873,.T.);
#14727=EDGE_CURVE('',#11169,#11593,#5874,.T.);
#14728=EDGE_CURVE('',#11170,#11592,#5875,.T.);
#14729=EDGE_CURVE('',#11171,#11591,#5876,.T.);
#14730=EDGE_CURVE('',#11172,#11590,#5877,.T.);
#14731=EDGE_CURVE('',#11173,#11589,#5878,.T.);
#14732=EDGE_CURVE('',#11174,#11588,#5879,.T.);
#14733=EDGE_CURVE('',#11175,#11587,#5880,.T.);
#14734=EDGE_CURVE('',#11176,#11586,#5881,.T.);
#14735=EDGE_CURVE('',#11177,#11585,#5882,.T.);
#14736=EDGE_CURVE('',#11178,#11584,#5883,.T.);
#14737=EDGE_CURVE('',#11497,#11830,#5884,.T.);
#14738=EDGE_CURVE('',#11401,#11839,#5885,.T.);
#14739=EDGE_CURVE('',#11839,#11839,#10572,.T.);
#14740=EDGE_CURVE('',#11840,#11840,#10573,.T.);
#14741=EDGE_CURVE('',#11841,#11841,#10574,.T.);
#14742=EDGE_CURVE('',#11841,#11840,#5886,.T.);
#14743=EDGE_CURVE('',#11842,#11842,#10575,.T.);
#14744=EDGE_CURVE('',#11842,#11841,#5887,.T.);
#14745=EDGE_CURVE('',#11843,#11843,#10576,.T.);
#14746=EDGE_CURVE('',#11843,#11796,#5888,.T.);
#17926=ORIENTED_EDGE('',*,*,#13716,.T.);
#17927=ORIENTED_EDGE('',*,*,#13717,.T.);
#17928=ORIENTED_EDGE('',*,*,#13718,.T.);
#17929=ORIENTED_EDGE('',*,*,#13719,.T.);
#17930=ORIENTED_EDGE('',*,*,#13720,.T.);
#17931=ORIENTED_EDGE('',*,*,#13721,.T.);
#17932=ORIENTED_EDGE('',*,*,#13722,.T.);
#17933=ORIENTED_EDGE('',*,*,#13717,.F.);
#17934=ORIENTED_EDGE('',*,*,#13723,.T.);
#17935=ORIENTED_EDGE('',*,*,#13724,.T.);
#17936=ORIENTED_EDGE('',*,*,#13725,.T.);
#17937=ORIENTED_EDGE('',*,*,#13726,.T.);
#17938=ORIENTED_EDGE('',*,*,#13727,.T.);
#17939=ORIENTED_EDGE('',*,*,#13728,.T.);
#17940=ORIENTED_EDGE('',*,*,#13729,.T.);
#17941=ORIENTED_EDGE('',*,*,#13730,.T.);
#17942=ORIENTED_EDGE('',*,*,#13731,.T.);
#17943=ORIENTED_EDGE('',*,*,#13732,.T.);
#17944=ORIENTED_EDGE('',*,*,#13733,.T.);
#17945=ORIENTED_EDGE('',*,*,#13734,.T.);
#17946=ORIENTED_EDGE('',*,*,#13735,.T.);
#17947=ORIENTED_EDGE('',*,*,#13736,.T.);
#17948=ORIENTED_EDGE('',*,*,#13737,.T.);
#17949=ORIENTED_EDGE('',*,*,#13738,.T.);
#17950=ORIENTED_EDGE('',*,*,#13739,.F.);
#17951=ORIENTED_EDGE('',*,*,#13740,.T.);
#17952=ORIENTED_EDGE('',*,*,#13741,.T.);
#17953=ORIENTED_EDGE('',*,*,#13742,.F.);
#17954=ORIENTED_EDGE('',*,*,#13743,.T.);
#17955=ORIENTED_EDGE('',*,*,#13744,.T.);
#17956=ORIENTED_EDGE('',*,*,#13745,.T.);
#17957=ORIENTED_EDGE('',*,*,#13746,.T.);
#17958=ORIENTED_EDGE('',*,*,#13747,.T.);
#17959=ORIENTED_EDGE('',*,*,#13748,.T.);
#17960=ORIENTED_EDGE('',*,*,#13749,.T.);
#17961=ORIENTED_EDGE('',*,*,#13750,.T.);
#17962=ORIENTED_EDGE('',*,*,#13751,.T.);
#17963=ORIENTED_EDGE('',*,*,#13752,.T.);
#17964=ORIENTED_EDGE('',*,*,#13753,.T.);
#17965=ORIENTED_EDGE('',*,*,#13754,.T.);
#17966=ORIENTED_EDGE('',*,*,#13755,.T.);
#17967=ORIENTED_EDGE('',*,*,#13756,.T.);
#17968=ORIENTED_EDGE('',*,*,#13757,.T.);
#17969=ORIENTED_EDGE('',*,*,#13758,.T.);
#17970=ORIENTED_EDGE('',*,*,#13759,.F.);
#17971=ORIENTED_EDGE('',*,*,#13760,.T.);
#17972=ORIENTED_EDGE('',*,*,#13761,.T.);
#17973=ORIENTED_EDGE('',*,*,#13762,.F.);
#17974=ORIENTED_EDGE('',*,*,#13763,.T.);
#17975=ORIENTED_EDGE('',*,*,#13764,.T.);
#17976=ORIENTED_EDGE('',*,*,#13765,.T.);
#17977=ORIENTED_EDGE('',*,*,#13766,.T.);
#17978=ORIENTED_EDGE('',*,*,#13767,.T.);
#17979=ORIENTED_EDGE('',*,*,#13768,.T.);
#17980=ORIENTED_EDGE('',*,*,#13769,.T.);
#17981=ORIENTED_EDGE('',*,*,#13770,.T.);
#17982=ORIENTED_EDGE('',*,*,#13771,.T.);
#17983=ORIENTED_EDGE('',*,*,#13772,.T.);
#17984=ORIENTED_EDGE('',*,*,#13773,.T.);
#17985=ORIENTED_EDGE('',*,*,#13774,.T.);
#17986=ORIENTED_EDGE('',*,*,#13775,.T.);
#17987=ORIENTED_EDGE('',*,*,#13776,.T.);
#17988=ORIENTED_EDGE('',*,*,#13777,.T.);
#17989=ORIENTED_EDGE('',*,*,#13778,.T.);
#17990=ORIENTED_EDGE('',*,*,#13779,.F.);
#17991=ORIENTED_EDGE('',*,*,#13780,.T.);
#17992=ORIENTED_EDGE('',*,*,#13781,.T.);
#17993=ORIENTED_EDGE('',*,*,#13782,.F.);
#17994=ORIENTED_EDGE('',*,*,#13783,.T.);
#17995=ORIENTED_EDGE('',*,*,#13784,.T.);
#17996=ORIENTED_EDGE('',*,*,#13785,.T.);
#17997=ORIENTED_EDGE('',*,*,#13786,.T.);
#17998=ORIENTED_EDGE('',*,*,#13787,.T.);
#17999=ORIENTED_EDGE('',*,*,#13788,.T.);
#18000=ORIENTED_EDGE('',*,*,#13789,.T.);
#18001=ORIENTED_EDGE('',*,*,#13790,.T.);
#18002=ORIENTED_EDGE('',*,*,#13791,.T.);
#18003=ORIENTED_EDGE('',*,*,#13792,.T.);
#18004=ORIENTED_EDGE('',*,*,#13793,.T.);
#18005=ORIENTED_EDGE('',*,*,#13794,.T.);
#18006=ORIENTED_EDGE('',*,*,#13795,.T.);
#18007=ORIENTED_EDGE('',*,*,#13796,.T.);
#18008=ORIENTED_EDGE('',*,*,#13797,.T.);
#18009=ORIENTED_EDGE('',*,*,#13798,.T.);
#18010=ORIENTED_EDGE('',*,*,#13799,.F.);
#18011=ORIENTED_EDGE('',*,*,#13800,.T.);
#18012=ORIENTED_EDGE('',*,*,#13801,.T.);
#18013=ORIENTED_EDGE('',*,*,#13802,.F.);
#18014=ORIENTED_EDGE('',*,*,#13803,.T.);
#18015=ORIENTED_EDGE('',*,*,#13804,.T.);
#18016=ORIENTED_EDGE('',*,*,#13805,.T.);
#18017=ORIENTED_EDGE('',*,*,#13806,.T.);
#18018=ORIENTED_EDGE('',*,*,#13807,.T.);
#18019=ORIENTED_EDGE('',*,*,#13808,.T.);
#18020=ORIENTED_EDGE('',*,*,#13809,.T.);
#18021=ORIENTED_EDGE('',*,*,#13810,.T.);
#18022=ORIENTED_EDGE('',*,*,#13811,.T.);
#18023=ORIENTED_EDGE('',*,*,#13812,.T.);
#18024=ORIENTED_EDGE('',*,*,#13813,.T.);
#18025=ORIENTED_EDGE('',*,*,#13814,.T.);
#18026=ORIENTED_EDGE('',*,*,#13815,.T.);
#18027=ORIENTED_EDGE('',*,*,#13816,.T.);
#18028=ORIENTED_EDGE('',*,*,#13817,.T.);
#18029=ORIENTED_EDGE('',*,*,#13818,.T.);
#18030=ORIENTED_EDGE('',*,*,#13819,.F.);
#18031=ORIENTED_EDGE('',*,*,#13820,.T.);
#18032=ORIENTED_EDGE('',*,*,#13821,.T.);
#18033=ORIENTED_EDGE('',*,*,#13822,.F.);
#18034=ORIENTED_EDGE('',*,*,#13823,.T.);
#18035=ORIENTED_EDGE('',*,*,#13824,.T.);
#18036=ORIENTED_EDGE('',*,*,#13825,.T.);
#18037=ORIENTED_EDGE('',*,*,#13826,.T.);
#18038=ORIENTED_EDGE('',*,*,#13827,.T.);
#18039=ORIENTED_EDGE('',*,*,#13828,.T.);
#18040=ORIENTED_EDGE('',*,*,#13829,.T.);
#18041=ORIENTED_EDGE('',*,*,#13830,.T.);
#18042=ORIENTED_EDGE('',*,*,#13831,.T.);
#18043=ORIENTED_EDGE('',*,*,#13832,.T.);
#18044=ORIENTED_EDGE('',*,*,#13833,.T.);
#18045=ORIENTED_EDGE('',*,*,#13834,.T.);
#18046=ORIENTED_EDGE('',*,*,#13835,.T.);
#18047=ORIENTED_EDGE('',*,*,#13836,.T.);
#18048=ORIENTED_EDGE('',*,*,#13837,.T.);
#18049=ORIENTED_EDGE('',*,*,#13838,.T.);
#18050=ORIENTED_EDGE('',*,*,#13839,.F.);
#18051=ORIENTED_EDGE('',*,*,#13840,.T.);
#18052=ORIENTED_EDGE('',*,*,#13841,.T.);
#18053=ORIENTED_EDGE('',*,*,#13842,.F.);
#18054=ORIENTED_EDGE('',*,*,#13843,.T.);
#18055=ORIENTED_EDGE('',*,*,#13844,.T.);
#18056=ORIENTED_EDGE('',*,*,#13845,.T.);
#18057=ORIENTED_EDGE('',*,*,#13846,.T.);
#18058=ORIENTED_EDGE('',*,*,#13847,.T.);
#18059=ORIENTED_EDGE('',*,*,#13848,.T.);
#18060=ORIENTED_EDGE('',*,*,#13849,.T.);
#18061=ORIENTED_EDGE('',*,*,#13850,.T.);
#18062=ORIENTED_EDGE('',*,*,#13851,.T.);
#18063=ORIENTED_EDGE('',*,*,#13852,.T.);
#18064=ORIENTED_EDGE('',*,*,#13853,.T.);
#18065=ORIENTED_EDGE('',*,*,#13854,.T.);
#18066=ORIENTED_EDGE('',*,*,#13855,.T.);
#18067=ORIENTED_EDGE('',*,*,#13856,.T.);
#18068=ORIENTED_EDGE('',*,*,#13857,.T.);
#18069=ORIENTED_EDGE('',*,*,#13858,.T.);
#18070=ORIENTED_EDGE('',*,*,#13859,.F.);
#18071=ORIENTED_EDGE('',*,*,#13860,.T.);
#18072=ORIENTED_EDGE('',*,*,#13861,.T.);
#18073=ORIENTED_EDGE('',*,*,#13862,.F.);
#18074=ORIENTED_EDGE('',*,*,#13863,.T.);
#18075=ORIENTED_EDGE('',*,*,#13864,.T.);
#18076=ORIENTED_EDGE('',*,*,#13865,.T.);
#18077=ORIENTED_EDGE('',*,*,#13866,.T.);
#18078=ORIENTED_EDGE('',*,*,#13867,.T.);
#18079=ORIENTED_EDGE('',*,*,#13868,.T.);
#18080=ORIENTED_EDGE('',*,*,#13869,.T.);
#18081=ORIENTED_EDGE('',*,*,#13870,.T.);
#18082=ORIENTED_EDGE('',*,*,#13871,.T.);
#18083=ORIENTED_EDGE('',*,*,#13872,.T.);
#18084=ORIENTED_EDGE('',*,*,#13873,.T.);
#18085=ORIENTED_EDGE('',*,*,#13874,.T.);
#18086=ORIENTED_EDGE('',*,*,#13875,.T.);
#18087=ORIENTED_EDGE('',*,*,#13876,.T.);
#18088=ORIENTED_EDGE('',*,*,#13877,.T.);
#18089=ORIENTED_EDGE('',*,*,#13878,.T.);
#18090=ORIENTED_EDGE('',*,*,#13879,.F.);
#18091=ORIENTED_EDGE('',*,*,#13880,.T.);
#18092=ORIENTED_EDGE('',*,*,#13881,.T.);
#18093=ORIENTED_EDGE('',*,*,#13882,.F.);
#18094=ORIENTED_EDGE('',*,*,#13883,.T.);
#18095=ORIENTED_EDGE('',*,*,#13884,.T.);
#18096=ORIENTED_EDGE('',*,*,#13885,.T.);
#18097=ORIENTED_EDGE('',*,*,#13886,.T.);
#18098=ORIENTED_EDGE('',*,*,#13887,.T.);
#18099=ORIENTED_EDGE('',*,*,#13888,.T.);
#18100=ORIENTED_EDGE('',*,*,#13889,.T.);
#18101=ORIENTED_EDGE('',*,*,#13890,.T.);
#18102=ORIENTED_EDGE('',*,*,#13891,.T.);
#18103=ORIENTED_EDGE('',*,*,#13892,.T.);
#18104=ORIENTED_EDGE('',*,*,#13893,.T.);
#18105=ORIENTED_EDGE('',*,*,#13894,.T.);
#18106=ORIENTED_EDGE('',*,*,#13895,.T.);
#18107=ORIENTED_EDGE('',*,*,#13896,.T.);
#18108=ORIENTED_EDGE('',*,*,#13897,.T.);
#18109=ORIENTED_EDGE('',*,*,#13898,.T.);
#18110=ORIENTED_EDGE('',*,*,#13899,.F.);
#18111=ORIENTED_EDGE('',*,*,#13900,.T.);
#18112=ORIENTED_EDGE('',*,*,#13901,.T.);
#18113=ORIENTED_EDGE('',*,*,#13902,.F.);
#18114=ORIENTED_EDGE('',*,*,#13903,.T.);
#18115=ORIENTED_EDGE('',*,*,#13904,.T.);
#18116=ORIENTED_EDGE('',*,*,#13905,.T.);
#18117=ORIENTED_EDGE('',*,*,#13906,.T.);
#18118=ORIENTED_EDGE('',*,*,#13907,.T.);
#18119=ORIENTED_EDGE('',*,*,#13908,.T.);
#18120=ORIENTED_EDGE('',*,*,#13909,.T.);
#18121=ORIENTED_EDGE('',*,*,#13910,.T.);
#18122=ORIENTED_EDGE('',*,*,#13911,.T.);
#18123=ORIENTED_EDGE('',*,*,#13912,.T.);
#18124=ORIENTED_EDGE('',*,*,#13913,.T.);
#18125=ORIENTED_EDGE('',*,*,#13914,.T.);
#18126=ORIENTED_EDGE('',*,*,#13915,.T.);
#18127=ORIENTED_EDGE('',*,*,#13916,.T.);
#18128=ORIENTED_EDGE('',*,*,#13917,.T.);
#18129=ORIENTED_EDGE('',*,*,#13918,.T.);
#18130=ORIENTED_EDGE('',*,*,#13919,.F.);
#18131=ORIENTED_EDGE('',*,*,#13920,.T.);
#18132=ORIENTED_EDGE('',*,*,#13921,.T.);
#18133=ORIENTED_EDGE('',*,*,#13922,.F.);
#18134=ORIENTED_EDGE('',*,*,#13923,.T.);
#18135=ORIENTED_EDGE('',*,*,#13924,.T.);
#18136=ORIENTED_EDGE('',*,*,#13925,.T.);
#18137=ORIENTED_EDGE('',*,*,#13926,.T.);
#18138=ORIENTED_EDGE('',*,*,#13927,.T.);
#18139=ORIENTED_EDGE('',*,*,#13928,.T.);
#18140=ORIENTED_EDGE('',*,*,#13929,.T.);
#18141=ORIENTED_EDGE('',*,*,#13930,.T.);
#18142=ORIENTED_EDGE('',*,*,#13931,.T.);
#18143=ORIENTED_EDGE('',*,*,#13932,.T.);
#18144=ORIENTED_EDGE('',*,*,#13933,.T.);
#18145=ORIENTED_EDGE('',*,*,#13934,.T.);
#18146=ORIENTED_EDGE('',*,*,#13935,.T.);
#18147=ORIENTED_EDGE('',*,*,#13936,.T.);
#18148=ORIENTED_EDGE('',*,*,#13937,.T.);
#18149=ORIENTED_EDGE('',*,*,#13938,.T.);
#18150=ORIENTED_EDGE('',*,*,#13939,.F.);
#18151=ORIENTED_EDGE('',*,*,#13940,.T.);
#18152=ORIENTED_EDGE('',*,*,#13941,.T.);
#18153=ORIENTED_EDGE('',*,*,#13942,.F.);
#18154=ORIENTED_EDGE('',*,*,#13943,.T.);
#18155=ORIENTED_EDGE('',*,*,#13944,.T.);
#18156=ORIENTED_EDGE('',*,*,#13945,.T.);
#18157=ORIENTED_EDGE('',*,*,#13946,.T.);
#18158=ORIENTED_EDGE('',*,*,#13947,.T.);
#18159=ORIENTED_EDGE('',*,*,#13948,.T.);
#18160=ORIENTED_EDGE('',*,*,#13949,.T.);
#18161=ORIENTED_EDGE('',*,*,#13950,.T.);
#18162=ORIENTED_EDGE('',*,*,#13951,.T.);
#18163=ORIENTED_EDGE('',*,*,#13952,.T.);
#18164=ORIENTED_EDGE('',*,*,#13953,.T.);
#18165=ORIENTED_EDGE('',*,*,#13954,.T.);
#18166=ORIENTED_EDGE('',*,*,#13955,.T.);
#18167=ORIENTED_EDGE('',*,*,#13956,.T.);
#18168=ORIENTED_EDGE('',*,*,#13957,.T.);
#18169=ORIENTED_EDGE('',*,*,#13958,.T.);
#18170=ORIENTED_EDGE('',*,*,#13959,.F.);
#18171=ORIENTED_EDGE('',*,*,#13960,.T.);
#18172=ORIENTED_EDGE('',*,*,#13961,.F.);
#18173=ORIENTED_EDGE('',*,*,#13716,.F.);
#18174=ORIENTED_EDGE('',*,*,#13962,.T.);
#18175=ORIENTED_EDGE('',*,*,#13963,.F.);
#18176=ORIENTED_EDGE('',*,*,#13964,.F.);
#18177=ORIENTED_EDGE('',*,*,#13965,.F.);
#18178=ORIENTED_EDGE('',*,*,#13723,.F.);
#18179=ORIENTED_EDGE('',*,*,#13721,.F.);
#18180=ORIENTED_EDGE('',*,*,#13966,.T.);
#18181=ORIENTED_EDGE('',*,*,#13967,.F.);
#18182=ORIENTED_EDGE('',*,*,#13962,.F.);
#18183=ORIENTED_EDGE('',*,*,#13968,.T.);
#18184=ORIENTED_EDGE('',*,*,#13942,.T.);
#18185=ORIENTED_EDGE('',*,*,#13969,.T.);
#18186=ORIENTED_EDGE('',*,*,#13970,.T.);
#18187=ORIENTED_EDGE('',*,*,#13971,.T.);
#18188=ORIENTED_EDGE('',*,*,#13972,.T.);
#18189=ORIENTED_EDGE('',*,*,#13968,.F.);
#18190=ORIENTED_EDGE('',*,*,#13973,.T.);
#18191=ORIENTED_EDGE('',*,*,#13974,.F.);
#18192=ORIENTED_EDGE('',*,*,#13975,.F.);
#18193=ORIENTED_EDGE('',*,*,#13976,.F.);
#18194=ORIENTED_EDGE('',*,*,#13943,.F.);
#18195=ORIENTED_EDGE('',*,*,#13972,.F.);
#18196=ORIENTED_EDGE('',*,*,#13977,.T.);
#18197=ORIENTED_EDGE('',*,*,#13978,.F.);
#18198=ORIENTED_EDGE('',*,*,#13973,.F.);
#18199=ORIENTED_EDGE('',*,*,#13979,.T.);
#18200=ORIENTED_EDGE('',*,*,#13922,.T.);
#18201=ORIENTED_EDGE('',*,*,#13980,.T.);
#18202=ORIENTED_EDGE('',*,*,#13981,.T.);
#18203=ORIENTED_EDGE('',*,*,#13982,.T.);
#18204=ORIENTED_EDGE('',*,*,#13983,.T.);
#18205=ORIENTED_EDGE('',*,*,#13979,.F.);
#18206=ORIENTED_EDGE('',*,*,#13984,.T.);
#18207=ORIENTED_EDGE('',*,*,#13985,.F.);
#18208=ORIENTED_EDGE('',*,*,#13986,.F.);
#18209=ORIENTED_EDGE('',*,*,#13987,.F.);
#18210=ORIENTED_EDGE('',*,*,#13923,.F.);
#18211=ORIENTED_EDGE('',*,*,#13983,.F.);
#18212=ORIENTED_EDGE('',*,*,#13988,.T.);
#18213=ORIENTED_EDGE('',*,*,#13989,.F.);
#18214=ORIENTED_EDGE('',*,*,#13984,.F.);
#18215=ORIENTED_EDGE('',*,*,#13990,.T.);
#18216=ORIENTED_EDGE('',*,*,#13902,.T.);
#18217=ORIENTED_EDGE('',*,*,#13991,.T.);
#18218=ORIENTED_EDGE('',*,*,#13992,.T.);
#18219=ORIENTED_EDGE('',*,*,#13993,.T.);
#18220=ORIENTED_EDGE('',*,*,#13994,.T.);
#18221=ORIENTED_EDGE('',*,*,#13990,.F.);
#18222=ORIENTED_EDGE('',*,*,#13995,.T.);
#18223=ORIENTED_EDGE('',*,*,#13996,.F.);
#18224=ORIENTED_EDGE('',*,*,#13997,.F.);
#18225=ORIENTED_EDGE('',*,*,#13998,.F.);
#18226=ORIENTED_EDGE('',*,*,#13903,.F.);
#18227=ORIENTED_EDGE('',*,*,#13994,.F.);
#18228=ORIENTED_EDGE('',*,*,#13999,.T.);
#18229=ORIENTED_EDGE('',*,*,#14000,.F.);
#18230=ORIENTED_EDGE('',*,*,#13995,.F.);
#18231=ORIENTED_EDGE('',*,*,#14001,.T.);
#18232=ORIENTED_EDGE('',*,*,#13882,.T.);
#18233=ORIENTED_EDGE('',*,*,#14002,.T.);
#18234=ORIENTED_EDGE('',*,*,#14003,.T.);
#18235=ORIENTED_EDGE('',*,*,#14004,.T.);
#18236=ORIENTED_EDGE('',*,*,#14005,.T.);
#18237=ORIENTED_EDGE('',*,*,#14001,.F.);
#18238=ORIENTED_EDGE('',*,*,#14006,.T.);
#18239=ORIENTED_EDGE('',*,*,#14007,.F.);
#18240=ORIENTED_EDGE('',*,*,#14008,.F.);
#18241=ORIENTED_EDGE('',*,*,#14009,.F.);
#18242=ORIENTED_EDGE('',*,*,#13883,.F.);
#18243=ORIENTED_EDGE('',*,*,#14005,.F.);
#18244=ORIENTED_EDGE('',*,*,#14010,.T.);
#18245=ORIENTED_EDGE('',*,*,#14011,.F.);
#18246=ORIENTED_EDGE('',*,*,#14006,.F.);
#18247=ORIENTED_EDGE('',*,*,#14012,.T.);
#18248=ORIENTED_EDGE('',*,*,#13862,.T.);
#18249=ORIENTED_EDGE('',*,*,#14013,.T.);
#18250=ORIENTED_EDGE('',*,*,#14014,.T.);
#18251=ORIENTED_EDGE('',*,*,#14015,.T.);
#18252=ORIENTED_EDGE('',*,*,#14016,.T.);
#18253=ORIENTED_EDGE('',*,*,#14012,.F.);
#18254=ORIENTED_EDGE('',*,*,#14017,.T.);
#18255=ORIENTED_EDGE('',*,*,#14018,.F.);
#18256=ORIENTED_EDGE('',*,*,#14019,.F.);
#18257=ORIENTED_EDGE('',*,*,#14020,.F.);
#18258=ORIENTED_EDGE('',*,*,#13863,.F.);
#18259=ORIENTED_EDGE('',*,*,#14016,.F.);
#18260=ORIENTED_EDGE('',*,*,#14021,.T.);
#18261=ORIENTED_EDGE('',*,*,#14022,.F.);
#18262=ORIENTED_EDGE('',*,*,#14017,.F.);
#18263=ORIENTED_EDGE('',*,*,#14023,.T.);
#18264=ORIENTED_EDGE('',*,*,#13842,.T.);
#18265=ORIENTED_EDGE('',*,*,#14024,.T.);
#18266=ORIENTED_EDGE('',*,*,#14025,.T.);
#18267=ORIENTED_EDGE('',*,*,#14026,.T.);
#18268=ORIENTED_EDGE('',*,*,#14027,.T.);
#18269=ORIENTED_EDGE('',*,*,#14023,.F.);
#18270=ORIENTED_EDGE('',*,*,#14028,.T.);
#18271=ORIENTED_EDGE('',*,*,#14029,.F.);
#18272=ORIENTED_EDGE('',*,*,#14030,.F.);
#18273=ORIENTED_EDGE('',*,*,#14031,.F.);
#18274=ORIENTED_EDGE('',*,*,#13843,.F.);
#18275=ORIENTED_EDGE('',*,*,#14027,.F.);
#18276=ORIENTED_EDGE('',*,*,#14032,.T.);
#18277=ORIENTED_EDGE('',*,*,#14033,.F.);
#18278=ORIENTED_EDGE('',*,*,#14028,.F.);
#18279=ORIENTED_EDGE('',*,*,#14034,.T.);
#18280=ORIENTED_EDGE('',*,*,#13822,.T.);
#18281=ORIENTED_EDGE('',*,*,#14035,.T.);
#18282=ORIENTED_EDGE('',*,*,#14036,.T.);
#18283=ORIENTED_EDGE('',*,*,#14037,.T.);
#18284=ORIENTED_EDGE('',*,*,#14038,.T.);
#18285=ORIENTED_EDGE('',*,*,#14034,.F.);
#18286=ORIENTED_EDGE('',*,*,#14039,.T.);
#18287=ORIENTED_EDGE('',*,*,#14040,.F.);
#18288=ORIENTED_EDGE('',*,*,#14041,.F.);
#18289=ORIENTED_EDGE('',*,*,#14042,.F.);
#18290=ORIENTED_EDGE('',*,*,#13823,.F.);
#18291=ORIENTED_EDGE('',*,*,#14038,.F.);
#18292=ORIENTED_EDGE('',*,*,#14043,.T.);
#18293=ORIENTED_EDGE('',*,*,#14044,.F.);
#18294=ORIENTED_EDGE('',*,*,#14039,.F.);
#18295=ORIENTED_EDGE('',*,*,#14045,.T.);
#18296=ORIENTED_EDGE('',*,*,#13802,.T.);
#18297=ORIENTED_EDGE('',*,*,#14046,.T.);
#18298=ORIENTED_EDGE('',*,*,#14047,.T.);
#18299=ORIENTED_EDGE('',*,*,#14048,.T.);
#18300=ORIENTED_EDGE('',*,*,#14049,.T.);
#18301=ORIENTED_EDGE('',*,*,#14045,.F.);
#18302=ORIENTED_EDGE('',*,*,#14050,.T.);
#18303=ORIENTED_EDGE('',*,*,#14051,.F.);
#18304=ORIENTED_EDGE('',*,*,#14052,.F.);
#18305=ORIENTED_EDGE('',*,*,#14053,.F.);
#18306=ORIENTED_EDGE('',*,*,#13803,.F.);
#18307=ORIENTED_EDGE('',*,*,#14049,.F.);
#18308=ORIENTED_EDGE('',*,*,#14054,.T.);
#18309=ORIENTED_EDGE('',*,*,#14055,.F.);
#18310=ORIENTED_EDGE('',*,*,#14050,.F.);
#18311=ORIENTED_EDGE('',*,*,#14056,.T.);
#18312=ORIENTED_EDGE('',*,*,#13782,.T.);
#18313=ORIENTED_EDGE('',*,*,#14057,.T.);
#18314=ORIENTED_EDGE('',*,*,#14058,.T.);
#18315=ORIENTED_EDGE('',*,*,#14059,.T.);
#18316=ORIENTED_EDGE('',*,*,#14060,.T.);
#18317=ORIENTED_EDGE('',*,*,#14056,.F.);
#18318=ORIENTED_EDGE('',*,*,#14061,.T.);
#18319=ORIENTED_EDGE('',*,*,#14062,.F.);
#18320=ORIENTED_EDGE('',*,*,#14063,.F.);
#18321=ORIENTED_EDGE('',*,*,#14064,.F.);
#18322=ORIENTED_EDGE('',*,*,#13783,.F.);
#18323=ORIENTED_EDGE('',*,*,#14060,.F.);
#18324=ORIENTED_EDGE('',*,*,#14065,.T.);
#18325=ORIENTED_EDGE('',*,*,#14066,.F.);
#18326=ORIENTED_EDGE('',*,*,#14061,.F.);
#18327=ORIENTED_EDGE('',*,*,#14067,.T.);
#18328=ORIENTED_EDGE('',*,*,#13762,.T.);
#18329=ORIENTED_EDGE('',*,*,#14068,.T.);
#18330=ORIENTED_EDGE('',*,*,#14069,.T.);
#18331=ORIENTED_EDGE('',*,*,#14070,.T.);
#18332=ORIENTED_EDGE('',*,*,#14071,.T.);
#18333=ORIENTED_EDGE('',*,*,#14067,.F.);
#18334=ORIENTED_EDGE('',*,*,#14072,.T.);
#18335=ORIENTED_EDGE('',*,*,#14073,.F.);
#18336=ORIENTED_EDGE('',*,*,#14074,.F.);
#18337=ORIENTED_EDGE('',*,*,#14075,.F.);
#18338=ORIENTED_EDGE('',*,*,#13763,.F.);
#18339=ORIENTED_EDGE('',*,*,#14071,.F.);
#18340=ORIENTED_EDGE('',*,*,#14076,.T.);
#18341=ORIENTED_EDGE('',*,*,#14077,.F.);
#18342=ORIENTED_EDGE('',*,*,#14072,.F.);
#18343=ORIENTED_EDGE('',*,*,#14078,.T.);
#18344=ORIENTED_EDGE('',*,*,#13742,.T.);
#18345=ORIENTED_EDGE('',*,*,#14079,.T.);
#18346=ORIENTED_EDGE('',*,*,#14080,.T.);
#18347=ORIENTED_EDGE('',*,*,#14081,.T.);
#18348=ORIENTED_EDGE('',*,*,#14082,.T.);
#18349=ORIENTED_EDGE('',*,*,#14078,.F.);
#18350=ORIENTED_EDGE('',*,*,#14083,.T.);
#18351=ORIENTED_EDGE('',*,*,#14084,.F.);
#18352=ORIENTED_EDGE('',*,*,#14085,.F.);
#18353=ORIENTED_EDGE('',*,*,#14086,.F.);
#18354=ORIENTED_EDGE('',*,*,#13743,.F.);
#18355=ORIENTED_EDGE('',*,*,#14082,.F.);
#18356=ORIENTED_EDGE('',*,*,#14087,.T.);
#18357=ORIENTED_EDGE('',*,*,#14088,.F.);
#18358=ORIENTED_EDGE('',*,*,#14083,.F.);
#18359=ORIENTED_EDGE('',*,*,#14089,.T.);
#18360=ORIENTED_EDGE('',*,*,#14090,.T.);
#18361=ORIENTED_EDGE('',*,*,#14091,.T.);
#18362=ORIENTED_EDGE('',*,*,#13739,.T.);
#18363=ORIENTED_EDGE('',*,*,#14092,.T.);
#18364=ORIENTED_EDGE('',*,*,#14093,.T.);
#18365=ORIENTED_EDGE('',*,*,#14090,.F.);
#18366=ORIENTED_EDGE('',*,*,#14094,.T.);
#18367=ORIENTED_EDGE('',*,*,#14095,.F.);
#18368=ORIENTED_EDGE('',*,*,#14096,.F.);
#18369=ORIENTED_EDGE('',*,*,#14089,.F.);
#18370=ORIENTED_EDGE('',*,*,#14097,.T.);
#18371=ORIENTED_EDGE('',*,*,#14098,.F.);
#18372=ORIENTED_EDGE('',*,*,#14094,.F.);
#18373=ORIENTED_EDGE('',*,*,#14099,.T.);
#18374=ORIENTED_EDGE('',*,*,#14100,.T.);
#18375=ORIENTED_EDGE('',*,*,#14101,.T.);
#18376=ORIENTED_EDGE('',*,*,#13959,.T.);
#18377=ORIENTED_EDGE('',*,*,#14102,.T.);
#18378=ORIENTED_EDGE('',*,*,#14103,.T.);
#18379=ORIENTED_EDGE('',*,*,#14100,.F.);
#18380=ORIENTED_EDGE('',*,*,#14104,.T.);
#18381=ORIENTED_EDGE('',*,*,#14105,.F.);
#18382=ORIENTED_EDGE('',*,*,#14106,.F.);
#18383=ORIENTED_EDGE('',*,*,#14099,.F.);
#18384=ORIENTED_EDGE('',*,*,#14107,.T.);
#18385=ORIENTED_EDGE('',*,*,#14108,.F.);
#18386=ORIENTED_EDGE('',*,*,#14104,.F.);
#18387=ORIENTED_EDGE('',*,*,#14109,.T.);
#18388=ORIENTED_EDGE('',*,*,#14110,.T.);
#18389=ORIENTED_EDGE('',*,*,#14111,.T.);
#18390=ORIENTED_EDGE('',*,*,#13939,.T.);
#18391=ORIENTED_EDGE('',*,*,#14112,.T.);
#18392=ORIENTED_EDGE('',*,*,#14113,.T.);
#18393=ORIENTED_EDGE('',*,*,#14110,.F.);
#18394=ORIENTED_EDGE('',*,*,#14114,.T.);
#18395=ORIENTED_EDGE('',*,*,#14115,.F.);
#18396=ORIENTED_EDGE('',*,*,#14116,.F.);
#18397=ORIENTED_EDGE('',*,*,#14109,.F.);
#18398=ORIENTED_EDGE('',*,*,#14117,.T.);
#18399=ORIENTED_EDGE('',*,*,#14118,.F.);
#18400=ORIENTED_EDGE('',*,*,#14114,.F.);
#18401=ORIENTED_EDGE('',*,*,#14119,.T.);
#18402=ORIENTED_EDGE('',*,*,#14120,.T.);
#18403=ORIENTED_EDGE('',*,*,#14121,.T.);
#18404=ORIENTED_EDGE('',*,*,#13919,.T.);
#18405=ORIENTED_EDGE('',*,*,#14122,.T.);
#18406=ORIENTED_EDGE('',*,*,#14123,.T.);
#18407=ORIENTED_EDGE('',*,*,#14120,.F.);
#18408=ORIENTED_EDGE('',*,*,#14124,.T.);
#18409=ORIENTED_EDGE('',*,*,#14125,.F.);
#18410=ORIENTED_EDGE('',*,*,#14126,.F.);
#18411=ORIENTED_EDGE('',*,*,#14119,.F.);
#18412=ORIENTED_EDGE('',*,*,#14127,.T.);
#18413=ORIENTED_EDGE('',*,*,#14128,.F.);
#18414=ORIENTED_EDGE('',*,*,#14124,.F.);
#18415=ORIENTED_EDGE('',*,*,#14129,.T.);
#18416=ORIENTED_EDGE('',*,*,#14130,.T.);
#18417=ORIENTED_EDGE('',*,*,#14131,.T.);
#18418=ORIENTED_EDGE('',*,*,#13899,.T.);
#18419=ORIENTED_EDGE('',*,*,#14132,.T.);
#18420=ORIENTED_EDGE('',*,*,#14133,.T.);
#18421=ORIENTED_EDGE('',*,*,#14130,.F.);
#18422=ORIENTED_EDGE('',*,*,#14134,.T.);
#18423=ORIENTED_EDGE('',*,*,#14135,.F.);
#18424=ORIENTED_EDGE('',*,*,#14136,.F.);
#18425=ORIENTED_EDGE('',*,*,#14129,.F.);
#18426=ORIENTED_EDGE('',*,*,#14137,.T.);
#18427=ORIENTED_EDGE('',*,*,#14138,.F.);
#18428=ORIENTED_EDGE('',*,*,#14134,.F.);
#18429=ORIENTED_EDGE('',*,*,#14139,.T.);
#18430=ORIENTED_EDGE('',*,*,#14140,.T.);
#18431=ORIENTED_EDGE('',*,*,#14141,.T.);
#18432=ORIENTED_EDGE('',*,*,#13879,.T.);
#18433=ORIENTED_EDGE('',*,*,#14142,.T.);
#18434=ORIENTED_EDGE('',*,*,#14143,.T.);
#18435=ORIENTED_EDGE('',*,*,#14140,.F.);
#18436=ORIENTED_EDGE('',*,*,#14144,.T.);
#18437=ORIENTED_EDGE('',*,*,#14145,.F.);
#18438=ORIENTED_EDGE('',*,*,#14146,.F.);
#18439=ORIENTED_EDGE('',*,*,#14139,.F.);
#18440=ORIENTED_EDGE('',*,*,#14147,.T.);
#18441=ORIENTED_EDGE('',*,*,#14148,.F.);
#18442=ORIENTED_EDGE('',*,*,#14144,.F.);
#18443=ORIENTED_EDGE('',*,*,#14149,.T.);
#18444=ORIENTED_EDGE('',*,*,#14150,.T.);
#18445=ORIENTED_EDGE('',*,*,#14151,.T.);
#18446=ORIENTED_EDGE('',*,*,#13859,.T.);
#18447=ORIENTED_EDGE('',*,*,#14152,.T.);
#18448=ORIENTED_EDGE('',*,*,#14153,.T.);
#18449=ORIENTED_EDGE('',*,*,#14150,.F.);
#18450=ORIENTED_EDGE('',*,*,#14154,.T.);
#18451=ORIENTED_EDGE('',*,*,#14155,.F.);
#18452=ORIENTED_EDGE('',*,*,#14156,.F.);
#18453=ORIENTED_EDGE('',*,*,#14149,.F.);
#18454=ORIENTED_EDGE('',*,*,#14157,.T.);
#18455=ORIENTED_EDGE('',*,*,#14158,.F.);
#18456=ORIENTED_EDGE('',*,*,#14154,.F.);
#18457=ORIENTED_EDGE('',*,*,#14159,.T.);
#18458=ORIENTED_EDGE('',*,*,#14160,.T.);
#18459=ORIENTED_EDGE('',*,*,#14161,.T.);
#18460=ORIENTED_EDGE('',*,*,#13839,.T.);
#18461=ORIENTED_EDGE('',*,*,#14162,.T.);
#18462=ORIENTED_EDGE('',*,*,#14163,.T.);
#18463=ORIENTED_EDGE('',*,*,#14160,.F.);
#18464=ORIENTED_EDGE('',*,*,#14164,.T.);
#18465=ORIENTED_EDGE('',*,*,#14165,.F.);
#18466=ORIENTED_EDGE('',*,*,#14166,.F.);
#18467=ORIENTED_EDGE('',*,*,#14159,.F.);
#18468=ORIENTED_EDGE('',*,*,#14167,.T.);
#18469=ORIENTED_EDGE('',*,*,#14168,.F.);
#18470=ORIENTED_EDGE('',*,*,#14164,.F.);
#18471=ORIENTED_EDGE('',*,*,#14169,.T.);
#18472=ORIENTED_EDGE('',*,*,#14170,.T.);
#18473=ORIENTED_EDGE('',*,*,#14171,.T.);
#18474=ORIENTED_EDGE('',*,*,#13819,.T.);
#18475=ORIENTED_EDGE('',*,*,#14172,.T.);
#18476=ORIENTED_EDGE('',*,*,#14173,.T.);
#18477=ORIENTED_EDGE('',*,*,#14170,.F.);
#18478=ORIENTED_EDGE('',*,*,#14174,.T.);
#18479=ORIENTED_EDGE('',*,*,#14175,.F.);
#18480=ORIENTED_EDGE('',*,*,#14176,.F.);
#18481=ORIENTED_EDGE('',*,*,#14169,.F.);
#18482=ORIENTED_EDGE('',*,*,#14177,.T.);
#18483=ORIENTED_EDGE('',*,*,#14178,.F.);
#18484=ORIENTED_EDGE('',*,*,#14174,.F.);
#18485=ORIENTED_EDGE('',*,*,#14179,.T.);
#18486=ORIENTED_EDGE('',*,*,#14180,.T.);
#18487=ORIENTED_EDGE('',*,*,#14181,.T.);
#18488=ORIENTED_EDGE('',*,*,#13799,.T.);
#18489=ORIENTED_EDGE('',*,*,#14182,.T.);
#18490=ORIENTED_EDGE('',*,*,#14183,.T.);
#18491=ORIENTED_EDGE('',*,*,#14180,.F.);
#18492=ORIENTED_EDGE('',*,*,#14184,.T.);
#18493=ORIENTED_EDGE('',*,*,#14185,.F.);
#18494=ORIENTED_EDGE('',*,*,#14186,.F.);
#18495=ORIENTED_EDGE('',*,*,#14179,.F.);
#18496=ORIENTED_EDGE('',*,*,#14187,.T.);
#18497=ORIENTED_EDGE('',*,*,#14188,.F.);
#18498=ORIENTED_EDGE('',*,*,#14184,.F.);
#18499=ORIENTED_EDGE('',*,*,#14189,.T.);
#18500=ORIENTED_EDGE('',*,*,#14190,.T.);
#18501=ORIENTED_EDGE('',*,*,#14191,.T.);
#18502=ORIENTED_EDGE('',*,*,#13779,.T.);
#18503=ORIENTED_EDGE('',*,*,#14192,.T.);
#18504=ORIENTED_EDGE('',*,*,#14193,.T.);
#18505=ORIENTED_EDGE('',*,*,#14190,.F.);
#18506=ORIENTED_EDGE('',*,*,#14194,.T.);
#18507=ORIENTED_EDGE('',*,*,#14195,.F.);
#18508=ORIENTED_EDGE('',*,*,#14196,.F.);
#18509=ORIENTED_EDGE('',*,*,#14189,.F.);
#18510=ORIENTED_EDGE('',*,*,#14197,.T.);
#18511=ORIENTED_EDGE('',*,*,#14198,.F.);
#18512=ORIENTED_EDGE('',*,*,#14194,.F.);
#18513=ORIENTED_EDGE('',*,*,#14199,.T.);
#18514=ORIENTED_EDGE('',*,*,#14200,.T.);
#18515=ORIENTED_EDGE('',*,*,#14201,.T.);
#18516=ORIENTED_EDGE('',*,*,#13759,.T.);
#18517=ORIENTED_EDGE('',*,*,#14202,.T.);
#18518=ORIENTED_EDGE('',*,*,#14203,.T.);
#18519=ORIENTED_EDGE('',*,*,#14200,.F.);
#18520=ORIENTED_EDGE('',*,*,#14204,.T.);
#18521=ORIENTED_EDGE('',*,*,#14205,.F.);
#18522=ORIENTED_EDGE('',*,*,#14206,.F.);
#18523=ORIENTED_EDGE('',*,*,#14199,.F.);
#18524=ORIENTED_EDGE('',*,*,#14207,.T.);
#18525=ORIENTED_EDGE('',*,*,#14208,.F.);
#18526=ORIENTED_EDGE('',*,*,#14204,.F.);
#18527=ORIENTED_EDGE('',*,*,#14209,.T.);
#18528=ORIENTED_EDGE('',*,*,#14210,.T.);
#18529=ORIENTED_EDGE('',*,*,#14211,.T.);
#18530=ORIENTED_EDGE('',*,*,#14212,.T.);
#18531=ORIENTED_EDGE('',*,*,#14084,.T.);
#18532=ORIENTED_EDGE('',*,*,#14088,.T.);
#18533=ORIENTED_EDGE('',*,*,#14212,.F.);
#18534=ORIENTED_EDGE('',*,*,#14213,.T.);
#18535=ORIENTED_EDGE('',*,*,#14214,.T.);
#18536=ORIENTED_EDGE('',*,*,#14215,.F.);
#18537=ORIENTED_EDGE('',*,*,#14216,.T.);
#18538=ORIENTED_EDGE('',*,*,#14217,.T.);
#18539=ORIENTED_EDGE('',*,*,#14218,.T.);
#18540=ORIENTED_EDGE('',*,*,#14219,.T.);
#18541=ORIENTED_EDGE('',*,*,#14220,.T.);
#18542=ORIENTED_EDGE('',*,*,#14221,.T.);
#18543=ORIENTED_EDGE('',*,*,#14222,.T.);
#18544=ORIENTED_EDGE('',*,*,#14223,.T.);
#18545=ORIENTED_EDGE('',*,*,#14224,.T.);
#18546=ORIENTED_EDGE('',*,*,#14225,.T.);
#18547=ORIENTED_EDGE('',*,*,#14226,.T.);
#18548=ORIENTED_EDGE('',*,*,#14227,.T.);
#18549=ORIENTED_EDGE('',*,*,#14228,.T.);
#18550=ORIENTED_EDGE('',*,*,#14229,.T.);
#18551=ORIENTED_EDGE('',*,*,#14230,.T.);
#18552=ORIENTED_EDGE('',*,*,#13964,.T.);
#18553=ORIENTED_EDGE('',*,*,#14231,.F.);
#18554=ORIENTED_EDGE('',*,*,#14232,.T.);
#18555=ORIENTED_EDGE('',*,*,#14233,.T.);
#18556=ORIENTED_EDGE('',*,*,#14234,.F.);
#18557=ORIENTED_EDGE('',*,*,#14235,.T.);
#18558=ORIENTED_EDGE('',*,*,#14236,.T.);
#18559=ORIENTED_EDGE('',*,*,#14237,.T.);
#18560=ORIENTED_EDGE('',*,*,#14238,.T.);
#18561=ORIENTED_EDGE('',*,*,#14239,.T.);
#18562=ORIENTED_EDGE('',*,*,#14240,.T.);
#18563=ORIENTED_EDGE('',*,*,#14241,.T.);
#18564=ORIENTED_EDGE('',*,*,#14242,.T.);
#18565=ORIENTED_EDGE('',*,*,#14243,.T.);
#18566=ORIENTED_EDGE('',*,*,#14244,.T.);
#18567=ORIENTED_EDGE('',*,*,#14245,.T.);
#18568=ORIENTED_EDGE('',*,*,#14246,.T.);
#18569=ORIENTED_EDGE('',*,*,#14247,.T.);
#18570=ORIENTED_EDGE('',*,*,#14248,.T.);
#18571=ORIENTED_EDGE('',*,*,#14249,.T.);
#18572=ORIENTED_EDGE('',*,*,#13975,.T.);
#18573=ORIENTED_EDGE('',*,*,#14250,.F.);
#18574=ORIENTED_EDGE('',*,*,#14251,.T.);
#18575=ORIENTED_EDGE('',*,*,#14252,.T.);
#18576=ORIENTED_EDGE('',*,*,#14253,.F.);
#18577=ORIENTED_EDGE('',*,*,#14254,.T.);
#18578=ORIENTED_EDGE('',*,*,#14255,.T.);
#18579=ORIENTED_EDGE('',*,*,#14256,.T.);
#18580=ORIENTED_EDGE('',*,*,#14257,.T.);
#18581=ORIENTED_EDGE('',*,*,#14258,.T.);
#18582=ORIENTED_EDGE('',*,*,#14259,.T.);
#18583=ORIENTED_EDGE('',*,*,#14260,.T.);
#18584=ORIENTED_EDGE('',*,*,#14261,.T.);
#18585=ORIENTED_EDGE('',*,*,#14262,.T.);
#18586=ORIENTED_EDGE('',*,*,#14263,.T.);
#18587=ORIENTED_EDGE('',*,*,#14264,.T.);
#18588=ORIENTED_EDGE('',*,*,#14265,.T.);
#18589=ORIENTED_EDGE('',*,*,#14266,.T.);
#18590=ORIENTED_EDGE('',*,*,#14267,.T.);
#18591=ORIENTED_EDGE('',*,*,#14268,.T.);
#18592=ORIENTED_EDGE('',*,*,#13986,.T.);
#18593=ORIENTED_EDGE('',*,*,#14269,.F.);
#18594=ORIENTED_EDGE('',*,*,#14270,.T.);
#18595=ORIENTED_EDGE('',*,*,#14271,.T.);
#18596=ORIENTED_EDGE('',*,*,#14272,.F.);
#18597=ORIENTED_EDGE('',*,*,#14273,.T.);
#18598=ORIENTED_EDGE('',*,*,#14274,.T.);
#18599=ORIENTED_EDGE('',*,*,#14275,.T.);
#18600=ORIENTED_EDGE('',*,*,#14276,.T.);
#18601=ORIENTED_EDGE('',*,*,#14277,.T.);
#18602=ORIENTED_EDGE('',*,*,#14278,.T.);
#18603=ORIENTED_EDGE('',*,*,#14279,.T.);
#18604=ORIENTED_EDGE('',*,*,#14280,.T.);
#18605=ORIENTED_EDGE('',*,*,#14281,.T.);
#18606=ORIENTED_EDGE('',*,*,#14282,.T.);
#18607=ORIENTED_EDGE('',*,*,#14283,.T.);
#18608=ORIENTED_EDGE('',*,*,#14284,.T.);
#18609=ORIENTED_EDGE('',*,*,#14285,.T.);
#18610=ORIENTED_EDGE('',*,*,#14286,.T.);
#18611=ORIENTED_EDGE('',*,*,#14287,.T.);
#18612=ORIENTED_EDGE('',*,*,#13997,.T.);
#18613=ORIENTED_EDGE('',*,*,#14288,.F.);
#18614=ORIENTED_EDGE('',*,*,#14289,.T.);
#18615=ORIENTED_EDGE('',*,*,#14290,.T.);
#18616=ORIENTED_EDGE('',*,*,#14291,.F.);
#18617=ORIENTED_EDGE('',*,*,#14292,.T.);
#18618=ORIENTED_EDGE('',*,*,#14293,.T.);
#18619=ORIENTED_EDGE('',*,*,#14294,.T.);
#18620=ORIENTED_EDGE('',*,*,#14295,.T.);
#18621=ORIENTED_EDGE('',*,*,#14296,.T.);
#18622=ORIENTED_EDGE('',*,*,#14297,.T.);
#18623=ORIENTED_EDGE('',*,*,#14298,.T.);
#18624=ORIENTED_EDGE('',*,*,#14299,.T.);
#18625=ORIENTED_EDGE('',*,*,#14300,.T.);
#18626=ORIENTED_EDGE('',*,*,#14301,.T.);
#18627=ORIENTED_EDGE('',*,*,#14302,.T.);
#18628=ORIENTED_EDGE('',*,*,#14303,.T.);
#18629=ORIENTED_EDGE('',*,*,#14304,.T.);
#18630=ORIENTED_EDGE('',*,*,#14305,.T.);
#18631=ORIENTED_EDGE('',*,*,#14306,.T.);
#18632=ORIENTED_EDGE('',*,*,#14008,.T.);
#18633=ORIENTED_EDGE('',*,*,#14307,.F.);
#18634=ORIENTED_EDGE('',*,*,#14308,.T.);
#18635=ORIENTED_EDGE('',*,*,#14309,.T.);
#18636=ORIENTED_EDGE('',*,*,#14310,.F.);
#18637=ORIENTED_EDGE('',*,*,#14311,.T.);
#18638=ORIENTED_EDGE('',*,*,#14312,.T.);
#18639=ORIENTED_EDGE('',*,*,#14313,.T.);
#18640=ORIENTED_EDGE('',*,*,#14314,.T.);
#18641=ORIENTED_EDGE('',*,*,#14315,.T.);
#18642=ORIENTED_EDGE('',*,*,#14316,.T.);
#18643=ORIENTED_EDGE('',*,*,#14317,.T.);
#18644=ORIENTED_EDGE('',*,*,#14318,.T.);
#18645=ORIENTED_EDGE('',*,*,#14319,.T.);
#18646=ORIENTED_EDGE('',*,*,#14320,.T.);
#18647=ORIENTED_EDGE('',*,*,#14321,.T.);
#18648=ORIENTED_EDGE('',*,*,#14322,.T.);
#18649=ORIENTED_EDGE('',*,*,#14323,.T.);
#18650=ORIENTED_EDGE('',*,*,#14324,.T.);
#18651=ORIENTED_EDGE('',*,*,#14325,.T.);
#18652=ORIENTED_EDGE('',*,*,#14019,.T.);
#18653=ORIENTED_EDGE('',*,*,#14326,.F.);
#18654=ORIENTED_EDGE('',*,*,#14327,.T.);
#18655=ORIENTED_EDGE('',*,*,#14328,.T.);
#18656=ORIENTED_EDGE('',*,*,#14329,.F.);
#18657=ORIENTED_EDGE('',*,*,#14330,.T.);
#18658=ORIENTED_EDGE('',*,*,#14331,.T.);
#18659=ORIENTED_EDGE('',*,*,#14332,.T.);
#18660=ORIENTED_EDGE('',*,*,#14333,.T.);
#18661=ORIENTED_EDGE('',*,*,#14334,.T.);
#18662=ORIENTED_EDGE('',*,*,#14335,.T.);
#18663=ORIENTED_EDGE('',*,*,#14336,.T.);
#18664=ORIENTED_EDGE('',*,*,#14337,.T.);
#18665=ORIENTED_EDGE('',*,*,#14338,.T.);
#18666=ORIENTED_EDGE('',*,*,#14339,.T.);
#18667=ORIENTED_EDGE('',*,*,#14340,.T.);
#18668=ORIENTED_EDGE('',*,*,#14341,.T.);
#18669=ORIENTED_EDGE('',*,*,#14342,.T.);
#18670=ORIENTED_EDGE('',*,*,#14343,.T.);
#18671=ORIENTED_EDGE('',*,*,#14344,.T.);
#18672=ORIENTED_EDGE('',*,*,#14030,.T.);
#18673=ORIENTED_EDGE('',*,*,#14345,.F.);
#18674=ORIENTED_EDGE('',*,*,#14346,.T.);
#18675=ORIENTED_EDGE('',*,*,#14347,.T.);
#18676=ORIENTED_EDGE('',*,*,#14348,.F.);
#18677=ORIENTED_EDGE('',*,*,#14349,.T.);
#18678=ORIENTED_EDGE('',*,*,#14350,.T.);
#18679=ORIENTED_EDGE('',*,*,#14351,.T.);
#18680=ORIENTED_EDGE('',*,*,#14352,.T.);
#18681=ORIENTED_EDGE('',*,*,#14353,.T.);
#18682=ORIENTED_EDGE('',*,*,#14354,.T.);
#18683=ORIENTED_EDGE('',*,*,#14355,.T.);
#18684=ORIENTED_EDGE('',*,*,#14356,.T.);
#18685=ORIENTED_EDGE('',*,*,#14357,.T.);
#18686=ORIENTED_EDGE('',*,*,#14358,.T.);
#18687=ORIENTED_EDGE('',*,*,#14359,.T.);
#18688=ORIENTED_EDGE('',*,*,#14360,.T.);
#18689=ORIENTED_EDGE('',*,*,#14361,.T.);
#18690=ORIENTED_EDGE('',*,*,#14362,.T.);
#18691=ORIENTED_EDGE('',*,*,#14363,.T.);
#18692=ORIENTED_EDGE('',*,*,#14041,.T.);
#18693=ORIENTED_EDGE('',*,*,#14364,.F.);
#18694=ORIENTED_EDGE('',*,*,#14365,.T.);
#18695=ORIENTED_EDGE('',*,*,#14366,.T.);
#18696=ORIENTED_EDGE('',*,*,#14367,.F.);
#18697=ORIENTED_EDGE('',*,*,#14368,.T.);
#18698=ORIENTED_EDGE('',*,*,#14369,.T.);
#18699=ORIENTED_EDGE('',*,*,#14370,.T.);
#18700=ORIENTED_EDGE('',*,*,#14371,.T.);
#18701=ORIENTED_EDGE('',*,*,#14372,.T.);
#18702=ORIENTED_EDGE('',*,*,#14373,.T.);
#18703=ORIENTED_EDGE('',*,*,#14374,.T.);
#18704=ORIENTED_EDGE('',*,*,#14375,.T.);
#18705=ORIENTED_EDGE('',*,*,#14376,.T.);
#18706=ORIENTED_EDGE('',*,*,#14377,.T.);
#18707=ORIENTED_EDGE('',*,*,#14378,.T.);
#18708=ORIENTED_EDGE('',*,*,#14379,.T.);
#18709=ORIENTED_EDGE('',*,*,#14380,.T.);
#18710=ORIENTED_EDGE('',*,*,#14381,.T.);
#18711=ORIENTED_EDGE('',*,*,#14382,.T.);
#18712=ORIENTED_EDGE('',*,*,#14052,.T.);
#18713=ORIENTED_EDGE('',*,*,#14383,.F.);
#18714=ORIENTED_EDGE('',*,*,#14384,.T.);
#18715=ORIENTED_EDGE('',*,*,#14385,.T.);
#18716=ORIENTED_EDGE('',*,*,#14386,.F.);
#18717=ORIENTED_EDGE('',*,*,#14387,.T.);
#18718=ORIENTED_EDGE('',*,*,#14388,.T.);
#18719=ORIENTED_EDGE('',*,*,#14389,.T.);
#18720=ORIENTED_EDGE('',*,*,#14390,.T.);
#18721=ORIENTED_EDGE('',*,*,#14391,.T.);
#18722=ORIENTED_EDGE('',*,*,#14392,.T.);
#18723=ORIENTED_EDGE('',*,*,#14393,.T.);
#18724=ORIENTED_EDGE('',*,*,#14394,.T.);
#18725=ORIENTED_EDGE('',*,*,#14395,.T.);
#18726=ORIENTED_EDGE('',*,*,#14396,.T.);
#18727=ORIENTED_EDGE('',*,*,#14397,.T.);
#18728=ORIENTED_EDGE('',*,*,#14398,.T.);
#18729=ORIENTED_EDGE('',*,*,#14399,.T.);
#18730=ORIENTED_EDGE('',*,*,#14400,.T.);
#18731=ORIENTED_EDGE('',*,*,#14401,.T.);
#18732=ORIENTED_EDGE('',*,*,#14063,.T.);
#18733=ORIENTED_EDGE('',*,*,#14402,.F.);
#18734=ORIENTED_EDGE('',*,*,#14403,.T.);
#18735=ORIENTED_EDGE('',*,*,#14404,.T.);
#18736=ORIENTED_EDGE('',*,*,#14405,.F.);
#18737=ORIENTED_EDGE('',*,*,#14406,.T.);
#18738=ORIENTED_EDGE('',*,*,#14407,.T.);
#18739=ORIENTED_EDGE('',*,*,#14408,.T.);
#18740=ORIENTED_EDGE('',*,*,#14409,.T.);
#18741=ORIENTED_EDGE('',*,*,#14410,.T.);
#18742=ORIENTED_EDGE('',*,*,#14411,.T.);
#18743=ORIENTED_EDGE('',*,*,#14412,.T.);
#18744=ORIENTED_EDGE('',*,*,#14413,.T.);
#18745=ORIENTED_EDGE('',*,*,#14414,.T.);
#18746=ORIENTED_EDGE('',*,*,#14415,.T.);
#18747=ORIENTED_EDGE('',*,*,#14416,.T.);
#18748=ORIENTED_EDGE('',*,*,#14417,.T.);
#18749=ORIENTED_EDGE('',*,*,#14418,.T.);
#18750=ORIENTED_EDGE('',*,*,#14419,.T.);
#18751=ORIENTED_EDGE('',*,*,#14420,.T.);
#18752=ORIENTED_EDGE('',*,*,#14074,.T.);
#18753=ORIENTED_EDGE('',*,*,#14421,.F.);
#18754=ORIENTED_EDGE('',*,*,#14422,.T.);
#18755=ORIENTED_EDGE('',*,*,#14423,.T.);
#18756=ORIENTED_EDGE('',*,*,#14424,.F.);
#18757=ORIENTED_EDGE('',*,*,#14425,.T.);
#18758=ORIENTED_EDGE('',*,*,#14426,.T.);
#18759=ORIENTED_EDGE('',*,*,#14427,.T.);
#18760=ORIENTED_EDGE('',*,*,#14428,.T.);
#18761=ORIENTED_EDGE('',*,*,#14429,.T.);
#18762=ORIENTED_EDGE('',*,*,#14430,.T.);
#18763=ORIENTED_EDGE('',*,*,#14431,.T.);
#18764=ORIENTED_EDGE('',*,*,#14432,.T.);
#18765=ORIENTED_EDGE('',*,*,#14433,.T.);
#18766=ORIENTED_EDGE('',*,*,#14434,.T.);
#18767=ORIENTED_EDGE('',*,*,#14435,.T.);
#18768=ORIENTED_EDGE('',*,*,#14436,.T.);
#18769=ORIENTED_EDGE('',*,*,#14437,.T.);
#18770=ORIENTED_EDGE('',*,*,#14438,.T.);
#18771=ORIENTED_EDGE('',*,*,#14439,.T.);
#18772=ORIENTED_EDGE('',*,*,#14085,.T.);
#18773=ORIENTED_EDGE('',*,*,#14440,.F.);
#18774=ORIENTED_EDGE('',*,*,#14441,.T.);
#18775=ORIENTED_EDGE('',*,*,#14424,.T.);
#18776=ORIENTED_EDGE('',*,*,#14442,.T.);
#18777=ORIENTED_EDGE('',*,*,#14205,.T.);
#18778=ORIENTED_EDGE('',*,*,#14208,.T.);
#18779=ORIENTED_EDGE('',*,*,#14443,.T.);
#18780=ORIENTED_EDGE('',*,*,#14444,.T.);
#18781=ORIENTED_EDGE('',*,*,#14445,.T.);
#18782=ORIENTED_EDGE('',*,*,#14446,.T.);
#18783=ORIENTED_EDGE('',*,*,#14421,.T.);
#18784=ORIENTED_EDGE('',*,*,#14073,.T.);
#18785=ORIENTED_EDGE('',*,*,#14077,.T.);
#18786=ORIENTED_EDGE('',*,*,#14447,.T.);
#18787=ORIENTED_EDGE('',*,*,#14405,.T.);
#18788=ORIENTED_EDGE('',*,*,#14448,.T.);
#18789=ORIENTED_EDGE('',*,*,#14195,.T.);
#18790=ORIENTED_EDGE('',*,*,#14198,.T.);
#18791=ORIENTED_EDGE('',*,*,#14449,.T.);
#18792=ORIENTED_EDGE('',*,*,#14450,.T.);
#18793=ORIENTED_EDGE('',*,*,#14451,.T.);
#18794=ORIENTED_EDGE('',*,*,#14452,.T.);
#18795=ORIENTED_EDGE('',*,*,#14402,.T.);
#18796=ORIENTED_EDGE('',*,*,#14062,.T.);
#18797=ORIENTED_EDGE('',*,*,#14066,.T.);
#18798=ORIENTED_EDGE('',*,*,#14453,.T.);
#18799=ORIENTED_EDGE('',*,*,#14386,.T.);
#18800=ORIENTED_EDGE('',*,*,#14454,.T.);
#18801=ORIENTED_EDGE('',*,*,#14185,.T.);
#18802=ORIENTED_EDGE('',*,*,#14188,.T.);
#18803=ORIENTED_EDGE('',*,*,#14455,.T.);
#18804=ORIENTED_EDGE('',*,*,#14456,.T.);
#18805=ORIENTED_EDGE('',*,*,#14457,.T.);
#18806=ORIENTED_EDGE('',*,*,#14458,.T.);
#18807=ORIENTED_EDGE('',*,*,#14383,.T.);
#18808=ORIENTED_EDGE('',*,*,#14051,.T.);
#18809=ORIENTED_EDGE('',*,*,#14055,.T.);
#18810=ORIENTED_EDGE('',*,*,#14459,.T.);
#18811=ORIENTED_EDGE('',*,*,#14367,.T.);
#18812=ORIENTED_EDGE('',*,*,#14460,.T.);
#18813=ORIENTED_EDGE('',*,*,#14175,.T.);
#18814=ORIENTED_EDGE('',*,*,#14178,.T.);
#18815=ORIENTED_EDGE('',*,*,#14461,.T.);
#18816=ORIENTED_EDGE('',*,*,#14462,.T.);
#18817=ORIENTED_EDGE('',*,*,#14463,.T.);
#18818=ORIENTED_EDGE('',*,*,#14464,.T.);
#18819=ORIENTED_EDGE('',*,*,#14364,.T.);
#18820=ORIENTED_EDGE('',*,*,#14040,.T.);
#18821=ORIENTED_EDGE('',*,*,#14044,.T.);
#18822=ORIENTED_EDGE('',*,*,#14465,.T.);
#18823=ORIENTED_EDGE('',*,*,#14348,.T.);
#18824=ORIENTED_EDGE('',*,*,#14466,.T.);
#18825=ORIENTED_EDGE('',*,*,#14165,.T.);
#18826=ORIENTED_EDGE('',*,*,#14168,.T.);
#18827=ORIENTED_EDGE('',*,*,#14467,.T.);
#18828=ORIENTED_EDGE('',*,*,#14468,.T.);
#18829=ORIENTED_EDGE('',*,*,#14469,.T.);
#18830=ORIENTED_EDGE('',*,*,#14470,.T.);
#18831=ORIENTED_EDGE('',*,*,#14345,.T.);
#18832=ORIENTED_EDGE('',*,*,#14029,.T.);
#18833=ORIENTED_EDGE('',*,*,#14033,.T.);
#18834=ORIENTED_EDGE('',*,*,#14471,.T.);
#18835=ORIENTED_EDGE('',*,*,#14329,.T.);
#18836=ORIENTED_EDGE('',*,*,#14472,.T.);
#18837=ORIENTED_EDGE('',*,*,#14155,.T.);
#18838=ORIENTED_EDGE('',*,*,#14158,.T.);
#18839=ORIENTED_EDGE('',*,*,#14473,.T.);
#18840=ORIENTED_EDGE('',*,*,#14474,.T.);
#18841=ORIENTED_EDGE('',*,*,#14475,.T.);
#18842=ORIENTED_EDGE('',*,*,#14476,.T.);
#18843=ORIENTED_EDGE('',*,*,#14326,.T.);
#18844=ORIENTED_EDGE('',*,*,#14018,.T.);
#18845=ORIENTED_EDGE('',*,*,#14022,.T.);
#18846=ORIENTED_EDGE('',*,*,#14477,.T.);
#18847=ORIENTED_EDGE('',*,*,#14310,.T.);
#18848=ORIENTED_EDGE('',*,*,#14478,.T.);
#18849=ORIENTED_EDGE('',*,*,#14145,.T.);
#18850=ORIENTED_EDGE('',*,*,#14148,.T.);
#18851=ORIENTED_EDGE('',*,*,#14479,.T.);
#18852=ORIENTED_EDGE('',*,*,#14480,.T.);
#18853=ORIENTED_EDGE('',*,*,#14481,.T.);
#18854=ORIENTED_EDGE('',*,*,#14482,.T.);
#18855=ORIENTED_EDGE('',*,*,#14307,.T.);
#18856=ORIENTED_EDGE('',*,*,#14007,.T.);
#18857=ORIENTED_EDGE('',*,*,#14011,.T.);
#18858=ORIENTED_EDGE('',*,*,#14483,.T.);
#18859=ORIENTED_EDGE('',*,*,#14291,.T.);
#18860=ORIENTED_EDGE('',*,*,#14484,.T.);
#18861=ORIENTED_EDGE('',*,*,#14135,.T.);
#18862=ORIENTED_EDGE('',*,*,#14138,.T.);
#18863=ORIENTED_EDGE('',*,*,#14485,.T.);
#18864=ORIENTED_EDGE('',*,*,#14486,.T.);
#18865=ORIENTED_EDGE('',*,*,#14487,.T.);
#18866=ORIENTED_EDGE('',*,*,#14488,.T.);
#18867=ORIENTED_EDGE('',*,*,#14288,.T.);
#18868=ORIENTED_EDGE('',*,*,#13996,.T.);
#18869=ORIENTED_EDGE('',*,*,#14000,.T.);
#18870=ORIENTED_EDGE('',*,*,#14489,.T.);
#18871=ORIENTED_EDGE('',*,*,#14272,.T.);
#18872=ORIENTED_EDGE('',*,*,#14490,.T.);
#18873=ORIENTED_EDGE('',*,*,#14125,.T.);
#18874=ORIENTED_EDGE('',*,*,#14128,.T.);
#18875=ORIENTED_EDGE('',*,*,#14491,.T.);
#18876=ORIENTED_EDGE('',*,*,#14492,.T.);
#18877=ORIENTED_EDGE('',*,*,#14493,.T.);
#18878=ORIENTED_EDGE('',*,*,#14494,.T.);
#18879=ORIENTED_EDGE('',*,*,#14269,.T.);
#18880=ORIENTED_EDGE('',*,*,#13985,.T.);
#18881=ORIENTED_EDGE('',*,*,#13989,.T.);
#18882=ORIENTED_EDGE('',*,*,#14495,.T.);
#18883=ORIENTED_EDGE('',*,*,#14253,.T.);
#18884=ORIENTED_EDGE('',*,*,#14496,.T.);
#18885=ORIENTED_EDGE('',*,*,#14115,.T.);
#18886=ORIENTED_EDGE('',*,*,#14118,.T.);
#18887=ORIENTED_EDGE('',*,*,#14497,.T.);
#18888=ORIENTED_EDGE('',*,*,#14498,.T.);
#18889=ORIENTED_EDGE('',*,*,#14499,.T.);
#18890=ORIENTED_EDGE('',*,*,#14500,.T.);
#18891=ORIENTED_EDGE('',*,*,#14250,.T.);
#18892=ORIENTED_EDGE('',*,*,#13974,.T.);
#18893=ORIENTED_EDGE('',*,*,#13978,.T.);
#18894=ORIENTED_EDGE('',*,*,#14501,.T.);
#18895=ORIENTED_EDGE('',*,*,#14234,.T.);
#18896=ORIENTED_EDGE('',*,*,#14502,.T.);
#18897=ORIENTED_EDGE('',*,*,#14105,.T.);
#18898=ORIENTED_EDGE('',*,*,#14108,.T.);
#18899=ORIENTED_EDGE('',*,*,#14503,.T.);
#18900=ORIENTED_EDGE('',*,*,#14504,.T.);
#18901=ORIENTED_EDGE('',*,*,#14505,.T.);
#18902=ORIENTED_EDGE('',*,*,#14506,.T.);
#18903=ORIENTED_EDGE('',*,*,#14231,.T.);
#18904=ORIENTED_EDGE('',*,*,#13963,.T.);
#18905=ORIENTED_EDGE('',*,*,#13967,.T.);
#18906=ORIENTED_EDGE('',*,*,#14507,.T.);
#18907=ORIENTED_EDGE('',*,*,#14215,.T.);
#18908=ORIENTED_EDGE('',*,*,#14508,.T.);
#18909=ORIENTED_EDGE('',*,*,#14095,.T.);
#18910=ORIENTED_EDGE('',*,*,#14098,.T.);
#18911=ORIENTED_EDGE('',*,*,#14509,.T.);
#18912=ORIENTED_EDGE('',*,*,#14510,.F.);
#18913=ORIENTED_EDGE('',*,*,#14511,.T.);
#18914=ORIENTED_EDGE('',*,*,#14512,.T.);
#18915=ORIENTED_EDGE('',*,*,#14513,.F.);
#18916=ORIENTED_EDGE('',*,*,#14514,.F.);
#18917=ORIENTED_EDGE('',*,*,#14513,.T.);
#18918=ORIENTED_EDGE('',*,*,#14515,.T.);
#18919=ORIENTED_EDGE('',*,*,#14516,.F.);
#18920=ORIENTED_EDGE('',*,*,#14517,.F.);
#18921=ORIENTED_EDGE('',*,*,#14518,.T.);
#18922=ORIENTED_EDGE('',*,*,#14519,.T.);
#18923=ORIENTED_EDGE('',*,*,#14511,.F.);
#18924=ORIENTED_EDGE('',*,*,#14520,.F.);
#18925=ORIENTED_EDGE('',*,*,#14516,.T.);
#18926=ORIENTED_EDGE('',*,*,#14521,.T.);
#18927=ORIENTED_EDGE('',*,*,#14518,.F.);
#18928=ORIENTED_EDGE('',*,*,#14515,.F.);
#18929=ORIENTED_EDGE('',*,*,#14512,.F.);
#18930=ORIENTED_EDGE('',*,*,#14519,.F.);
#18931=ORIENTED_EDGE('',*,*,#14521,.F.);
#18932=ORIENTED_EDGE('',*,*,#13741,.F.);
#18933=ORIENTED_EDGE('',*,*,#14522,.T.);
#18934=ORIENTED_EDGE('',*,*,#14213,.F.);
#18935=ORIENTED_EDGE('',*,*,#14211,.F.);
#18936=ORIENTED_EDGE('',*,*,#14523,.F.);
#18937=ORIENTED_EDGE('',*,*,#14079,.F.);
#18938=ORIENTED_EDGE('',*,*,#14080,.F.);
#18939=ORIENTED_EDGE('',*,*,#14523,.T.);
#18940=ORIENTED_EDGE('',*,*,#14210,.F.);
#18941=ORIENTED_EDGE('',*,*,#14524,.F.);
#18942=ORIENTED_EDGE('',*,*,#14081,.F.);
#18943=ORIENTED_EDGE('',*,*,#14524,.T.);
#18944=ORIENTED_EDGE('',*,*,#14209,.F.);
#18945=ORIENTED_EDGE('',*,*,#14087,.F.);
#18946=ORIENTED_EDGE('',*,*,#13744,.F.);
#18947=ORIENTED_EDGE('',*,*,#14086,.T.);
#18948=ORIENTED_EDGE('',*,*,#14439,.F.);
#18949=ORIENTED_EDGE('',*,*,#14525,.F.);
#18950=ORIENTED_EDGE('',*,*,#13745,.F.);
#18951=ORIENTED_EDGE('',*,*,#14525,.T.);
#18952=ORIENTED_EDGE('',*,*,#14438,.F.);
#18953=ORIENTED_EDGE('',*,*,#14526,.F.);
#18954=ORIENTED_EDGE('',*,*,#13746,.F.);
#18955=ORIENTED_EDGE('',*,*,#14526,.T.);
#18956=ORIENTED_EDGE('',*,*,#14437,.F.);
#18957=ORIENTED_EDGE('',*,*,#14527,.F.);
#18958=ORIENTED_EDGE('',*,*,#13747,.F.);
#18959=ORIENTED_EDGE('',*,*,#14527,.T.);
#18960=ORIENTED_EDGE('',*,*,#14436,.F.);
#18961=ORIENTED_EDGE('',*,*,#14528,.F.);
#18962=ORIENTED_EDGE('',*,*,#13748,.F.);
#18963=ORIENTED_EDGE('',*,*,#14528,.T.);
#18964=ORIENTED_EDGE('',*,*,#14435,.F.);
#18965=ORIENTED_EDGE('',*,*,#14529,.F.);
#18966=ORIENTED_EDGE('',*,*,#13749,.F.);
#18967=ORIENTED_EDGE('',*,*,#14529,.T.);
#18968=ORIENTED_EDGE('',*,*,#14434,.F.);
#18969=ORIENTED_EDGE('',*,*,#14530,.F.);
#18970=ORIENTED_EDGE('',*,*,#13750,.F.);
#18971=ORIENTED_EDGE('',*,*,#14530,.T.);
#18972=ORIENTED_EDGE('',*,*,#14433,.F.);
#18973=ORIENTED_EDGE('',*,*,#14531,.F.);
#18974=ORIENTED_EDGE('',*,*,#13751,.F.);
#18975=ORIENTED_EDGE('',*,*,#14531,.T.);
#18976=ORIENTED_EDGE('',*,*,#14432,.F.);
#18977=ORIENTED_EDGE('',*,*,#14532,.F.);
#18978=ORIENTED_EDGE('',*,*,#13752,.F.);
#18979=ORIENTED_EDGE('',*,*,#14532,.T.);
#18980=ORIENTED_EDGE('',*,*,#14431,.F.);
#18981=ORIENTED_EDGE('',*,*,#14533,.F.);
#18982=ORIENTED_EDGE('',*,*,#13753,.F.);
#18983=ORIENTED_EDGE('',*,*,#14533,.T.);
#18984=ORIENTED_EDGE('',*,*,#14430,.F.);
#18985=ORIENTED_EDGE('',*,*,#14534,.F.);
#18986=ORIENTED_EDGE('',*,*,#13754,.F.);
#18987=ORIENTED_EDGE('',*,*,#14534,.T.);
#18988=ORIENTED_EDGE('',*,*,#14429,.F.);
#18989=ORIENTED_EDGE('',*,*,#14535,.F.);
#18990=ORIENTED_EDGE('',*,*,#13755,.F.);
#18991=ORIENTED_EDGE('',*,*,#14535,.T.);
#18992=ORIENTED_EDGE('',*,*,#14428,.F.);
#18993=ORIENTED_EDGE('',*,*,#14536,.F.);
#18994=ORIENTED_EDGE('',*,*,#13756,.F.);
#18995=ORIENTED_EDGE('',*,*,#14536,.T.);
#18996=ORIENTED_EDGE('',*,*,#14427,.F.);
#18997=ORIENTED_EDGE('',*,*,#14537,.F.);
#18998=ORIENTED_EDGE('',*,*,#13757,.F.);
#18999=ORIENTED_EDGE('',*,*,#14537,.T.);
#19000=ORIENTED_EDGE('',*,*,#14426,.F.);
#19001=ORIENTED_EDGE('',*,*,#14538,.F.);
#19002=ORIENTED_EDGE('',*,*,#14202,.F.);
#19003=ORIENTED_EDGE('',*,*,#13758,.F.);
#19004=ORIENTED_EDGE('',*,*,#14538,.T.);
#19005=ORIENTED_EDGE('',*,*,#14425,.F.);
#19006=ORIENTED_EDGE('',*,*,#14441,.F.);
#19007=ORIENTED_EDGE('',*,*,#14539,.F.);
#19008=ORIENTED_EDGE('',*,*,#14203,.F.);
#19009=ORIENTED_EDGE('',*,*,#14539,.T.);
#19010=ORIENTED_EDGE('',*,*,#14443,.F.);
#19011=ORIENTED_EDGE('',*,*,#14207,.F.);
#19012=ORIENTED_EDGE('',*,*,#13760,.F.);
#19013=ORIENTED_EDGE('',*,*,#14201,.F.);
#19014=ORIENTED_EDGE('',*,*,#14206,.T.);
#19015=ORIENTED_EDGE('',*,*,#14442,.F.);
#19016=ORIENTED_EDGE('',*,*,#14423,.F.);
#19017=ORIENTED_EDGE('',*,*,#14540,.F.);
#19018=ORIENTED_EDGE('',*,*,#13761,.F.);
#19019=ORIENTED_EDGE('',*,*,#14540,.T.);
#19020=ORIENTED_EDGE('',*,*,#14422,.F.);
#19021=ORIENTED_EDGE('',*,*,#14446,.F.);
#19022=ORIENTED_EDGE('',*,*,#14541,.F.);
#19023=ORIENTED_EDGE('',*,*,#14068,.F.);
#19024=ORIENTED_EDGE('',*,*,#14069,.F.);
#19025=ORIENTED_EDGE('',*,*,#14541,.T.);
#19026=ORIENTED_EDGE('',*,*,#14445,.F.);
#19027=ORIENTED_EDGE('',*,*,#14542,.F.);
#19028=ORIENTED_EDGE('',*,*,#14070,.F.);
#19029=ORIENTED_EDGE('',*,*,#14542,.T.);
#19030=ORIENTED_EDGE('',*,*,#14444,.F.);
#19031=ORIENTED_EDGE('',*,*,#14076,.F.);
#19032=ORIENTED_EDGE('',*,*,#13764,.F.);
#19033=ORIENTED_EDGE('',*,*,#14075,.T.);
#19034=ORIENTED_EDGE('',*,*,#14420,.F.);
#19035=ORIENTED_EDGE('',*,*,#14543,.F.);
#19036=ORIENTED_EDGE('',*,*,#13765,.F.);
#19037=ORIENTED_EDGE('',*,*,#14543,.T.);
#19038=ORIENTED_EDGE('',*,*,#14419,.F.);
#19039=ORIENTED_EDGE('',*,*,#14544,.F.);
#19040=ORIENTED_EDGE('',*,*,#13766,.F.);
#19041=ORIENTED_EDGE('',*,*,#14544,.T.);
#19042=ORIENTED_EDGE('',*,*,#14418,.F.);
#19043=ORIENTED_EDGE('',*,*,#14545,.F.);
#19044=ORIENTED_EDGE('',*,*,#13767,.F.);
#19045=ORIENTED_EDGE('',*,*,#14545,.T.);
#19046=ORIENTED_EDGE('',*,*,#14417,.F.);
#19047=ORIENTED_EDGE('',*,*,#14546,.F.);
#19048=ORIENTED_EDGE('',*,*,#13768,.F.);
#19049=ORIENTED_EDGE('',*,*,#14546,.T.);
#19050=ORIENTED_EDGE('',*,*,#14416,.F.);
#19051=ORIENTED_EDGE('',*,*,#14547,.F.);
#19052=ORIENTED_EDGE('',*,*,#13769,.F.);
#19053=ORIENTED_EDGE('',*,*,#14547,.T.);
#19054=ORIENTED_EDGE('',*,*,#14415,.F.);
#19055=ORIENTED_EDGE('',*,*,#14548,.F.);
#19056=ORIENTED_EDGE('',*,*,#13770,.F.);
#19057=ORIENTED_EDGE('',*,*,#14548,.T.);
#19058=ORIENTED_EDGE('',*,*,#14414,.F.);
#19059=ORIENTED_EDGE('',*,*,#14549,.F.);
#19060=ORIENTED_EDGE('',*,*,#13771,.F.);
#19061=ORIENTED_EDGE('',*,*,#14549,.T.);
#19062=ORIENTED_EDGE('',*,*,#14413,.F.);
#19063=ORIENTED_EDGE('',*,*,#14550,.F.);
#19064=ORIENTED_EDGE('',*,*,#13772,.F.);
#19065=ORIENTED_EDGE('',*,*,#14550,.T.);
#19066=ORIENTED_EDGE('',*,*,#14412,.F.);
#19067=ORIENTED_EDGE('',*,*,#14551,.F.);
#19068=ORIENTED_EDGE('',*,*,#13773,.F.);
#19069=ORIENTED_EDGE('',*,*,#14551,.T.);
#19070=ORIENTED_EDGE('',*,*,#14411,.F.);
#19071=ORIENTED_EDGE('',*,*,#14552,.F.);
#19072=ORIENTED_EDGE('',*,*,#13774,.F.);
#19073=ORIENTED_EDGE('',*,*,#14552,.T.);
#19074=ORIENTED_EDGE('',*,*,#14410,.F.);
#19075=ORIENTED_EDGE('',*,*,#14553,.F.);
#19076=ORIENTED_EDGE('',*,*,#13775,.F.);
#19077=ORIENTED_EDGE('',*,*,#14553,.T.);
#19078=ORIENTED_EDGE('',*,*,#14409,.F.);
#19079=ORIENTED_EDGE('',*,*,#14554,.F.);
#19080=ORIENTED_EDGE('',*,*,#13776,.F.);
#19081=ORIENTED_EDGE('',*,*,#14554,.T.);
#19082=ORIENTED_EDGE('',*,*,#14408,.F.);
#19083=ORIENTED_EDGE('',*,*,#14555,.F.);
#19084=ORIENTED_EDGE('',*,*,#13777,.F.);
#19085=ORIENTED_EDGE('',*,*,#14555,.T.);
#19086=ORIENTED_EDGE('',*,*,#14407,.F.);
#19087=ORIENTED_EDGE('',*,*,#14556,.F.);
#19088=ORIENTED_EDGE('',*,*,#14192,.F.);
#19089=ORIENTED_EDGE('',*,*,#13778,.F.);
#19090=ORIENTED_EDGE('',*,*,#14556,.T.);
#19091=ORIENTED_EDGE('',*,*,#14406,.F.);
#19092=ORIENTED_EDGE('',*,*,#14447,.F.);
#19093=ORIENTED_EDGE('',*,*,#14557,.F.);
#19094=ORIENTED_EDGE('',*,*,#14193,.F.);
#19095=ORIENTED_EDGE('',*,*,#14557,.T.);
#19096=ORIENTED_EDGE('',*,*,#14449,.F.);
#19097=ORIENTED_EDGE('',*,*,#14197,.F.);
#19098=ORIENTED_EDGE('',*,*,#13780,.F.);
#19099=ORIENTED_EDGE('',*,*,#14191,.F.);
#19100=ORIENTED_EDGE('',*,*,#14196,.T.);
#19101=ORIENTED_EDGE('',*,*,#14448,.F.);
#19102=ORIENTED_EDGE('',*,*,#14404,.F.);
#19103=ORIENTED_EDGE('',*,*,#14558,.F.);
#19104=ORIENTED_EDGE('',*,*,#13781,.F.);
#19105=ORIENTED_EDGE('',*,*,#14558,.T.);
#19106=ORIENTED_EDGE('',*,*,#14403,.F.);
#19107=ORIENTED_EDGE('',*,*,#14452,.F.);
#19108=ORIENTED_EDGE('',*,*,#14559,.F.);
#19109=ORIENTED_EDGE('',*,*,#14057,.F.);
#19110=ORIENTED_EDGE('',*,*,#14058,.F.);
#19111=ORIENTED_EDGE('',*,*,#14559,.T.);
#19112=ORIENTED_EDGE('',*,*,#14451,.F.);
#19113=ORIENTED_EDGE('',*,*,#14560,.F.);
#19114=ORIENTED_EDGE('',*,*,#14059,.F.);
#19115=ORIENTED_EDGE('',*,*,#14560,.T.);
#19116=ORIENTED_EDGE('',*,*,#14450,.F.);
#19117=ORIENTED_EDGE('',*,*,#14065,.F.);
#19118=ORIENTED_EDGE('',*,*,#13784,.F.);
#19119=ORIENTED_EDGE('',*,*,#14064,.T.);
#19120=ORIENTED_EDGE('',*,*,#14401,.F.);
#19121=ORIENTED_EDGE('',*,*,#14561,.F.);
#19122=ORIENTED_EDGE('',*,*,#13785,.F.);
#19123=ORIENTED_EDGE('',*,*,#14561,.T.);
#19124=ORIENTED_EDGE('',*,*,#14400,.F.);
#19125=ORIENTED_EDGE('',*,*,#14562,.F.);
#19126=ORIENTED_EDGE('',*,*,#13786,.F.);
#19127=ORIENTED_EDGE('',*,*,#14562,.T.);
#19128=ORIENTED_EDGE('',*,*,#14399,.F.);
#19129=ORIENTED_EDGE('',*,*,#14563,.F.);
#19130=ORIENTED_EDGE('',*,*,#13787,.F.);
#19131=ORIENTED_EDGE('',*,*,#14563,.T.);
#19132=ORIENTED_EDGE('',*,*,#14398,.F.);
#19133=ORIENTED_EDGE('',*,*,#14564,.F.);
#19134=ORIENTED_EDGE('',*,*,#13788,.F.);
#19135=ORIENTED_EDGE('',*,*,#14564,.T.);
#19136=ORIENTED_EDGE('',*,*,#14397,.F.);
#19137=ORIENTED_EDGE('',*,*,#14565,.F.);
#19138=ORIENTED_EDGE('',*,*,#13789,.F.);
#19139=ORIENTED_EDGE('',*,*,#14565,.T.);
#19140=ORIENTED_EDGE('',*,*,#14396,.F.);
#19141=ORIENTED_EDGE('',*,*,#14566,.F.);
#19142=ORIENTED_EDGE('',*,*,#13790,.F.);
#19143=ORIENTED_EDGE('',*,*,#14566,.T.);
#19144=ORIENTED_EDGE('',*,*,#14395,.F.);
#19145=ORIENTED_EDGE('',*,*,#14567,.F.);
#19146=ORIENTED_EDGE('',*,*,#13791,.F.);
#19147=ORIENTED_EDGE('',*,*,#14567,.T.);
#19148=ORIENTED_EDGE('',*,*,#14394,.F.);
#19149=ORIENTED_EDGE('',*,*,#14568,.F.);
#19150=ORIENTED_EDGE('',*,*,#13792,.F.);
#19151=ORIENTED_EDGE('',*,*,#14568,.T.);
#19152=ORIENTED_EDGE('',*,*,#14393,.F.);
#19153=ORIENTED_EDGE('',*,*,#14569,.F.);
#19154=ORIENTED_EDGE('',*,*,#13793,.F.);
#19155=ORIENTED_EDGE('',*,*,#14569,.T.);
#19156=ORIENTED_EDGE('',*,*,#14392,.F.);
#19157=ORIENTED_EDGE('',*,*,#14570,.F.);
#19158=ORIENTED_EDGE('',*,*,#13794,.F.);
#19159=ORIENTED_EDGE('',*,*,#14570,.T.);
#19160=ORIENTED_EDGE('',*,*,#14391,.F.);
#19161=ORIENTED_EDGE('',*,*,#14571,.F.);
#19162=ORIENTED_EDGE('',*,*,#13795,.F.);
#19163=ORIENTED_EDGE('',*,*,#14571,.T.);
#19164=ORIENTED_EDGE('',*,*,#14390,.F.);
#19165=ORIENTED_EDGE('',*,*,#14572,.F.);
#19166=ORIENTED_EDGE('',*,*,#13796,.F.);
#19167=ORIENTED_EDGE('',*,*,#14572,.T.);
#19168=ORIENTED_EDGE('',*,*,#14389,.F.);
#19169=ORIENTED_EDGE('',*,*,#14573,.F.);
#19170=ORIENTED_EDGE('',*,*,#13797,.F.);
#19171=ORIENTED_EDGE('',*,*,#14573,.T.);
#19172=ORIENTED_EDGE('',*,*,#14388,.F.);
#19173=ORIENTED_EDGE('',*,*,#14574,.F.);
#19174=ORIENTED_EDGE('',*,*,#14182,.F.);
#19175=ORIENTED_EDGE('',*,*,#13798,.F.);
#19176=ORIENTED_EDGE('',*,*,#14574,.T.);
#19177=ORIENTED_EDGE('',*,*,#14387,.F.);
#19178=ORIENTED_EDGE('',*,*,#14453,.F.);
#19179=ORIENTED_EDGE('',*,*,#14575,.F.);
#19180=ORIENTED_EDGE('',*,*,#14183,.F.);
#19181=ORIENTED_EDGE('',*,*,#14575,.T.);
#19182=ORIENTED_EDGE('',*,*,#14455,.F.);
#19183=ORIENTED_EDGE('',*,*,#14187,.F.);
#19184=ORIENTED_EDGE('',*,*,#13800,.F.);
#19185=ORIENTED_EDGE('',*,*,#14181,.F.);
#19186=ORIENTED_EDGE('',*,*,#14186,.T.);
#19187=ORIENTED_EDGE('',*,*,#14454,.F.);
#19188=ORIENTED_EDGE('',*,*,#14385,.F.);
#19189=ORIENTED_EDGE('',*,*,#14576,.F.);
#19190=ORIENTED_EDGE('',*,*,#13801,.F.);
#19191=ORIENTED_EDGE('',*,*,#14576,.T.);
#19192=ORIENTED_EDGE('',*,*,#14384,.F.);
#19193=ORIENTED_EDGE('',*,*,#14458,.F.);
#19194=ORIENTED_EDGE('',*,*,#14577,.F.);
#19195=ORIENTED_EDGE('',*,*,#14046,.F.);
#19196=ORIENTED_EDGE('',*,*,#14047,.F.);
#19197=ORIENTED_EDGE('',*,*,#14577,.T.);
#19198=ORIENTED_EDGE('',*,*,#14457,.F.);
#19199=ORIENTED_EDGE('',*,*,#14578,.F.);
#19200=ORIENTED_EDGE('',*,*,#14048,.F.);
#19201=ORIENTED_EDGE('',*,*,#14578,.T.);
#19202=ORIENTED_EDGE('',*,*,#14456,.F.);
#19203=ORIENTED_EDGE('',*,*,#14054,.F.);
#19204=ORIENTED_EDGE('',*,*,#13804,.F.);
#19205=ORIENTED_EDGE('',*,*,#14053,.T.);
#19206=ORIENTED_EDGE('',*,*,#14382,.F.);
#19207=ORIENTED_EDGE('',*,*,#14579,.F.);
#19208=ORIENTED_EDGE('',*,*,#13805,.F.);
#19209=ORIENTED_EDGE('',*,*,#14579,.T.);
#19210=ORIENTED_EDGE('',*,*,#14381,.F.);
#19211=ORIENTED_EDGE('',*,*,#14580,.F.);
#19212=ORIENTED_EDGE('',*,*,#13806,.F.);
#19213=ORIENTED_EDGE('',*,*,#14580,.T.);
#19214=ORIENTED_EDGE('',*,*,#14380,.F.);
#19215=ORIENTED_EDGE('',*,*,#14581,.F.);
#19216=ORIENTED_EDGE('',*,*,#13807,.F.);
#19217=ORIENTED_EDGE('',*,*,#14581,.T.);
#19218=ORIENTED_EDGE('',*,*,#14379,.F.);
#19219=ORIENTED_EDGE('',*,*,#14582,.F.);
#19220=ORIENTED_EDGE('',*,*,#13808,.F.);
#19221=ORIENTED_EDGE('',*,*,#14582,.T.);
#19222=ORIENTED_EDGE('',*,*,#14378,.F.);
#19223=ORIENTED_EDGE('',*,*,#14583,.F.);
#19224=ORIENTED_EDGE('',*,*,#13809,.F.);
#19225=ORIENTED_EDGE('',*,*,#14583,.T.);
#19226=ORIENTED_EDGE('',*,*,#14377,.F.);
#19227=ORIENTED_EDGE('',*,*,#14584,.F.);
#19228=ORIENTED_EDGE('',*,*,#13810,.F.);
#19229=ORIENTED_EDGE('',*,*,#14584,.T.);
#19230=ORIENTED_EDGE('',*,*,#14376,.F.);
#19231=ORIENTED_EDGE('',*,*,#14585,.F.);
#19232=ORIENTED_EDGE('',*,*,#13811,.F.);
#19233=ORIENTED_EDGE('',*,*,#14585,.T.);
#19234=ORIENTED_EDGE('',*,*,#14375,.F.);
#19235=ORIENTED_EDGE('',*,*,#14586,.F.);
#19236=ORIENTED_EDGE('',*,*,#13812,.F.);
#19237=ORIENTED_EDGE('',*,*,#14586,.T.);
#19238=ORIENTED_EDGE('',*,*,#14374,.F.);
#19239=ORIENTED_EDGE('',*,*,#14587,.F.);
#19240=ORIENTED_EDGE('',*,*,#13813,.F.);
#19241=ORIENTED_EDGE('',*,*,#14587,.T.);
#19242=ORIENTED_EDGE('',*,*,#14373,.F.);
#19243=ORIENTED_EDGE('',*,*,#14588,.F.);
#19244=ORIENTED_EDGE('',*,*,#13814,.F.);
#19245=ORIENTED_EDGE('',*,*,#14588,.T.);
#19246=ORIENTED_EDGE('',*,*,#14372,.F.);
#19247=ORIENTED_EDGE('',*,*,#14589,.F.);
#19248=ORIENTED_EDGE('',*,*,#13815,.F.);
#19249=ORIENTED_EDGE('',*,*,#14589,.T.);
#19250=ORIENTED_EDGE('',*,*,#14371,.F.);
#19251=ORIENTED_EDGE('',*,*,#14590,.F.);
#19252=ORIENTED_EDGE('',*,*,#13816,.F.);
#19253=ORIENTED_EDGE('',*,*,#14590,.T.);
#19254=ORIENTED_EDGE('',*,*,#14370,.F.);
#19255=ORIENTED_EDGE('',*,*,#14591,.F.);
#19256=ORIENTED_EDGE('',*,*,#13817,.F.);
#19257=ORIENTED_EDGE('',*,*,#14591,.T.);
#19258=ORIENTED_EDGE('',*,*,#14369,.F.);
#19259=ORIENTED_EDGE('',*,*,#14592,.F.);
#19260=ORIENTED_EDGE('',*,*,#14172,.F.);
#19261=ORIENTED_EDGE('',*,*,#13818,.F.);
#19262=ORIENTED_EDGE('',*,*,#14592,.T.);
#19263=ORIENTED_EDGE('',*,*,#14368,.F.);
#19264=ORIENTED_EDGE('',*,*,#14459,.F.);
#19265=ORIENTED_EDGE('',*,*,#14593,.F.);
#19266=ORIENTED_EDGE('',*,*,#14173,.F.);
#19267=ORIENTED_EDGE('',*,*,#14593,.T.);
#19268=ORIENTED_EDGE('',*,*,#14461,.F.);
#19269=ORIENTED_EDGE('',*,*,#14177,.F.);
#19270=ORIENTED_EDGE('',*,*,#13820,.F.);
#19271=ORIENTED_EDGE('',*,*,#14171,.F.);
#19272=ORIENTED_EDGE('',*,*,#14176,.T.);
#19273=ORIENTED_EDGE('',*,*,#14460,.F.);
#19274=ORIENTED_EDGE('',*,*,#14366,.F.);
#19275=ORIENTED_EDGE('',*,*,#14594,.F.);
#19276=ORIENTED_EDGE('',*,*,#13821,.F.);
#19277=ORIENTED_EDGE('',*,*,#14594,.T.);
#19278=ORIENTED_EDGE('',*,*,#14365,.F.);
#19279=ORIENTED_EDGE('',*,*,#14464,.F.);
#19280=ORIENTED_EDGE('',*,*,#14595,.F.);
#19281=ORIENTED_EDGE('',*,*,#14035,.F.);
#19282=ORIENTED_EDGE('',*,*,#14036,.F.);
#19283=ORIENTED_EDGE('',*,*,#14595,.T.);
#19284=ORIENTED_EDGE('',*,*,#14463,.F.);
#19285=ORIENTED_EDGE('',*,*,#14596,.F.);
#19286=ORIENTED_EDGE('',*,*,#14037,.F.);
#19287=ORIENTED_EDGE('',*,*,#14596,.T.);
#19288=ORIENTED_EDGE('',*,*,#14462,.F.);
#19289=ORIENTED_EDGE('',*,*,#14043,.F.);
#19290=ORIENTED_EDGE('',*,*,#13824,.F.);
#19291=ORIENTED_EDGE('',*,*,#14042,.T.);
#19292=ORIENTED_EDGE('',*,*,#14363,.F.);
#19293=ORIENTED_EDGE('',*,*,#14597,.F.);
#19294=ORIENTED_EDGE('',*,*,#13825,.F.);
#19295=ORIENTED_EDGE('',*,*,#14597,.T.);
#19296=ORIENTED_EDGE('',*,*,#14362,.F.);
#19297=ORIENTED_EDGE('',*,*,#14598,.F.);
#19298=ORIENTED_EDGE('',*,*,#13826,.F.);
#19299=ORIENTED_EDGE('',*,*,#14598,.T.);
#19300=ORIENTED_EDGE('',*,*,#14361,.F.);
#19301=ORIENTED_EDGE('',*,*,#14599,.F.);
#19302=ORIENTED_EDGE('',*,*,#13827,.F.);
#19303=ORIENTED_EDGE('',*,*,#14599,.T.);
#19304=ORIENTED_EDGE('',*,*,#14360,.F.);
#19305=ORIENTED_EDGE('',*,*,#14600,.F.);
#19306=ORIENTED_EDGE('',*,*,#13828,.F.);
#19307=ORIENTED_EDGE('',*,*,#14600,.T.);
#19308=ORIENTED_EDGE('',*,*,#14359,.F.);
#19309=ORIENTED_EDGE('',*,*,#14601,.F.);
#19310=ORIENTED_EDGE('',*,*,#13829,.F.);
#19311=ORIENTED_EDGE('',*,*,#14601,.T.);
#19312=ORIENTED_EDGE('',*,*,#14358,.F.);
#19313=ORIENTED_EDGE('',*,*,#14602,.F.);
#19314=ORIENTED_EDGE('',*,*,#13830,.F.);
#19315=ORIENTED_EDGE('',*,*,#14602,.T.);
#19316=ORIENTED_EDGE('',*,*,#14357,.F.);
#19317=ORIENTED_EDGE('',*,*,#14603,.F.);
#19318=ORIENTED_EDGE('',*,*,#13831,.F.);
#19319=ORIENTED_EDGE('',*,*,#14603,.T.);
#19320=ORIENTED_EDGE('',*,*,#14356,.F.);
#19321=ORIENTED_EDGE('',*,*,#14604,.F.);
#19322=ORIENTED_EDGE('',*,*,#13832,.F.);
#19323=ORIENTED_EDGE('',*,*,#14604,.T.);
#19324=ORIENTED_EDGE('',*,*,#14355,.F.);
#19325=ORIENTED_EDGE('',*,*,#14605,.F.);
#19326=ORIENTED_EDGE('',*,*,#13833,.F.);
#19327=ORIENTED_EDGE('',*,*,#14605,.T.);
#19328=ORIENTED_EDGE('',*,*,#14354,.F.);
#19329=ORIENTED_EDGE('',*,*,#14606,.F.);
#19330=ORIENTED_EDGE('',*,*,#13834,.F.);
#19331=ORIENTED_EDGE('',*,*,#14606,.T.);
#19332=ORIENTED_EDGE('',*,*,#14353,.F.);
#19333=ORIENTED_EDGE('',*,*,#14607,.F.);
#19334=ORIENTED_EDGE('',*,*,#13835,.F.);
#19335=ORIENTED_EDGE('',*,*,#14607,.T.);
#19336=ORIENTED_EDGE('',*,*,#14352,.F.);
#19337=ORIENTED_EDGE('',*,*,#14608,.F.);
#19338=ORIENTED_EDGE('',*,*,#13836,.F.);
#19339=ORIENTED_EDGE('',*,*,#14608,.T.);
#19340=ORIENTED_EDGE('',*,*,#14351,.F.);
#19341=ORIENTED_EDGE('',*,*,#14609,.F.);
#19342=ORIENTED_EDGE('',*,*,#13837,.F.);
#19343=ORIENTED_EDGE('',*,*,#14609,.T.);
#19344=ORIENTED_EDGE('',*,*,#14350,.F.);
#19345=ORIENTED_EDGE('',*,*,#14610,.F.);
#19346=ORIENTED_EDGE('',*,*,#14162,.F.);
#19347=ORIENTED_EDGE('',*,*,#13838,.F.);
#19348=ORIENTED_EDGE('',*,*,#14610,.T.);
#19349=ORIENTED_EDGE('',*,*,#14349,.F.);
#19350=ORIENTED_EDGE('',*,*,#14465,.F.);
#19351=ORIENTED_EDGE('',*,*,#14611,.F.);
#19352=ORIENTED_EDGE('',*,*,#14163,.F.);
#19353=ORIENTED_EDGE('',*,*,#14611,.T.);
#19354=ORIENTED_EDGE('',*,*,#14467,.F.);
#19355=ORIENTED_EDGE('',*,*,#14167,.F.);
#19356=ORIENTED_EDGE('',*,*,#13840,.F.);
#19357=ORIENTED_EDGE('',*,*,#14161,.F.);
#19358=ORIENTED_EDGE('',*,*,#14166,.T.);
#19359=ORIENTED_EDGE('',*,*,#14466,.F.);
#19360=ORIENTED_EDGE('',*,*,#14347,.F.);
#19361=ORIENTED_EDGE('',*,*,#14612,.F.);
#19362=ORIENTED_EDGE('',*,*,#13841,.F.);
#19363=ORIENTED_EDGE('',*,*,#14612,.T.);
#19364=ORIENTED_EDGE('',*,*,#14346,.F.);
#19365=ORIENTED_EDGE('',*,*,#14470,.F.);
#19366=ORIENTED_EDGE('',*,*,#14613,.F.);
#19367=ORIENTED_EDGE('',*,*,#14024,.F.);
#19368=ORIENTED_EDGE('',*,*,#14025,.F.);
#19369=ORIENTED_EDGE('',*,*,#14613,.T.);
#19370=ORIENTED_EDGE('',*,*,#14469,.F.);
#19371=ORIENTED_EDGE('',*,*,#14614,.F.);
#19372=ORIENTED_EDGE('',*,*,#14026,.F.);
#19373=ORIENTED_EDGE('',*,*,#14614,.T.);
#19374=ORIENTED_EDGE('',*,*,#14468,.F.);
#19375=ORIENTED_EDGE('',*,*,#14032,.F.);
#19376=ORIENTED_EDGE('',*,*,#13844,.F.);
#19377=ORIENTED_EDGE('',*,*,#14031,.T.);
#19378=ORIENTED_EDGE('',*,*,#14344,.F.);
#19379=ORIENTED_EDGE('',*,*,#14615,.F.);
#19380=ORIENTED_EDGE('',*,*,#13845,.F.);
#19381=ORIENTED_EDGE('',*,*,#14615,.T.);
#19382=ORIENTED_EDGE('',*,*,#14343,.F.);
#19383=ORIENTED_EDGE('',*,*,#14616,.F.);
#19384=ORIENTED_EDGE('',*,*,#13846,.F.);
#19385=ORIENTED_EDGE('',*,*,#14616,.T.);
#19386=ORIENTED_EDGE('',*,*,#14342,.F.);
#19387=ORIENTED_EDGE('',*,*,#14617,.F.);
#19388=ORIENTED_EDGE('',*,*,#13847,.F.);
#19389=ORIENTED_EDGE('',*,*,#14617,.T.);
#19390=ORIENTED_EDGE('',*,*,#14341,.F.);
#19391=ORIENTED_EDGE('',*,*,#14618,.F.);
#19392=ORIENTED_EDGE('',*,*,#13848,.F.);
#19393=ORIENTED_EDGE('',*,*,#14618,.T.);
#19394=ORIENTED_EDGE('',*,*,#14340,.F.);
#19395=ORIENTED_EDGE('',*,*,#14619,.F.);
#19396=ORIENTED_EDGE('',*,*,#13849,.F.);
#19397=ORIENTED_EDGE('',*,*,#14619,.T.);
#19398=ORIENTED_EDGE('',*,*,#14339,.F.);
#19399=ORIENTED_EDGE('',*,*,#14620,.F.);
#19400=ORIENTED_EDGE('',*,*,#13850,.F.);
#19401=ORIENTED_EDGE('',*,*,#14620,.T.);
#19402=ORIENTED_EDGE('',*,*,#14338,.F.);
#19403=ORIENTED_EDGE('',*,*,#14621,.F.);
#19404=ORIENTED_EDGE('',*,*,#13851,.F.);
#19405=ORIENTED_EDGE('',*,*,#14621,.T.);
#19406=ORIENTED_EDGE('',*,*,#14337,.F.);
#19407=ORIENTED_EDGE('',*,*,#14622,.F.);
#19408=ORIENTED_EDGE('',*,*,#13852,.F.);
#19409=ORIENTED_EDGE('',*,*,#14622,.T.);
#19410=ORIENTED_EDGE('',*,*,#14336,.F.);
#19411=ORIENTED_EDGE('',*,*,#14623,.F.);
#19412=ORIENTED_EDGE('',*,*,#13853,.F.);
#19413=ORIENTED_EDGE('',*,*,#14623,.T.);
#19414=ORIENTED_EDGE('',*,*,#14335,.F.);
#19415=ORIENTED_EDGE('',*,*,#14624,.F.);
#19416=ORIENTED_EDGE('',*,*,#13854,.F.);
#19417=ORIENTED_EDGE('',*,*,#14624,.T.);
#19418=ORIENTED_EDGE('',*,*,#14334,.F.);
#19419=ORIENTED_EDGE('',*,*,#14625,.F.);
#19420=ORIENTED_EDGE('',*,*,#13855,.F.);
#19421=ORIENTED_EDGE('',*,*,#14625,.T.);
#19422=ORIENTED_EDGE('',*,*,#14333,.F.);
#19423=ORIENTED_EDGE('',*,*,#14626,.F.);
#19424=ORIENTED_EDGE('',*,*,#13856,.F.);
#19425=ORIENTED_EDGE('',*,*,#14626,.T.);
#19426=ORIENTED_EDGE('',*,*,#14332,.F.);
#19427=ORIENTED_EDGE('',*,*,#14627,.F.);
#19428=ORIENTED_EDGE('',*,*,#13857,.F.);
#19429=ORIENTED_EDGE('',*,*,#14627,.T.);
#19430=ORIENTED_EDGE('',*,*,#14331,.F.);
#19431=ORIENTED_EDGE('',*,*,#14628,.F.);
#19432=ORIENTED_EDGE('',*,*,#14152,.F.);
#19433=ORIENTED_EDGE('',*,*,#13858,.F.);
#19434=ORIENTED_EDGE('',*,*,#14628,.T.);
#19435=ORIENTED_EDGE('',*,*,#14330,.F.);
#19436=ORIENTED_EDGE('',*,*,#14471,.F.);
#19437=ORIENTED_EDGE('',*,*,#14629,.F.);
#19438=ORIENTED_EDGE('',*,*,#14153,.F.);
#19439=ORIENTED_EDGE('',*,*,#14629,.T.);
#19440=ORIENTED_EDGE('',*,*,#14473,.F.);
#19441=ORIENTED_EDGE('',*,*,#14157,.F.);
#19442=ORIENTED_EDGE('',*,*,#13860,.F.);
#19443=ORIENTED_EDGE('',*,*,#14151,.F.);
#19444=ORIENTED_EDGE('',*,*,#14156,.T.);
#19445=ORIENTED_EDGE('',*,*,#14472,.F.);
#19446=ORIENTED_EDGE('',*,*,#14328,.F.);
#19447=ORIENTED_EDGE('',*,*,#14630,.F.);
#19448=ORIENTED_EDGE('',*,*,#13861,.F.);
#19449=ORIENTED_EDGE('',*,*,#14630,.T.);
#19450=ORIENTED_EDGE('',*,*,#14327,.F.);
#19451=ORIENTED_EDGE('',*,*,#14476,.F.);
#19452=ORIENTED_EDGE('',*,*,#14631,.F.);
#19453=ORIENTED_EDGE('',*,*,#14013,.F.);
#19454=ORIENTED_EDGE('',*,*,#14014,.F.);
#19455=ORIENTED_EDGE('',*,*,#14631,.T.);
#19456=ORIENTED_EDGE('',*,*,#14475,.F.);
#19457=ORIENTED_EDGE('',*,*,#14632,.F.);
#19458=ORIENTED_EDGE('',*,*,#14015,.F.);
#19459=ORIENTED_EDGE('',*,*,#14632,.T.);
#19460=ORIENTED_EDGE('',*,*,#14474,.F.);
#19461=ORIENTED_EDGE('',*,*,#14021,.F.);
#19462=ORIENTED_EDGE('',*,*,#13864,.F.);
#19463=ORIENTED_EDGE('',*,*,#14020,.T.);
#19464=ORIENTED_EDGE('',*,*,#14325,.F.);
#19465=ORIENTED_EDGE('',*,*,#14633,.F.);
#19466=ORIENTED_EDGE('',*,*,#13865,.F.);
#19467=ORIENTED_EDGE('',*,*,#14633,.T.);
#19468=ORIENTED_EDGE('',*,*,#14324,.F.);
#19469=ORIENTED_EDGE('',*,*,#14634,.F.);
#19470=ORIENTED_EDGE('',*,*,#13866,.F.);
#19471=ORIENTED_EDGE('',*,*,#14634,.T.);
#19472=ORIENTED_EDGE('',*,*,#14323,.F.);
#19473=ORIENTED_EDGE('',*,*,#14635,.F.);
#19474=ORIENTED_EDGE('',*,*,#13867,.F.);
#19475=ORIENTED_EDGE('',*,*,#14635,.T.);
#19476=ORIENTED_EDGE('',*,*,#14322,.F.);
#19477=ORIENTED_EDGE('',*,*,#14636,.F.);
#19478=ORIENTED_EDGE('',*,*,#13868,.F.);
#19479=ORIENTED_EDGE('',*,*,#14636,.T.);
#19480=ORIENTED_EDGE('',*,*,#14321,.F.);
#19481=ORIENTED_EDGE('',*,*,#14637,.F.);
#19482=ORIENTED_EDGE('',*,*,#13869,.F.);
#19483=ORIENTED_EDGE('',*,*,#14637,.T.);
#19484=ORIENTED_EDGE('',*,*,#14320,.F.);
#19485=ORIENTED_EDGE('',*,*,#14638,.F.);
#19486=ORIENTED_EDGE('',*,*,#13870,.F.);
#19487=ORIENTED_EDGE('',*,*,#14638,.T.);
#19488=ORIENTED_EDGE('',*,*,#14319,.F.);
#19489=ORIENTED_EDGE('',*,*,#14639,.F.);
#19490=ORIENTED_EDGE('',*,*,#13871,.F.);
#19491=ORIENTED_EDGE('',*,*,#14639,.T.);
#19492=ORIENTED_EDGE('',*,*,#14318,.F.);
#19493=ORIENTED_EDGE('',*,*,#14640,.F.);
#19494=ORIENTED_EDGE('',*,*,#13872,.F.);
#19495=ORIENTED_EDGE('',*,*,#14640,.T.);
#19496=ORIENTED_EDGE('',*,*,#14317,.F.);
#19497=ORIENTED_EDGE('',*,*,#14641,.F.);
#19498=ORIENTED_EDGE('',*,*,#13873,.F.);
#19499=ORIENTED_EDGE('',*,*,#14641,.T.);
#19500=ORIENTED_EDGE('',*,*,#14316,.F.);
#19501=ORIENTED_EDGE('',*,*,#14642,.F.);
#19502=ORIENTED_EDGE('',*,*,#13874,.F.);
#19503=ORIENTED_EDGE('',*,*,#14642,.T.);
#19504=ORIENTED_EDGE('',*,*,#14315,.F.);
#19505=ORIENTED_EDGE('',*,*,#14643,.F.);
#19506=ORIENTED_EDGE('',*,*,#13875,.F.);
#19507=ORIENTED_EDGE('',*,*,#14643,.T.);
#19508=ORIENTED_EDGE('',*,*,#14314,.F.);
#19509=ORIENTED_EDGE('',*,*,#14644,.F.);
#19510=ORIENTED_EDGE('',*,*,#13876,.F.);
#19511=ORIENTED_EDGE('',*,*,#14644,.T.);
#19512=ORIENTED_EDGE('',*,*,#14313,.F.);
#19513=ORIENTED_EDGE('',*,*,#14645,.F.);
#19514=ORIENTED_EDGE('',*,*,#13877,.F.);
#19515=ORIENTED_EDGE('',*,*,#14645,.T.);
#19516=ORIENTED_EDGE('',*,*,#14312,.F.);
#19517=ORIENTED_EDGE('',*,*,#14646,.F.);
#19518=ORIENTED_EDGE('',*,*,#14142,.F.);
#19519=ORIENTED_EDGE('',*,*,#13878,.F.);
#19520=ORIENTED_EDGE('',*,*,#14646,.T.);
#19521=ORIENTED_EDGE('',*,*,#14311,.F.);
#19522=ORIENTED_EDGE('',*,*,#14477,.F.);
#19523=ORIENTED_EDGE('',*,*,#14647,.F.);
#19524=ORIENTED_EDGE('',*,*,#14143,.F.);
#19525=ORIENTED_EDGE('',*,*,#14647,.T.);
#19526=ORIENTED_EDGE('',*,*,#14479,.F.);
#19527=ORIENTED_EDGE('',*,*,#14147,.F.);
#19528=ORIENTED_EDGE('',*,*,#13880,.F.);
#19529=ORIENTED_EDGE('',*,*,#14141,.F.);
#19530=ORIENTED_EDGE('',*,*,#14146,.T.);
#19531=ORIENTED_EDGE('',*,*,#14478,.F.);
#19532=ORIENTED_EDGE('',*,*,#14309,.F.);
#19533=ORIENTED_EDGE('',*,*,#14648,.F.);
#19534=ORIENTED_EDGE('',*,*,#13881,.F.);
#19535=ORIENTED_EDGE('',*,*,#14648,.T.);
#19536=ORIENTED_EDGE('',*,*,#14308,.F.);
#19537=ORIENTED_EDGE('',*,*,#14482,.F.);
#19538=ORIENTED_EDGE('',*,*,#14649,.F.);
#19539=ORIENTED_EDGE('',*,*,#14002,.F.);
#19540=ORIENTED_EDGE('',*,*,#14003,.F.);
#19541=ORIENTED_EDGE('',*,*,#14649,.T.);
#19542=ORIENTED_EDGE('',*,*,#14481,.F.);
#19543=ORIENTED_EDGE('',*,*,#14650,.F.);
#19544=ORIENTED_EDGE('',*,*,#14004,.F.);
#19545=ORIENTED_EDGE('',*,*,#14650,.T.);
#19546=ORIENTED_EDGE('',*,*,#14480,.F.);
#19547=ORIENTED_EDGE('',*,*,#14010,.F.);
#19548=ORIENTED_EDGE('',*,*,#13884,.F.);
#19549=ORIENTED_EDGE('',*,*,#14009,.T.);
#19550=ORIENTED_EDGE('',*,*,#14306,.F.);
#19551=ORIENTED_EDGE('',*,*,#14651,.F.);
#19552=ORIENTED_EDGE('',*,*,#13885,.F.);
#19553=ORIENTED_EDGE('',*,*,#14651,.T.);
#19554=ORIENTED_EDGE('',*,*,#14305,.F.);
#19555=ORIENTED_EDGE('',*,*,#14652,.F.);
#19556=ORIENTED_EDGE('',*,*,#13886,.F.);
#19557=ORIENTED_EDGE('',*,*,#14652,.T.);
#19558=ORIENTED_EDGE('',*,*,#14304,.F.);
#19559=ORIENTED_EDGE('',*,*,#14653,.F.);
#19560=ORIENTED_EDGE('',*,*,#13887,.F.);
#19561=ORIENTED_EDGE('',*,*,#14653,.T.);
#19562=ORIENTED_EDGE('',*,*,#14303,.F.);
#19563=ORIENTED_EDGE('',*,*,#14654,.F.);
#19564=ORIENTED_EDGE('',*,*,#13888,.F.);
#19565=ORIENTED_EDGE('',*,*,#14654,.T.);
#19566=ORIENTED_EDGE('',*,*,#14302,.F.);
#19567=ORIENTED_EDGE('',*,*,#14655,.F.);
#19568=ORIENTED_EDGE('',*,*,#13889,.F.);
#19569=ORIENTED_EDGE('',*,*,#14655,.T.);
#19570=ORIENTED_EDGE('',*,*,#14301,.F.);
#19571=ORIENTED_EDGE('',*,*,#14656,.F.);
#19572=ORIENTED_EDGE('',*,*,#13890,.F.);
#19573=ORIENTED_EDGE('',*,*,#14656,.T.);
#19574=ORIENTED_EDGE('',*,*,#14300,.F.);
#19575=ORIENTED_EDGE('',*,*,#14657,.F.);
#19576=ORIENTED_EDGE('',*,*,#13891,.F.);
#19577=ORIENTED_EDGE('',*,*,#14657,.T.);
#19578=ORIENTED_EDGE('',*,*,#14299,.F.);
#19579=ORIENTED_EDGE('',*,*,#14658,.F.);
#19580=ORIENTED_EDGE('',*,*,#13892,.F.);
#19581=ORIENTED_EDGE('',*,*,#14658,.T.);
#19582=ORIENTED_EDGE('',*,*,#14298,.F.);
#19583=ORIENTED_EDGE('',*,*,#14659,.F.);
#19584=ORIENTED_EDGE('',*,*,#13893,.F.);
#19585=ORIENTED_EDGE('',*,*,#14659,.T.);
#19586=ORIENTED_EDGE('',*,*,#14297,.F.);
#19587=ORIENTED_EDGE('',*,*,#14660,.F.);
#19588=ORIENTED_EDGE('',*,*,#13894,.F.);
#19589=ORIENTED_EDGE('',*,*,#14660,.T.);
#19590=ORIENTED_EDGE('',*,*,#14296,.F.);
#19591=ORIENTED_EDGE('',*,*,#14661,.F.);
#19592=ORIENTED_EDGE('',*,*,#13895,.F.);
#19593=ORIENTED_EDGE('',*,*,#14661,.T.);
#19594=ORIENTED_EDGE('',*,*,#14295,.F.);
#19595=ORIENTED_EDGE('',*,*,#14662,.F.);
#19596=ORIENTED_EDGE('',*,*,#13896,.F.);
#19597=ORIENTED_EDGE('',*,*,#14662,.T.);
#19598=ORIENTED_EDGE('',*,*,#14294,.F.);
#19599=ORIENTED_EDGE('',*,*,#14663,.F.);
#19600=ORIENTED_EDGE('',*,*,#13897,.F.);
#19601=ORIENTED_EDGE('',*,*,#14663,.T.);
#19602=ORIENTED_EDGE('',*,*,#14293,.F.);
#19603=ORIENTED_EDGE('',*,*,#14664,.F.);
#19604=ORIENTED_EDGE('',*,*,#14132,.F.);
#19605=ORIENTED_EDGE('',*,*,#13898,.F.);
#19606=ORIENTED_EDGE('',*,*,#14664,.T.);
#19607=ORIENTED_EDGE('',*,*,#14292,.F.);
#19608=ORIENTED_EDGE('',*,*,#14483,.F.);
#19609=ORIENTED_EDGE('',*,*,#14665,.F.);
#19610=ORIENTED_EDGE('',*,*,#14133,.F.);
#19611=ORIENTED_EDGE('',*,*,#14665,.T.);
#19612=ORIENTED_EDGE('',*,*,#14485,.F.);
#19613=ORIENTED_EDGE('',*,*,#14137,.F.);
#19614=ORIENTED_EDGE('',*,*,#13900,.F.);
#19615=ORIENTED_EDGE('',*,*,#14131,.F.);
#19616=ORIENTED_EDGE('',*,*,#14136,.T.);
#19617=ORIENTED_EDGE('',*,*,#14484,.F.);
#19618=ORIENTED_EDGE('',*,*,#14290,.F.);
#19619=ORIENTED_EDGE('',*,*,#14666,.F.);
#19620=ORIENTED_EDGE('',*,*,#13901,.F.);
#19621=ORIENTED_EDGE('',*,*,#14666,.T.);
#19622=ORIENTED_EDGE('',*,*,#14289,.F.);
#19623=ORIENTED_EDGE('',*,*,#14488,.F.);
#19624=ORIENTED_EDGE('',*,*,#14667,.F.);
#19625=ORIENTED_EDGE('',*,*,#13991,.F.);
#19626=ORIENTED_EDGE('',*,*,#13992,.F.);
#19627=ORIENTED_EDGE('',*,*,#14667,.T.);
#19628=ORIENTED_EDGE('',*,*,#14487,.F.);
#19629=ORIENTED_EDGE('',*,*,#14668,.F.);
#19630=ORIENTED_EDGE('',*,*,#13993,.F.);
#19631=ORIENTED_EDGE('',*,*,#14668,.T.);
#19632=ORIENTED_EDGE('',*,*,#14486,.F.);
#19633=ORIENTED_EDGE('',*,*,#13999,.F.);
#19634=ORIENTED_EDGE('',*,*,#13904,.F.);
#19635=ORIENTED_EDGE('',*,*,#13998,.T.);
#19636=ORIENTED_EDGE('',*,*,#14287,.F.);
#19637=ORIENTED_EDGE('',*,*,#14669,.F.);
#19638=ORIENTED_EDGE('',*,*,#13905,.F.);
#19639=ORIENTED_EDGE('',*,*,#14669,.T.);
#19640=ORIENTED_EDGE('',*,*,#14286,.F.);
#19641=ORIENTED_EDGE('',*,*,#14670,.F.);
#19642=ORIENTED_EDGE('',*,*,#13906,.F.);
#19643=ORIENTED_EDGE('',*,*,#14670,.T.);
#19644=ORIENTED_EDGE('',*,*,#14285,.F.);
#19645=ORIENTED_EDGE('',*,*,#14671,.F.);
#19646=ORIENTED_EDGE('',*,*,#13907,.F.);
#19647=ORIENTED_EDGE('',*,*,#14671,.T.);
#19648=ORIENTED_EDGE('',*,*,#14284,.F.);
#19649=ORIENTED_EDGE('',*,*,#14672,.F.);
#19650=ORIENTED_EDGE('',*,*,#13908,.F.);
#19651=ORIENTED_EDGE('',*,*,#14672,.T.);
#19652=ORIENTED_EDGE('',*,*,#14283,.F.);
#19653=ORIENTED_EDGE('',*,*,#14673,.F.);
#19654=ORIENTED_EDGE('',*,*,#13909,.F.);
#19655=ORIENTED_EDGE('',*,*,#14673,.T.);
#19656=ORIENTED_EDGE('',*,*,#14282,.F.);
#19657=ORIENTED_EDGE('',*,*,#14674,.F.);
#19658=ORIENTED_EDGE('',*,*,#13910,.F.);
#19659=ORIENTED_EDGE('',*,*,#14674,.T.);
#19660=ORIENTED_EDGE('',*,*,#14281,.F.);
#19661=ORIENTED_EDGE('',*,*,#14675,.F.);
#19662=ORIENTED_EDGE('',*,*,#13911,.F.);
#19663=ORIENTED_EDGE('',*,*,#14675,.T.);
#19664=ORIENTED_EDGE('',*,*,#14280,.F.);
#19665=ORIENTED_EDGE('',*,*,#14676,.F.);
#19666=ORIENTED_EDGE('',*,*,#13912,.F.);
#19667=ORIENTED_EDGE('',*,*,#14676,.T.);
#19668=ORIENTED_EDGE('',*,*,#14279,.F.);
#19669=ORIENTED_EDGE('',*,*,#14677,.F.);
#19670=ORIENTED_EDGE('',*,*,#13913,.F.);
#19671=ORIENTED_EDGE('',*,*,#14677,.T.);
#19672=ORIENTED_EDGE('',*,*,#14278,.F.);
#19673=ORIENTED_EDGE('',*,*,#14678,.F.);
#19674=ORIENTED_EDGE('',*,*,#13914,.F.);
#19675=ORIENTED_EDGE('',*,*,#14678,.T.);
#19676=ORIENTED_EDGE('',*,*,#14277,.F.);
#19677=ORIENTED_EDGE('',*,*,#14679,.F.);
#19678=ORIENTED_EDGE('',*,*,#13915,.F.);
#19679=ORIENTED_EDGE('',*,*,#14679,.T.);
#19680=ORIENTED_EDGE('',*,*,#14276,.F.);
#19681=ORIENTED_EDGE('',*,*,#14680,.F.);
#19682=ORIENTED_EDGE('',*,*,#13916,.F.);
#19683=ORIENTED_EDGE('',*,*,#14680,.T.);
#19684=ORIENTED_EDGE('',*,*,#14275,.F.);
#19685=ORIENTED_EDGE('',*,*,#14681,.F.);
#19686=ORIENTED_EDGE('',*,*,#13917,.F.);
#19687=ORIENTED_EDGE('',*,*,#14681,.T.);
#19688=ORIENTED_EDGE('',*,*,#14274,.F.);
#19689=ORIENTED_EDGE('',*,*,#14682,.F.);
#19690=ORIENTED_EDGE('',*,*,#14122,.F.);
#19691=ORIENTED_EDGE('',*,*,#13918,.F.);
#19692=ORIENTED_EDGE('',*,*,#14682,.T.);
#19693=ORIENTED_EDGE('',*,*,#14273,.F.);
#19694=ORIENTED_EDGE('',*,*,#14489,.F.);
#19695=ORIENTED_EDGE('',*,*,#14683,.F.);
#19696=ORIENTED_EDGE('',*,*,#14123,.F.);
#19697=ORIENTED_EDGE('',*,*,#14683,.T.);
#19698=ORIENTED_EDGE('',*,*,#14491,.F.);
#19699=ORIENTED_EDGE('',*,*,#14127,.F.);
#19700=ORIENTED_EDGE('',*,*,#13920,.F.);
#19701=ORIENTED_EDGE('',*,*,#14121,.F.);
#19702=ORIENTED_EDGE('',*,*,#14126,.T.);
#19703=ORIENTED_EDGE('',*,*,#14490,.F.);
#19704=ORIENTED_EDGE('',*,*,#14271,.F.);
#19705=ORIENTED_EDGE('',*,*,#14684,.F.);
#19706=ORIENTED_EDGE('',*,*,#13921,.F.);
#19707=ORIENTED_EDGE('',*,*,#14684,.T.);
#19708=ORIENTED_EDGE('',*,*,#14270,.F.);
#19709=ORIENTED_EDGE('',*,*,#14494,.F.);
#19710=ORIENTED_EDGE('',*,*,#14685,.F.);
#19711=ORIENTED_EDGE('',*,*,#13980,.F.);
#19712=ORIENTED_EDGE('',*,*,#13981,.F.);
#19713=ORIENTED_EDGE('',*,*,#14685,.T.);
#19714=ORIENTED_EDGE('',*,*,#14493,.F.);
#19715=ORIENTED_EDGE('',*,*,#14686,.F.);
#19716=ORIENTED_EDGE('',*,*,#13982,.F.);
#19717=ORIENTED_EDGE('',*,*,#14686,.T.);
#19718=ORIENTED_EDGE('',*,*,#14492,.F.);
#19719=ORIENTED_EDGE('',*,*,#13988,.F.);
#19720=ORIENTED_EDGE('',*,*,#13924,.F.);
#19721=ORIENTED_EDGE('',*,*,#13987,.T.);
#19722=ORIENTED_EDGE('',*,*,#14268,.F.);
#19723=ORIENTED_EDGE('',*,*,#14687,.F.);
#19724=ORIENTED_EDGE('',*,*,#13925,.F.);
#19725=ORIENTED_EDGE('',*,*,#14687,.T.);
#19726=ORIENTED_EDGE('',*,*,#14267,.F.);
#19727=ORIENTED_EDGE('',*,*,#14688,.F.);
#19728=ORIENTED_EDGE('',*,*,#13926,.F.);
#19729=ORIENTED_EDGE('',*,*,#14688,.T.);
#19730=ORIENTED_EDGE('',*,*,#14266,.F.);
#19731=ORIENTED_EDGE('',*,*,#14689,.F.);
#19732=ORIENTED_EDGE('',*,*,#13927,.F.);
#19733=ORIENTED_EDGE('',*,*,#14689,.T.);
#19734=ORIENTED_EDGE('',*,*,#14265,.F.);
#19735=ORIENTED_EDGE('',*,*,#14690,.F.);
#19736=ORIENTED_EDGE('',*,*,#13928,.F.);
#19737=ORIENTED_EDGE('',*,*,#14690,.T.);
#19738=ORIENTED_EDGE('',*,*,#14264,.F.);
#19739=ORIENTED_EDGE('',*,*,#14691,.F.);
#19740=ORIENTED_EDGE('',*,*,#13929,.F.);
#19741=ORIENTED_EDGE('',*,*,#14691,.T.);
#19742=ORIENTED_EDGE('',*,*,#14263,.F.);
#19743=ORIENTED_EDGE('',*,*,#14692,.F.);
#19744=ORIENTED_EDGE('',*,*,#13930,.F.);
#19745=ORIENTED_EDGE('',*,*,#14692,.T.);
#19746=ORIENTED_EDGE('',*,*,#14262,.F.);
#19747=ORIENTED_EDGE('',*,*,#14693,.F.);
#19748=ORIENTED_EDGE('',*,*,#13931,.F.);
#19749=ORIENTED_EDGE('',*,*,#14693,.T.);
#19750=ORIENTED_EDGE('',*,*,#14261,.F.);
#19751=ORIENTED_EDGE('',*,*,#14694,.F.);
#19752=ORIENTED_EDGE('',*,*,#13932,.F.);
#19753=ORIENTED_EDGE('',*,*,#14694,.T.);
#19754=ORIENTED_EDGE('',*,*,#14260,.F.);
#19755=ORIENTED_EDGE('',*,*,#14695,.F.);
#19756=ORIENTED_EDGE('',*,*,#13933,.F.);
#19757=ORIENTED_EDGE('',*,*,#14695,.T.);
#19758=ORIENTED_EDGE('',*,*,#14259,.F.);
#19759=ORIENTED_EDGE('',*,*,#14696,.F.);
#19760=ORIENTED_EDGE('',*,*,#13934,.F.);
#19761=ORIENTED_EDGE('',*,*,#14696,.T.);
#19762=ORIENTED_EDGE('',*,*,#14258,.F.);
#19763=ORIENTED_EDGE('',*,*,#14697,.F.);
#19764=ORIENTED_EDGE('',*,*,#13935,.F.);
#19765=ORIENTED_EDGE('',*,*,#14697,.T.);
#19766=ORIENTED_EDGE('',*,*,#14257,.F.);
#19767=ORIENTED_EDGE('',*,*,#14698,.F.);
#19768=ORIENTED_EDGE('',*,*,#13936,.F.);
#19769=ORIENTED_EDGE('',*,*,#14698,.T.);
#19770=ORIENTED_EDGE('',*,*,#14256,.F.);
#19771=ORIENTED_EDGE('',*,*,#14699,.F.);
#19772=ORIENTED_EDGE('',*,*,#13937,.F.);
#19773=ORIENTED_EDGE('',*,*,#14699,.T.);
#19774=ORIENTED_EDGE('',*,*,#14255,.F.);
#19775=ORIENTED_EDGE('',*,*,#14700,.F.);
#19776=ORIENTED_EDGE('',*,*,#14112,.F.);
#19777=ORIENTED_EDGE('',*,*,#13938,.F.);
#19778=ORIENTED_EDGE('',*,*,#14700,.T.);
#19779=ORIENTED_EDGE('',*,*,#14254,.F.);
#19780=ORIENTED_EDGE('',*,*,#14495,.F.);
#19781=ORIENTED_EDGE('',*,*,#14701,.F.);
#19782=ORIENTED_EDGE('',*,*,#14113,.F.);
#19783=ORIENTED_EDGE('',*,*,#14701,.T.);
#19784=ORIENTED_EDGE('',*,*,#14497,.F.);
#19785=ORIENTED_EDGE('',*,*,#14117,.F.);
#19786=ORIENTED_EDGE('',*,*,#13940,.F.);
#19787=ORIENTED_EDGE('',*,*,#14111,.F.);
#19788=ORIENTED_EDGE('',*,*,#14116,.T.);
#19789=ORIENTED_EDGE('',*,*,#14496,.F.);
#19790=ORIENTED_EDGE('',*,*,#14252,.F.);
#19791=ORIENTED_EDGE('',*,*,#14702,.F.);
#19792=ORIENTED_EDGE('',*,*,#13941,.F.);
#19793=ORIENTED_EDGE('',*,*,#14702,.T.);
#19794=ORIENTED_EDGE('',*,*,#14251,.F.);
#19795=ORIENTED_EDGE('',*,*,#14500,.F.);
#19796=ORIENTED_EDGE('',*,*,#14703,.F.);
#19797=ORIENTED_EDGE('',*,*,#13969,.F.);
#19798=ORIENTED_EDGE('',*,*,#13970,.F.);
#19799=ORIENTED_EDGE('',*,*,#14703,.T.);
#19800=ORIENTED_EDGE('',*,*,#14499,.F.);
#19801=ORIENTED_EDGE('',*,*,#14704,.F.);
#19802=ORIENTED_EDGE('',*,*,#13971,.F.);
#19803=ORIENTED_EDGE('',*,*,#14704,.T.);
#19804=ORIENTED_EDGE('',*,*,#14498,.F.);
#19805=ORIENTED_EDGE('',*,*,#13977,.F.);
#19806=ORIENTED_EDGE('',*,*,#13944,.F.);
#19807=ORIENTED_EDGE('',*,*,#13976,.T.);
#19808=ORIENTED_EDGE('',*,*,#14249,.F.);
#19809=ORIENTED_EDGE('',*,*,#14705,.F.);
#19810=ORIENTED_EDGE('',*,*,#13945,.F.);
#19811=ORIENTED_EDGE('',*,*,#14705,.T.);
#19812=ORIENTED_EDGE('',*,*,#14248,.F.);
#19813=ORIENTED_EDGE('',*,*,#14706,.F.);
#19814=ORIENTED_EDGE('',*,*,#13946,.F.);
#19815=ORIENTED_EDGE('',*,*,#14706,.T.);
#19816=ORIENTED_EDGE('',*,*,#14247,.F.);
#19817=ORIENTED_EDGE('',*,*,#14707,.F.);
#19818=ORIENTED_EDGE('',*,*,#13947,.F.);
#19819=ORIENTED_EDGE('',*,*,#14707,.T.);
#19820=ORIENTED_EDGE('',*,*,#14246,.F.);
#19821=ORIENTED_EDGE('',*,*,#14708,.F.);
#19822=ORIENTED_EDGE('',*,*,#13948,.F.);
#19823=ORIENTED_EDGE('',*,*,#14708,.T.);
#19824=ORIENTED_EDGE('',*,*,#14245,.F.);
#19825=ORIENTED_EDGE('',*,*,#14709,.F.);
#19826=ORIENTED_EDGE('',*,*,#13949,.F.);
#19827=ORIENTED_EDGE('',*,*,#14709,.T.);
#19828=ORIENTED_EDGE('',*,*,#14244,.F.);
#19829=ORIENTED_EDGE('',*,*,#14710,.F.);
#19830=ORIENTED_EDGE('',*,*,#13950,.F.);
#19831=ORIENTED_EDGE('',*,*,#14710,.T.);
#19832=ORIENTED_EDGE('',*,*,#14243,.F.);
#19833=ORIENTED_EDGE('',*,*,#14711,.F.);
#19834=ORIENTED_EDGE('',*,*,#13951,.F.);
#19835=ORIENTED_EDGE('',*,*,#14711,.T.);
#19836=ORIENTED_EDGE('',*,*,#14242,.F.);
#19837=ORIENTED_EDGE('',*,*,#14712,.F.);
#19838=ORIENTED_EDGE('',*,*,#13952,.F.);
#19839=ORIENTED_EDGE('',*,*,#14712,.T.);
#19840=ORIENTED_EDGE('',*,*,#14241,.F.);
#19841=ORIENTED_EDGE('',*,*,#14713,.F.);
#19842=ORIENTED_EDGE('',*,*,#13953,.F.);
#19843=ORIENTED_EDGE('',*,*,#14713,.T.);
#19844=ORIENTED_EDGE('',*,*,#14240,.F.);
#19845=ORIENTED_EDGE('',*,*,#14714,.F.);
#19846=ORIENTED_EDGE('',*,*,#13954,.F.);
#19847=ORIENTED_EDGE('',*,*,#14714,.T.);
#19848=ORIENTED_EDGE('',*,*,#14239,.F.);
#19849=ORIENTED_EDGE('',*,*,#14715,.F.);
#19850=ORIENTED_EDGE('',*,*,#13955,.F.);
#19851=ORIENTED_EDGE('',*,*,#14715,.T.);
#19852=ORIENTED_EDGE('',*,*,#14238,.F.);
#19853=ORIENTED_EDGE('',*,*,#14716,.F.);
#19854=ORIENTED_EDGE('',*,*,#13956,.F.);
#19855=ORIENTED_EDGE('',*,*,#14716,.T.);
#19856=ORIENTED_EDGE('',*,*,#14237,.F.);
#19857=ORIENTED_EDGE('',*,*,#14717,.F.);
#19858=ORIENTED_EDGE('',*,*,#13957,.F.);
#19859=ORIENTED_EDGE('',*,*,#14717,.T.);
#19860=ORIENTED_EDGE('',*,*,#14236,.F.);
#19861=ORIENTED_EDGE('',*,*,#14718,.F.);
#19862=ORIENTED_EDGE('',*,*,#14102,.F.);
#19863=ORIENTED_EDGE('',*,*,#13958,.F.);
#19864=ORIENTED_EDGE('',*,*,#14718,.T.);
#19865=ORIENTED_EDGE('',*,*,#14235,.F.);
#19866=ORIENTED_EDGE('',*,*,#14501,.F.);
#19867=ORIENTED_EDGE('',*,*,#14719,.F.);
#19868=ORIENTED_EDGE('',*,*,#14103,.F.);
#19869=ORIENTED_EDGE('',*,*,#14719,.T.);
#19870=ORIENTED_EDGE('',*,*,#14503,.F.);
#19871=ORIENTED_EDGE('',*,*,#14107,.F.);
#19872=ORIENTED_EDGE('',*,*,#13960,.F.);
#19873=ORIENTED_EDGE('',*,*,#14101,.F.);
#19874=ORIENTED_EDGE('',*,*,#14106,.T.);
#19875=ORIENTED_EDGE('',*,*,#14502,.F.);
#19876=ORIENTED_EDGE('',*,*,#14233,.F.);
#19877=ORIENTED_EDGE('',*,*,#14720,.F.);
#19878=ORIENTED_EDGE('',*,*,#13722,.F.);
#19879=ORIENTED_EDGE('',*,*,#14720,.T.);
#19880=ORIENTED_EDGE('',*,*,#14232,.F.);
#19881=ORIENTED_EDGE('',*,*,#14506,.F.);
#19882=ORIENTED_EDGE('',*,*,#14721,.F.);
#19883=ORIENTED_EDGE('',*,*,#13718,.F.);
#19884=ORIENTED_EDGE('',*,*,#13719,.F.);
#19885=ORIENTED_EDGE('',*,*,#14721,.T.);
#19886=ORIENTED_EDGE('',*,*,#14505,.F.);
#19887=ORIENTED_EDGE('',*,*,#14722,.F.);
#19888=ORIENTED_EDGE('',*,*,#13720,.F.);
#19889=ORIENTED_EDGE('',*,*,#14722,.T.);
#19890=ORIENTED_EDGE('',*,*,#14504,.F.);
#19891=ORIENTED_EDGE('',*,*,#13966,.F.);
#19892=ORIENTED_EDGE('',*,*,#13724,.F.);
#19893=ORIENTED_EDGE('',*,*,#13965,.T.);
#19894=ORIENTED_EDGE('',*,*,#14230,.F.);
#19895=ORIENTED_EDGE('',*,*,#14723,.F.);
#19896=ORIENTED_EDGE('',*,*,#13725,.F.);
#19897=ORIENTED_EDGE('',*,*,#14723,.T.);
#19898=ORIENTED_EDGE('',*,*,#14229,.F.);
#19899=ORIENTED_EDGE('',*,*,#14724,.F.);
#19900=ORIENTED_EDGE('',*,*,#13726,.F.);
#19901=ORIENTED_EDGE('',*,*,#14724,.T.);
#19902=ORIENTED_EDGE('',*,*,#14228,.F.);
#19903=ORIENTED_EDGE('',*,*,#14725,.F.);
#19904=ORIENTED_EDGE('',*,*,#13727,.F.);
#19905=ORIENTED_EDGE('',*,*,#14725,.T.);
#19906=ORIENTED_EDGE('',*,*,#14227,.F.);
#19907=ORIENTED_EDGE('',*,*,#14726,.F.);
#19908=ORIENTED_EDGE('',*,*,#13728,.F.);
#19909=ORIENTED_EDGE('',*,*,#14726,.T.);
#19910=ORIENTED_EDGE('',*,*,#14226,.F.);
#19911=ORIENTED_EDGE('',*,*,#14727,.F.);
#19912=ORIENTED_EDGE('',*,*,#13729,.F.);
#19913=ORIENTED_EDGE('',*,*,#14727,.T.);
#19914=ORIENTED_EDGE('',*,*,#14225,.F.);
#19915=ORIENTED_EDGE('',*,*,#14728,.F.);
#19916=ORIENTED_EDGE('',*,*,#13730,.F.);
#19917=ORIENTED_EDGE('',*,*,#14728,.T.);
#19918=ORIENTED_EDGE('',*,*,#14224,.F.);
#19919=ORIENTED_EDGE('',*,*,#14729,.F.);
#19920=ORIENTED_EDGE('',*,*,#13731,.F.);
#19921=ORIENTED_EDGE('',*,*,#14729,.T.);
#19922=ORIENTED_EDGE('',*,*,#14223,.F.);
#19923=ORIENTED_EDGE('',*,*,#14730,.F.);
#19924=ORIENTED_EDGE('',*,*,#13732,.F.);
#19925=ORIENTED_EDGE('',*,*,#14730,.T.);
#19926=ORIENTED_EDGE('',*,*,#14222,.F.);
#19927=ORIENTED_EDGE('',*,*,#14731,.F.);
#19928=ORIENTED_EDGE('',*,*,#13733,.F.);
#19929=ORIENTED_EDGE('',*,*,#14731,.T.);
#19930=ORIENTED_EDGE('',*,*,#14221,.F.);
#19931=ORIENTED_EDGE('',*,*,#14732,.F.);
#19932=ORIENTED_EDGE('',*,*,#13734,.F.);
#19933=ORIENTED_EDGE('',*,*,#14732,.T.);
#19934=ORIENTED_EDGE('',*,*,#14220,.F.);
#19935=ORIENTED_EDGE('',*,*,#14733,.F.);
#19936=ORIENTED_EDGE('',*,*,#13735,.F.);
#19937=ORIENTED_EDGE('',*,*,#14733,.T.);
#19938=ORIENTED_EDGE('',*,*,#14219,.F.);
#19939=ORIENTED_EDGE('',*,*,#14734,.F.);
#19940=ORIENTED_EDGE('',*,*,#13736,.F.);
#19941=ORIENTED_EDGE('',*,*,#14734,.T.);
#19942=ORIENTED_EDGE('',*,*,#14218,.F.);
#19943=ORIENTED_EDGE('',*,*,#14735,.F.);
#19944=ORIENTED_EDGE('',*,*,#13737,.F.);
#19945=ORIENTED_EDGE('',*,*,#14735,.T.);
#19946=ORIENTED_EDGE('',*,*,#14217,.F.);
#19947=ORIENTED_EDGE('',*,*,#14736,.F.);
#19948=ORIENTED_EDGE('',*,*,#14092,.F.);
#19949=ORIENTED_EDGE('',*,*,#13738,.F.);
#19950=ORIENTED_EDGE('',*,*,#14736,.T.);
#19951=ORIENTED_EDGE('',*,*,#14216,.F.);
#19952=ORIENTED_EDGE('',*,*,#14507,.F.);
#19953=ORIENTED_EDGE('',*,*,#14737,.F.);
#19954=ORIENTED_EDGE('',*,*,#14093,.F.);
#19955=ORIENTED_EDGE('',*,*,#14737,.T.);
#19956=ORIENTED_EDGE('',*,*,#14509,.F.);
#19957=ORIENTED_EDGE('',*,*,#14097,.F.);
#19958=ORIENTED_EDGE('',*,*,#13740,.F.);
#19959=ORIENTED_EDGE('',*,*,#14091,.F.);
#19960=ORIENTED_EDGE('',*,*,#14096,.T.);
#19961=ORIENTED_EDGE('',*,*,#14508,.F.);
#19962=ORIENTED_EDGE('',*,*,#14214,.F.);
#19963=ORIENTED_EDGE('',*,*,#14522,.F.);
#19964=ORIENTED_EDGE('',*,*,#13961,.T.);
#19965=ORIENTED_EDGE('',*,*,#14738,.T.);
#19966=ORIENTED_EDGE('',*,*,#14739,.T.);
#19967=ORIENTED_EDGE('',*,*,#14738,.F.);
#19968=ORIENTED_EDGE('',*,*,#14740,.F.);
#19969=ORIENTED_EDGE('',*,*,#14741,.F.);
#19970=ORIENTED_EDGE('',*,*,#14742,.T.);
#19971=ORIENTED_EDGE('',*,*,#14740,.T.);
#19972=ORIENTED_EDGE('',*,*,#14742,.F.);
#19973=ORIENTED_EDGE('',*,*,#14743,.F.);
#19974=ORIENTED_EDGE('',*,*,#14744,.T.);
#19975=ORIENTED_EDGE('',*,*,#14741,.T.);
#19976=ORIENTED_EDGE('',*,*,#14744,.F.);
#19977=ORIENTED_EDGE('',*,*,#14520,.T.);
#19978=ORIENTED_EDGE('',*,*,#14517,.T.);
#19979=ORIENTED_EDGE('',*,*,#14510,.T.);
#19980=ORIENTED_EDGE('',*,*,#14514,.T.);
#19981=ORIENTED_EDGE('',*,*,#14739,.F.);
#19982=ORIENTED_EDGE('',*,*,#14743,.T.);
#19983=ORIENTED_EDGE('',*,*,#14745,.F.);
#19984=ORIENTED_EDGE('',*,*,#14746,.T.);
#19985=ORIENTED_EDGE('',*,*,#14440,.T.);
#19986=ORIENTED_EDGE('',*,*,#14746,.F.);
#19987=ORIENTED_EDGE('',*,*,#14745,.T.);
#23589=CONICAL_SURFACE('',#26055,7.69,0.785398163397446);
#23911=ADVANCED_FACE('',(#2052),#814,.T.);
#23912=ADVANCED_FACE('',(#2053,#645),#815,.F.);
#23913=ADVANCED_FACE('',(#2054),#816,.T.);
#23914=ADVANCED_FACE('',(#2055),#817,.T.);
#23915=ADVANCED_FACE('',(#2056),#818,.T.);
#23916=ADVANCED_FACE('',(#2057),#819,.T.);
#23917=ADVANCED_FACE('',(#2058),#820,.T.);
#23918=ADVANCED_FACE('',(#2059),#821,.T.);
#23919=ADVANCED_FACE('',(#2060),#822,.T.);
#23920=ADVANCED_FACE('',(#2061),#823,.T.);
#23921=ADVANCED_FACE('',(#2062),#824,.T.);
#23922=ADVANCED_FACE('',(#2063),#825,.T.);
#23923=ADVANCED_FACE('',(#2064),#826,.T.);
#23924=ADVANCED_FACE('',(#2065),#827,.T.);
#23925=ADVANCED_FACE('',(#2066),#828,.T.);
#23926=ADVANCED_FACE('',(#2067),#829,.T.);
#23927=ADVANCED_FACE('',(#2068),#830,.T.);
#23928=ADVANCED_FACE('',(#2069),#831,.T.);
#23929=ADVANCED_FACE('',(#2070),#832,.T.);
#23930=ADVANCED_FACE('',(#2071),#833,.T.);
#23931=ADVANCED_FACE('',(#2072),#834,.T.);
#23932=ADVANCED_FACE('',(#2073),#835,.T.);
#23933=ADVANCED_FACE('',(#2074),#836,.T.);
#23934=ADVANCED_FACE('',(#2075),#837,.T.);
#23935=ADVANCED_FACE('',(#2076),#838,.T.);
#23936=ADVANCED_FACE('',(#2077),#839,.T.);
#23937=ADVANCED_FACE('',(#2078),#840,.T.);
#23938=ADVANCED_FACE('',(#2079),#841,.T.);
#23939=ADVANCED_FACE('',(#2080),#842,.T.);
#23940=ADVANCED_FACE('',(#2081),#843,.T.);
#23941=ADVANCED_FACE('',(#2082),#844,.T.);
#23942=ADVANCED_FACE('',(#2083),#845,.T.);
#23943=ADVANCED_FACE('',(#2084),#846,.T.);
#23944=ADVANCED_FACE('',(#2085),#847,.T.);
#23945=ADVANCED_FACE('',(#2086),#848,.T.);
#23946=ADVANCED_FACE('',(#2087),#849,.T.);
#23947=ADVANCED_FACE('',(#2088),#850,.T.);
#23948=ADVANCED_FACE('',(#2089),#851,.T.);
#23949=ADVANCED_FACE('',(#2090),#852,.T.);
#23950=ADVANCED_FACE('',(#2091),#853,.T.);
#23951=ADVANCED_FACE('',(#2092),#854,.T.);
#23952=ADVANCED_FACE('',(#2093),#855,.T.);
#23953=ADVANCED_FACE('',(#2094),#856,.T.);
#23954=ADVANCED_FACE('',(#2095),#857,.T.);
#23955=ADVANCED_FACE('',(#2096),#858,.T.);
#23956=ADVANCED_FACE('',(#2097),#859,.T.);
#23957=ADVANCED_FACE('',(#2098),#860,.T.);
#23958=ADVANCED_FACE('',(#2099),#861,.T.);
#23959=ADVANCED_FACE('',(#2100),#862,.T.);
#23960=ADVANCED_FACE('',(#2101),#863,.T.);
#23961=ADVANCED_FACE('',(#2102),#864,.T.);
#23962=ADVANCED_FACE('',(#2103),#865,.T.);
#23963=ADVANCED_FACE('',(#2104),#866,.T.);
#23964=ADVANCED_FACE('',(#2105),#867,.T.);
#23965=ADVANCED_FACE('',(#2106),#868,.T.);
#23966=ADVANCED_FACE('',(#2107),#869,.T.);
#23967=ADVANCED_FACE('',(#2108),#870,.T.);
#23968=ADVANCED_FACE('',(#2109),#871,.T.);
#23969=ADVANCED_FACE('',(#2110),#872,.T.);
#23970=ADVANCED_FACE('',(#2111),#873,.T.);
#23971=ADVANCED_FACE('',(#2112),#874,.T.);
#23972=ADVANCED_FACE('',(#2113),#875,.T.);
#23973=ADVANCED_FACE('',(#2114),#876,.T.);
#23974=ADVANCED_FACE('',(#2115),#877,.T.);
#23975=ADVANCED_FACE('',(#2116),#878,.T.);
#23976=ADVANCED_FACE('',(#2117),#879,.T.);
#23977=ADVANCED_FACE('',(#2118),#880,.T.);
#23978=ADVANCED_FACE('',(#2119),#881,.T.);
#23979=ADVANCED_FACE('',(#2120),#882,.T.);
#23980=ADVANCED_FACE('',(#2121),#883,.T.);
#23981=ADVANCED_FACE('',(#2122),#884,.T.);
#23982=ADVANCED_FACE('',(#2123),#885,.T.);
#23983=ADVANCED_FACE('',(#2124),#886,.T.);
#23984=ADVANCED_FACE('',(#2125),#887,.T.);
#23985=ADVANCED_FACE('',(#2126,#646),#888,.T.);
#23986=ADVANCED_FACE('',(#2127),#889,.T.);
#23987=ADVANCED_FACE('',(#2128),#890,.T.);
#23988=ADVANCED_FACE('',(#2129),#891,.T.);
#23989=ADVANCED_FACE('',(#2130),#892,.T.);
#23990=ADVANCED_FACE('',(#2131),#893,.T.);
#23991=ADVANCED_FACE('',(#2132),#894,.T.);
#23992=ADVANCED_FACE('',(#2133),#895,.T.);
#23993=ADVANCED_FACE('',(#2134),#896,.T.);
#23994=ADVANCED_FACE('',(#2135),#897,.T.);
#23995=ADVANCED_FACE('',(#2136),#898,.T.);
#23996=ADVANCED_FACE('',(#2137),#899,.T.);
#23997=ADVANCED_FACE('',(#2138),#900,.T.);
#23998=ADVANCED_FACE('',(#2139),#901,.T.);
#23999=ADVANCED_FACE('',(#2140),#902,.T.);
#24000=ADVANCED_FACE('',(#2141),#903,.T.);
#24001=ADVANCED_FACE('',(#2142),#904,.T.);
#24002=ADVANCED_FACE('',(#2143),#905,.T.);
#24003=ADVANCED_FACE('',(#2144),#906,.T.);
#24004=ADVANCED_FACE('',(#2145),#907,.T.);
#24005=ADVANCED_FACE('',(#2146),#908,.T.);
#24006=ADVANCED_FACE('',(#2147),#909,.T.);
#24007=ADVANCED_FACE('',(#2148),#910,.T.);
#24008=ADVANCED_FACE('',(#2149),#911,.T.);
#24009=ADVANCED_FACE('',(#2150),#912,.F.);
#24010=ADVANCED_FACE('',(#2151),#913,.F.);
#24011=ADVANCED_FACE('',(#2152),#914,.F.);
#24012=ADVANCED_FACE('',(#2153),#915,.F.);
#24013=ADVANCED_FACE('',(#2154),#916,.F.);
#24014=ADVANCED_FACE('',(#2155),#917,.T.);
#24015=ADVANCED_FACE('',(#2156),#918,.T.);
#24016=ADVANCED_FACE('',(#2157),#919,.T.);
#24017=ADVANCED_FACE('',(#2158),#920,.T.);
#24018=ADVANCED_FACE('',(#2159),#921,.T.);
#24019=ADVANCED_FACE('',(#2160),#922,.T.);
#24020=ADVANCED_FACE('',(#2161),#923,.T.);
#24021=ADVANCED_FACE('',(#2162),#924,.T.);
#24022=ADVANCED_FACE('',(#2163),#925,.T.);
#24023=ADVANCED_FACE('',(#2164),#926,.T.);
#24024=ADVANCED_FACE('',(#2165),#927,.T.);
#24025=ADVANCED_FACE('',(#2166),#928,.T.);
#24026=ADVANCED_FACE('',(#2167),#929,.T.);
#24027=ADVANCED_FACE('',(#2168),#930,.T.);
#24028=ADVANCED_FACE('',(#2169),#931,.T.);
#24029=ADVANCED_FACE('',(#2170),#932,.T.);
#24030=ADVANCED_FACE('',(#2171),#933,.T.);
#24031=ADVANCED_FACE('',(#2172),#934,.T.);
#24032=ADVANCED_FACE('',(#2173),#935,.T.);
#24033=ADVANCED_FACE('',(#2174),#936,.T.);
#24034=ADVANCED_FACE('',(#2175),#937,.T.);
#24035=ADVANCED_FACE('',(#2176),#938,.T.);
#24036=ADVANCED_FACE('',(#2177),#939,.T.);
#24037=ADVANCED_FACE('',(#2178),#940,.T.);
#24038=ADVANCED_FACE('',(#2179),#941,.T.);
#24039=ADVANCED_FACE('',(#2180),#942,.T.);
#24040=ADVANCED_FACE('',(#2181),#943,.T.);
#24041=ADVANCED_FACE('',(#2182),#944,.T.);
#24042=ADVANCED_FACE('',(#2183),#945,.T.);
#24043=ADVANCED_FACE('',(#2184),#946,.T.);
#24044=ADVANCED_FACE('',(#2185),#947,.T.);
#24045=ADVANCED_FACE('',(#2186),#948,.T.);
#24046=ADVANCED_FACE('',(#2187),#949,.T.);
#24047=ADVANCED_FACE('',(#2188),#950,.T.);
#24048=ADVANCED_FACE('',(#2189),#951,.T.);
#24049=ADVANCED_FACE('',(#2190),#952,.T.);
#24050=ADVANCED_FACE('',(#2191),#953,.T.);
#24051=ADVANCED_FACE('',(#2192),#954,.T.);
#24052=ADVANCED_FACE('',(#2193),#955,.T.);
#24053=ADVANCED_FACE('',(#2194),#956,.T.);
#24054=ADVANCED_FACE('',(#2195),#957,.T.);
#24055=ADVANCED_FACE('',(#2196),#958,.T.);
#24056=ADVANCED_FACE('',(#2197),#959,.T.);
#24057=ADVANCED_FACE('',(#2198),#960,.T.);
#24058=ADVANCED_FACE('',(#2199),#961,.T.);
#24059=ADVANCED_FACE('',(#2200),#962,.T.);
#24060=ADVANCED_FACE('',(#2201),#963,.T.);
#24061=ADVANCED_FACE('',(#2202),#964,.T.);
#24062=ADVANCED_FACE('',(#2203),#965,.T.);
#24063=ADVANCED_FACE('',(#2204),#966,.T.);
#24064=ADVANCED_FACE('',(#2205),#967,.T.);
#24065=ADVANCED_FACE('',(#2206),#968,.T.);
#24066=ADVANCED_FACE('',(#2207),#969,.T.);
#24067=ADVANCED_FACE('',(#2208),#970,.T.);
#24068=ADVANCED_FACE('',(#2209),#971,.T.);
#24069=ADVANCED_FACE('',(#2210),#972,.T.);
#24070=ADVANCED_FACE('',(#2211),#973,.T.);
#24071=ADVANCED_FACE('',(#2212),#974,.T.);
#24072=ADVANCED_FACE('',(#2213),#975,.T.);
#24073=ADVANCED_FACE('',(#2214),#976,.T.);
#24074=ADVANCED_FACE('',(#2215),#977,.T.);
#24075=ADVANCED_FACE('',(#2216),#978,.T.);
#24076=ADVANCED_FACE('',(#2217),#979,.T.);
#24077=ADVANCED_FACE('',(#2218),#980,.T.);
#24078=ADVANCED_FACE('',(#2219),#981,.T.);
#24079=ADVANCED_FACE('',(#2220),#982,.T.);
#24080=ADVANCED_FACE('',(#2221),#983,.T.);
#24081=ADVANCED_FACE('',(#2222),#984,.T.);
#24082=ADVANCED_FACE('',(#2223),#985,.T.);
#24083=ADVANCED_FACE('',(#2224),#986,.T.);
#24084=ADVANCED_FACE('',(#2225),#987,.T.);
#24085=ADVANCED_FACE('',(#2226),#988,.T.);
#24086=ADVANCED_FACE('',(#2227),#989,.T.);
#24087=ADVANCED_FACE('',(#2228),#990,.T.);
#24088=ADVANCED_FACE('',(#2229),#991,.T.);
#24089=ADVANCED_FACE('',(#2230),#992,.T.);
#24090=ADVANCED_FACE('',(#2231),#993,.T.);
#24091=ADVANCED_FACE('',(#2232),#994,.T.);
#24092=ADVANCED_FACE('',(#2233),#995,.T.);
#24093=ADVANCED_FACE('',(#2234),#996,.T.);
#24094=ADVANCED_FACE('',(#2235),#997,.T.);
#24095=ADVANCED_FACE('',(#2236),#998,.T.);
#24096=ADVANCED_FACE('',(#2237),#999,.T.);
#24097=ADVANCED_FACE('',(#2238),#1000,.T.);
#24098=ADVANCED_FACE('',(#2239),#1001,.T.);
#24099=ADVANCED_FACE('',(#2240),#1002,.T.);
#24100=ADVANCED_FACE('',(#2241),#1003,.T.);
#24101=ADVANCED_FACE('',(#2242),#1004,.T.);
#24102=ADVANCED_FACE('',(#2243),#1005,.T.);
#24103=ADVANCED_FACE('',(#2244),#1006,.T.);
#24104=ADVANCED_FACE('',(#2245),#1007,.T.);
#24105=ADVANCED_FACE('',(#2246),#1008,.T.);
#24106=ADVANCED_FACE('',(#2247),#1009,.T.);
#24107=ADVANCED_FACE('',(#2248),#1010,.T.);
#24108=ADVANCED_FACE('',(#2249),#1011,.T.);
#24109=ADVANCED_FACE('',(#2250),#1012,.T.);
#24110=ADVANCED_FACE('',(#2251),#1013,.T.);
#24111=ADVANCED_FACE('',(#2252),#1014,.T.);
#24112=ADVANCED_FACE('',(#2253),#1015,.T.);
#24113=ADVANCED_FACE('',(#2254),#1016,.T.);
#24114=ADVANCED_FACE('',(#2255),#1017,.T.);
#24115=ADVANCED_FACE('',(#2256),#1018,.T.);
#24116=ADVANCED_FACE('',(#2257),#1019,.T.);
#24117=ADVANCED_FACE('',(#2258),#1020,.T.);
#24118=ADVANCED_FACE('',(#2259),#1021,.T.);
#24119=ADVANCED_FACE('',(#2260),#1022,.T.);
#24120=ADVANCED_FACE('',(#2261),#1023,.T.);
#24121=ADVANCED_FACE('',(#2262),#1024,.T.);
#24122=ADVANCED_FACE('',(#2263),#1025,.T.);
#24123=ADVANCED_FACE('',(#2264),#1026,.T.);
#24124=ADVANCED_FACE('',(#2265),#1027,.T.);
#24125=ADVANCED_FACE('',(#2266),#1028,.T.);
#24126=ADVANCED_FACE('',(#2267),#1029,.T.);
#24127=ADVANCED_FACE('',(#2268),#1030,.T.);
#24128=ADVANCED_FACE('',(#2269),#1031,.T.);
#24129=ADVANCED_FACE('',(#2270),#1032,.T.);
#24130=ADVANCED_FACE('',(#2271),#1033,.T.);
#24131=ADVANCED_FACE('',(#2272),#1034,.T.);
#24132=ADVANCED_FACE('',(#2273),#1035,.T.);
#24133=ADVANCED_FACE('',(#2274),#1036,.T.);
#24134=ADVANCED_FACE('',(#2275),#1037,.T.);
#24135=ADVANCED_FACE('',(#2276),#1038,.T.);
#24136=ADVANCED_FACE('',(#2277),#1039,.T.);
#24137=ADVANCED_FACE('',(#2278),#1040,.T.);
#24138=ADVANCED_FACE('',(#2279),#1041,.T.);
#24139=ADVANCED_FACE('',(#2280),#1042,.T.);
#24140=ADVANCED_FACE('',(#2281),#1043,.T.);
#24141=ADVANCED_FACE('',(#2282),#1044,.T.);
#24142=ADVANCED_FACE('',(#2283),#1045,.T.);
#24143=ADVANCED_FACE('',(#2284),#1046,.T.);
#24144=ADVANCED_FACE('',(#2285),#1047,.T.);
#24145=ADVANCED_FACE('',(#2286),#1048,.T.);
#24146=ADVANCED_FACE('',(#2287),#1049,.T.);
#24147=ADVANCED_FACE('',(#2288),#1050,.T.);
#24148=ADVANCED_FACE('',(#2289),#1051,.T.);
#24149=ADVANCED_FACE('',(#2290),#1052,.T.);
#24150=ADVANCED_FACE('',(#2291),#1053,.T.);
#24151=ADVANCED_FACE('',(#2292),#1054,.T.);
#24152=ADVANCED_FACE('',(#2293),#1055,.T.);
#24153=ADVANCED_FACE('',(#2294),#1056,.T.);
#24154=ADVANCED_FACE('',(#2295),#1057,.T.);
#24155=ADVANCED_FACE('',(#2296),#1058,.T.);
#24156=ADVANCED_FACE('',(#2297),#1059,.T.);
#24157=ADVANCED_FACE('',(#2298),#1060,.T.);
#24158=ADVANCED_FACE('',(#2299),#1061,.T.);
#24159=ADVANCED_FACE('',(#2300),#1062,.T.);
#24160=ADVANCED_FACE('',(#2301),#1063,.T.);
#24161=ADVANCED_FACE('',(#2302),#1064,.T.);
#24162=ADVANCED_FACE('',(#2303),#1065,.T.);
#24163=ADVANCED_FACE('',(#2304),#1066,.T.);
#24164=ADVANCED_FACE('',(#2305),#1067,.T.);
#24165=ADVANCED_FACE('',(#2306),#1068,.T.);
#24166=ADVANCED_FACE('',(#2307),#1069,.T.);
#24167=ADVANCED_FACE('',(#2308),#1070,.T.);
#24168=ADVANCED_FACE('',(#2309),#1071,.T.);
#24169=ADVANCED_FACE('',(#2310),#1072,.T.);
#24170=ADVANCED_FACE('',(#2311),#1073,.T.);
#24171=ADVANCED_FACE('',(#2312),#1074,.T.);
#24172=ADVANCED_FACE('',(#2313),#1075,.T.);
#24173=ADVANCED_FACE('',(#2314),#1076,.T.);
#24174=ADVANCED_FACE('',(#2315),#1077,.T.);
#24175=ADVANCED_FACE('',(#2316),#1078,.T.);
#24176=ADVANCED_FACE('',(#2317),#1079,.T.);
#24177=ADVANCED_FACE('',(#2318),#1080,.T.);
#24178=ADVANCED_FACE('',(#2319),#1081,.T.);
#24179=ADVANCED_FACE('',(#2320),#1082,.T.);
#24180=ADVANCED_FACE('',(#2321),#1083,.T.);
#24181=ADVANCED_FACE('',(#2322),#1084,.T.);
#24182=ADVANCED_FACE('',(#2323),#1085,.T.);
#24183=ADVANCED_FACE('',(#2324),#1086,.T.);
#24184=ADVANCED_FACE('',(#2325),#1087,.T.);
#24185=ADVANCED_FACE('',(#2326),#1088,.T.);
#24186=ADVANCED_FACE('',(#2327),#1089,.T.);
#24187=ADVANCED_FACE('',(#2328),#1090,.T.);
#24188=ADVANCED_FACE('',(#2329),#1091,.T.);
#24189=ADVANCED_FACE('',(#2330),#1092,.T.);
#24190=ADVANCED_FACE('',(#2331),#1093,.T.);
#24191=ADVANCED_FACE('',(#2332),#1094,.T.);
#24192=ADVANCED_FACE('',(#2333),#1095,.T.);
#24193=ADVANCED_FACE('',(#2334),#1096,.T.);
#24194=ADVANCED_FACE('',(#2335),#1097,.T.);
#24195=ADVANCED_FACE('',(#2336),#1098,.T.);
#24196=ADVANCED_FACE('',(#2337),#1099,.T.);
#24197=ADVANCED_FACE('',(#2338),#1100,.T.);
#24198=ADVANCED_FACE('',(#2339),#1101,.T.);
#24199=ADVANCED_FACE('',(#2340),#1102,.T.);
#24200=ADVANCED_FACE('',(#2341),#1103,.T.);
#24201=ADVANCED_FACE('',(#2342),#1104,.T.);
#24202=ADVANCED_FACE('',(#2343),#1105,.T.);
#24203=ADVANCED_FACE('',(#2344),#1106,.T.);
#24204=ADVANCED_FACE('',(#2345),#1107,.T.);
#24205=ADVANCED_FACE('',(#2346),#1108,.T.);
#24206=ADVANCED_FACE('',(#2347),#1109,.T.);
#24207=ADVANCED_FACE('',(#2348),#1110,.T.);
#24208=ADVANCED_FACE('',(#2349),#1111,.T.);
#24209=ADVANCED_FACE('',(#2350),#1112,.T.);
#24210=ADVANCED_FACE('',(#2351),#1113,.T.);
#24211=ADVANCED_FACE('',(#2352),#1114,.T.);
#24212=ADVANCED_FACE('',(#2353),#1115,.T.);
#24213=ADVANCED_FACE('',(#2354),#1116,.T.);
#24214=ADVANCED_FACE('',(#2355),#1117,.T.);
#24215=ADVANCED_FACE('',(#2356),#1118,.T.);
#24216=ADVANCED_FACE('',(#2357),#1119,.T.);
#24217=ADVANCED_FACE('',(#2358),#1120,.T.);
#24218=ADVANCED_FACE('',(#2359),#1121,.T.);
#24219=ADVANCED_FACE('',(#2360),#1122,.T.);
#24220=ADVANCED_FACE('',(#2361),#1123,.T.);
#24221=ADVANCED_FACE('',(#2362),#1124,.T.);
#24222=ADVANCED_FACE('',(#2363),#1125,.T.);
#24223=ADVANCED_FACE('',(#2364),#1126,.T.);
#24224=ADVANCED_FACE('',(#2365),#1127,.T.);
#24225=ADVANCED_FACE('',(#2366),#1128,.T.);
#24226=ADVANCED_FACE('',(#2367),#1129,.T.);
#24227=ADVANCED_FACE('',(#2368),#1130,.T.);
#24228=ADVANCED_FACE('',(#2369),#1131,.T.);
#24229=ADVANCED_FACE('',(#2370),#1132,.T.);
#24230=ADVANCED_FACE('',(#2371),#1133,.T.);
#24231=ADVANCED_FACE('',(#2372),#1134,.T.);
#24232=ADVANCED_FACE('',(#2373),#1135,.T.);
#24233=ADVANCED_FACE('',(#2374),#1136,.T.);
#24234=ADVANCED_FACE('',(#2375),#1137,.T.);
#24235=ADVANCED_FACE('',(#2376),#1138,.T.);
#24236=ADVANCED_FACE('',(#2377),#1139,.T.);
#24237=ADVANCED_FACE('',(#2378),#1140,.T.);
#24238=ADVANCED_FACE('',(#2379),#1141,.T.);
#24239=ADVANCED_FACE('',(#2380),#1142,.T.);
#24240=ADVANCED_FACE('',(#2381),#1143,.T.);
#24241=ADVANCED_FACE('',(#2382),#1144,.T.);
#24242=ADVANCED_FACE('',(#2383),#1145,.T.);
#24243=ADVANCED_FACE('',(#2384),#1146,.T.);
#24244=ADVANCED_FACE('',(#2385),#1147,.T.);
#24245=ADVANCED_FACE('',(#2386),#1148,.T.);
#24246=ADVANCED_FACE('',(#2387),#1149,.T.);
#24247=ADVANCED_FACE('',(#2388),#1150,.T.);
#24248=ADVANCED_FACE('',(#2389),#1151,.T.);
#24249=ADVANCED_FACE('',(#2390),#1152,.T.);
#24250=ADVANCED_FACE('',(#2391),#1153,.T.);
#24251=ADVANCED_FACE('',(#2392),#1154,.T.);
#24252=ADVANCED_FACE('',(#2393),#1155,.T.);
#24253=ADVANCED_FACE('',(#2394),#1156,.T.);
#24254=ADVANCED_FACE('',(#2395),#514,.T.);
#24255=ADVANCED_FACE('',(#2396),#1157,.T.);
#24256=ADVANCED_FACE('',(#2397),#23589,.T.);
#24257=ADVANCED_FACE('',(#2398,#647),#515,.T.);
#24258=ADVANCED_FACE('',(#2399,#648),#1158,.T.);
#24259=ADVANCED_FACE('',(#2400),#516,.T.);
#24260=ADVANCED_FACE('',(#2401),#1159,.T.);
#24940=CLOSED_SHELL('',(#23911,#23912,#23913,#23914,#23915,#23916,#23917,
#23918,#23919,#23920,#23921,#23922,#23923,#23924,#23925,#23926,#23927,#23928,
#23929,#23930,#23931,#23932,#23933,#23934,#23935,#23936,#23937,#23938,#23939,
#23940,#23941,#23942,#23943,#23944,#23945,#23946,#23947,#23948,#23949,#23950,
#23951,#23952,#23953,#23954,#23955,#23956,#23957,#23958,#23959,#23960,#23961,
#23962,#23963,#23964,#23965,#23966,#23967,#23968,#23969,#23970,#23971,#23972,
#23973,#23974,#23975,#23976,#23977,#23978,#23979,#23980,#23981,#23982,#23983,
#23984,#23985,#23986,#23987,#23988,#23989,#23990,#23991,#23992,#23993,#23994,
#23995,#23996,#23997,#23998,#23999,#24000,#24001,#24002,#24003,#24004,#24005,
#24006,#24007,#24008,#24009,#24010,#24011,#24012,#24013,#24014,#24015,#24016,
#24017,#24018,#24019,#24020,#24021,#24022,#24023,#24024,#24025,#24026,#24027,
#24028,#24029,#24030,#24031,#24032,#24033,#24034,#24035,#24036,#24037,#24038,
#24039,#24040,#24041,#24042,#24043,#24044,#24045,#24046,#24047,#24048,#24049,
#24050,#24051,#24052,#24053,#24054,#24055,#24056,#24057,#24058,#24059,#24060,
#24061,#24062,#24063,#24064,#24065,#24066,#24067,#24068,#24069,#24070,#24071,
#24072,#24073,#24074,#24075,#24076,#24077,#24078,#24079,#24080,#24081,#24082,
#24083,#24084,#24085,#24086,#24087,#24088,#24089,#24090,#24091,#24092,#24093,
#24094,#24095,#24096,#24097,#24098,#24099,#24100,#24101,#24102,#24103,#24104,
#24105,#24106,#24107,#24108,#24109,#24110,#24111,#24112,#24113,#24114,#24115,
#24116,#24117,#24118,#24119,#24120,#24121,#24122,#24123,#24124,#24125,#24126,
#24127,#24128,#24129,#24130,#24131,#24132,#24133,#24134,#24135,#24136,#24137,
#24138,#24139,#24140,#24141,#24142,#24143,#24144,#24145,#24146,#24147,#24148,
#24149,#24150,#24151,#24152,#24153,#24154,#24155,#24156,#24157,#24158,#24159,
#24160,#24161,#24162,#24163,#24164,#24165,#24166,#24167,#24168,#24169,#24170,
#24171,#24172,#24173,#24174,#24175,#24176,#24177,#24178,#24179,#24180,#24181,
#24182,#24183,#24184,#24185,#24186,#24187,#24188,#24189,#24190,#24191,#24192,
#24193,#24194,#24195,#24196,#24197,#24198,#24199,#24200,#24201,#24202,#24203,
#24204,#24205,#24206,#24207,#24208,#24209,#24210,#24211,#24212,#24213,#24214,
#24215,#24216,#24217,#24218,#24219,#24220,#24221,#24222,#24223,#24224,#24225,
#24226,#24227,#24228,#24229,#24230,#24231,#24232,#24233,#24234,#24235,#24236,
#24237,#24238,#24239,#24240,#24241,#24242,#24243,#24244,#24245,#24246,#24247,
#24248,#24249,#24250,#24251,#24252,#24253,#24254,#24255,#24256,#24257,#24258,
#24259,#24260));
#25703=AXIS2_PLACEMENT_3D('',#36027,#28460,#28461);
#25704=AXIS2_PLACEMENT_3D('',#36028,#28462,#28463);
#25705=AXIS2_PLACEMENT_3D('',#36041,#28470,#28471);
#25706=AXIS2_PLACEMENT_3D('',#36520,#28711,#28712);
#25707=AXIS2_PLACEMENT_3D('',#36521,#28713,#28714);
#25708=AXIS2_PLACEMENT_3D('',#36529,#28719,#28720);
#25709=AXIS2_PLACEMENT_3D('',#36533,#28723,#28724);
#25710=AXIS2_PLACEMENT_3D('',#36543,#28730,#28731);
#25711=AXIS2_PLACEMENT_3D('',#36551,#28736,#28737);
#25712=AXIS2_PLACEMENT_3D('',#36555,#28740,#28741);
#25713=AXIS2_PLACEMENT_3D('',#36565,#28747,#28748);
#25714=AXIS2_PLACEMENT_3D('',#36573,#28753,#28754);
#25715=AXIS2_PLACEMENT_3D('',#36577,#28757,#28758);
#25716=AXIS2_PLACEMENT_3D('',#36587,#28764,#28765);
#25717=AXIS2_PLACEMENT_3D('',#36595,#28770,#28771);
#25718=AXIS2_PLACEMENT_3D('',#36599,#28774,#28775);
#25719=AXIS2_PLACEMENT_3D('',#36609,#28781,#28782);
#25720=AXIS2_PLACEMENT_3D('',#36617,#28787,#28788);
#25721=AXIS2_PLACEMENT_3D('',#36621,#28791,#28792);
#25722=AXIS2_PLACEMENT_3D('',#36631,#28798,#28799);
#25723=AXIS2_PLACEMENT_3D('',#36639,#28804,#28805);
#25724=AXIS2_PLACEMENT_3D('',#36643,#28808,#28809);
#25725=AXIS2_PLACEMENT_3D('',#36653,#28815,#28816);
#25726=AXIS2_PLACEMENT_3D('',#36661,#28821,#28822);
#25727=AXIS2_PLACEMENT_3D('',#36665,#28825,#28826);
#25728=AXIS2_PLACEMENT_3D('',#36675,#28832,#28833);
#25729=AXIS2_PLACEMENT_3D('',#36683,#28838,#28839);
#25730=AXIS2_PLACEMENT_3D('',#36687,#28842,#28843);
#25731=AXIS2_PLACEMENT_3D('',#36697,#28849,#28850);
#25732=AXIS2_PLACEMENT_3D('',#36705,#28855,#28856);
#25733=AXIS2_PLACEMENT_3D('',#36709,#28859,#28860);
#25734=AXIS2_PLACEMENT_3D('',#36719,#28866,#28867);
#25735=AXIS2_PLACEMENT_3D('',#36727,#28872,#28873);
#25736=AXIS2_PLACEMENT_3D('',#36731,#28876,#28877);
#25737=AXIS2_PLACEMENT_3D('',#36741,#28883,#28884);
#25738=AXIS2_PLACEMENT_3D('',#36749,#28889,#28890);
#25739=AXIS2_PLACEMENT_3D('',#36753,#28893,#28894);
#25740=AXIS2_PLACEMENT_3D('',#36763,#28900,#28901);
#25741=AXIS2_PLACEMENT_3D('',#36771,#28906,#28907);
#25742=AXIS2_PLACEMENT_3D('',#36775,#28910,#28911);
#25743=AXIS2_PLACEMENT_3D('',#36785,#28917,#28918);
#25744=AXIS2_PLACEMENT_3D('',#36791,#28922,#28923);
#25745=AXIS2_PLACEMENT_3D('',#36795,#28926,#28927);
#25746=AXIS2_PLACEMENT_3D('',#36805,#28933,#28934);
#25747=AXIS2_PLACEMENT_3D('',#36811,#28938,#28939);
#25748=AXIS2_PLACEMENT_3D('',#36815,#28942,#28943);
#25749=AXIS2_PLACEMENT_3D('',#36825,#28949,#28950);
#25750=AXIS2_PLACEMENT_3D('',#36831,#28954,#28955);
#25751=AXIS2_PLACEMENT_3D('',#36835,#28958,#28959);
#25752=AXIS2_PLACEMENT_3D('',#36845,#28965,#28966);
#25753=AXIS2_PLACEMENT_3D('',#36851,#28970,#28971);
#25754=AXIS2_PLACEMENT_3D('',#36855,#28974,#28975);
#25755=AXIS2_PLACEMENT_3D('',#36865,#28981,#28982);
#25756=AXIS2_PLACEMENT_3D('',#36871,#28986,#28987);
#25757=AXIS2_PLACEMENT_3D('',#36875,#28990,#28991);
#25758=AXIS2_PLACEMENT_3D('',#36885,#28997,#28998);
#25759=AXIS2_PLACEMENT_3D('',#36891,#29002,#29003);
#25760=AXIS2_PLACEMENT_3D('',#36895,#29006,#29007);
#25761=AXIS2_PLACEMENT_3D('',#36905,#29013,#29014);
#25762=AXIS2_PLACEMENT_3D('',#36911,#29018,#29019);
#25763=AXIS2_PLACEMENT_3D('',#36915,#29022,#29023);
#25764=AXIS2_PLACEMENT_3D('',#36925,#29029,#29030);
#25765=AXIS2_PLACEMENT_3D('',#36931,#29034,#29035);
#25766=AXIS2_PLACEMENT_3D('',#36935,#29038,#29039);
#25767=AXIS2_PLACEMENT_3D('',#36945,#29045,#29046);
#25768=AXIS2_PLACEMENT_3D('',#36951,#29050,#29051);
#25769=AXIS2_PLACEMENT_3D('',#36955,#29054,#29055);
#25770=AXIS2_PLACEMENT_3D('',#36965,#29061,#29062);
#25771=AXIS2_PLACEMENT_3D('',#36971,#29066,#29067);
#25772=AXIS2_PLACEMENT_3D('',#36975,#29070,#29071);
#25773=AXIS2_PLACEMENT_3D('',#36985,#29077,#29078);
#25774=AXIS2_PLACEMENT_3D('',#36991,#29082,#29083);
#25775=AXIS2_PLACEMENT_3D('',#36995,#29086,#29087);
#25776=AXIS2_PLACEMENT_3D('',#37005,#29093,#29094);
#25777=AXIS2_PLACEMENT_3D('',#37011,#29098,#29099);
#25778=AXIS2_PLACEMENT_3D('',#37015,#29102,#29103);
#25779=AXIS2_PLACEMENT_3D('',#37023,#29108,#29109);
#25780=AXIS2_PLACEMENT_3D('',#37467,#29337,#29338);
#25781=AXIS2_PLACEMENT_3D('',#37468,#29339,#29340);
#25782=AXIS2_PLACEMENT_3D('',#37473,#29344,#29345);
#25783=AXIS2_PLACEMENT_3D('',#37479,#29349,#29350);
#25784=AXIS2_PLACEMENT_3D('',#37484,#29354,#29355);
#25785=AXIS2_PLACEMENT_3D('',#37490,#29359,#29360);
#25786=AXIS2_PLACEMENT_3D('',#37495,#29364,#29365);
#25787=AXIS2_PLACEMENT_3D('',#37501,#29369,#29370);
#25788=AXIS2_PLACEMENT_3D('',#37506,#29374,#29375);
#25789=AXIS2_PLACEMENT_3D('',#37512,#29379,#29380);
#25790=AXIS2_PLACEMENT_3D('',#37517,#29384,#29385);
#25791=AXIS2_PLACEMENT_3D('',#37523,#29389,#29390);
#25792=AXIS2_PLACEMENT_3D('',#37528,#29394,#29395);
#25793=AXIS2_PLACEMENT_3D('',#37534,#29399,#29400);
#25794=AXIS2_PLACEMENT_3D('',#37539,#29404,#29405);
#25795=AXIS2_PLACEMENT_3D('',#37545,#29409,#29410);
#25796=AXIS2_PLACEMENT_3D('',#37550,#29414,#29415);
#25797=AXIS2_PLACEMENT_3D('',#37556,#29419,#29420);
#25798=AXIS2_PLACEMENT_3D('',#37561,#29424,#29425);
#25799=AXIS2_PLACEMENT_3D('',#37567,#29429,#29430);
#25800=AXIS2_PLACEMENT_3D('',#37572,#29434,#29435);
#25801=AXIS2_PLACEMENT_3D('',#37578,#29439,#29440);
#25802=AXIS2_PLACEMENT_3D('',#37583,#29444,#29445);
#25803=AXIS2_PLACEMENT_3D('',#37589,#29449,#29450);
#25804=AXIS2_PLACEMENT_3D('',#37594,#29454,#29455);
#25805=AXIS2_PLACEMENT_3D('',#37597,#29456,#29457);
#25806=AXIS2_PLACEMENT_3D('',#37603,#29461,#29462);
#25807=AXIS2_PLACEMENT_3D('',#37609,#29466,#29467);
#25808=AXIS2_PLACEMENT_3D('',#37615,#29471,#29472);
#25809=AXIS2_PLACEMENT_3D('',#37616,#29473,#29474);
#25810=AXIS2_PLACEMENT_3D('',#37618,#29476,#29477);
#25811=AXIS2_PLACEMENT_3D('',#37619,#29478,#29479);
#25812=AXIS2_PLACEMENT_3D('',#37622,#29482,#29483);
#25813=AXIS2_PLACEMENT_3D('',#37624,#29485,#29486);
#25814=AXIS2_PLACEMENT_3D('',#37625,#29487,#29488);
#25815=AXIS2_PLACEMENT_3D('',#37627,#29490,#29491);
#25816=AXIS2_PLACEMENT_3D('',#37629,#29493,#29494);
#25817=AXIS2_PLACEMENT_3D('',#37631,#29496,#29497);
#25818=AXIS2_PLACEMENT_3D('',#37633,#29499,#29500);
#25819=AXIS2_PLACEMENT_3D('',#37635,#29502,#29503);
#25820=AXIS2_PLACEMENT_3D('',#37637,#29505,#29506);
#25821=AXIS2_PLACEMENT_3D('',#37639,#29508,#29509);
#25822=AXIS2_PLACEMENT_3D('',#37641,#29511,#29512);
#25823=AXIS2_PLACEMENT_3D('',#37643,#29514,#29515);
#25824=AXIS2_PLACEMENT_3D('',#37645,#29517,#29518);
#25825=AXIS2_PLACEMENT_3D('',#37647,#29520,#29521);
#25826=AXIS2_PLACEMENT_3D('',#37649,#29523,#29524);
#25827=AXIS2_PLACEMENT_3D('',#37651,#29526,#29527);
#25828=AXIS2_PLACEMENT_3D('',#37653,#29529,#29530);
#25829=AXIS2_PLACEMENT_3D('',#37655,#29532,#29533);
#25830=AXIS2_PLACEMENT_3D('',#37656,#29534,#29535);
#25831=AXIS2_PLACEMENT_3D('',#37658,#29537,#29538);
#25832=AXIS2_PLACEMENT_3D('',#37660,#29540,#29541);
#25833=AXIS2_PLACEMENT_3D('',#37662,#29543,#29544);
#25834=AXIS2_PLACEMENT_3D('',#37663,#29545,#29546);
#25835=AXIS2_PLACEMENT_3D('',#37665,#29548,#29549);
#25836=AXIS2_PLACEMENT_3D('',#37667,#29551,#29552);
#25837=AXIS2_PLACEMENT_3D('',#37669,#29554,#29555);
#25838=AXIS2_PLACEMENT_3D('',#37671,#29557,#29558);
#25839=AXIS2_PLACEMENT_3D('',#37673,#29560,#29561);
#25840=AXIS2_PLACEMENT_3D('',#37675,#29563,#29564);
#25841=AXIS2_PLACEMENT_3D('',#37677,#29566,#29567);
#25842=AXIS2_PLACEMENT_3D('',#37679,#29569,#29570);
#25843=AXIS2_PLACEMENT_3D('',#37681,#29572,#29573);
#25844=AXIS2_PLACEMENT_3D('',#37683,#29575,#29576);
#25845=AXIS2_PLACEMENT_3D('',#37685,#29578,#29579);
#25846=AXIS2_PLACEMENT_3D('',#37687,#29581,#29582);
#25847=AXIS2_PLACEMENT_3D('',#37689,#29584,#29585);
#25848=AXIS2_PLACEMENT_3D('',#37691,#29587,#29588);
#25849=AXIS2_PLACEMENT_3D('',#37693,#29590,#29591);
#25850=AXIS2_PLACEMENT_3D('',#37694,#29592,#29593);
#25851=AXIS2_PLACEMENT_3D('',#37696,#29595,#29596);
#25852=AXIS2_PLACEMENT_3D('',#37698,#29598,#29599);
#25853=AXIS2_PLACEMENT_3D('',#37700,#29601,#29602);
#25854=AXIS2_PLACEMENT_3D('',#37701,#29603,#29604);
#25855=AXIS2_PLACEMENT_3D('',#37703,#29606,#29607);
#25856=AXIS2_PLACEMENT_3D('',#37705,#29609,#29610);
#25857=AXIS2_PLACEMENT_3D('',#37707,#29612,#29613);
#25858=AXIS2_PLACEMENT_3D('',#37709,#29615,#29616);
#25859=AXIS2_PLACEMENT_3D('',#37711,#29618,#29619);
#25860=AXIS2_PLACEMENT_3D('',#37713,#29621,#29622);
#25861=AXIS2_PLACEMENT_3D('',#37715,#29624,#29625);
#25862=AXIS2_PLACEMENT_3D('',#37717,#29627,#29628);
#25863=AXIS2_PLACEMENT_3D('',#37719,#29630,#29631);
#25864=AXIS2_PLACEMENT_3D('',#37721,#29633,#29634);
#25865=AXIS2_PLACEMENT_3D('',#37723,#29636,#29637);
#25866=AXIS2_PLACEMENT_3D('',#37725,#29639,#29640);
#25867=AXIS2_PLACEMENT_3D('',#37727,#29642,#29643);
#25868=AXIS2_PLACEMENT_3D('',#37729,#29645,#29646);
#25869=AXIS2_PLACEMENT_3D('',#37731,#29648,#29649);
#25870=AXIS2_PLACEMENT_3D('',#37732,#29650,#29651);
#25871=AXIS2_PLACEMENT_3D('',#37734,#29653,#29654);
#25872=AXIS2_PLACEMENT_3D('',#37736,#29656,#29657);
#25873=AXIS2_PLACEMENT_3D('',#37738,#29659,#29660);
#25874=AXIS2_PLACEMENT_3D('',#37739,#29661,#29662);
#25875=AXIS2_PLACEMENT_3D('',#37741,#29664,#29665);
#25876=AXIS2_PLACEMENT_3D('',#37743,#29667,#29668);
#25877=AXIS2_PLACEMENT_3D('',#37745,#29670,#29671);
#25878=AXIS2_PLACEMENT_3D('',#37747,#29673,#29674);
#25879=AXIS2_PLACEMENT_3D('',#37749,#29676,#29677);
#25880=AXIS2_PLACEMENT_3D('',#37751,#29679,#29680);
#25881=AXIS2_PLACEMENT_3D('',#37753,#29682,#29683);
#25882=AXIS2_PLACEMENT_3D('',#37755,#29685,#29686);
#25883=AXIS2_PLACEMENT_3D('',#37757,#29688,#29689);
#25884=AXIS2_PLACEMENT_3D('',#37759,#29691,#29692);
#25885=AXIS2_PLACEMENT_3D('',#37761,#29694,#29695);
#25886=AXIS2_PLACEMENT_3D('',#37763,#29697,#29698);
#25887=AXIS2_PLACEMENT_3D('',#37765,#29700,#29701);
#25888=AXIS2_PLACEMENT_3D('',#37767,#29703,#29704);
#25889=AXIS2_PLACEMENT_3D('',#37769,#29706,#29707);
#25890=AXIS2_PLACEMENT_3D('',#37770,#29708,#29709);
#25891=AXIS2_PLACEMENT_3D('',#37772,#29711,#29712);
#25892=AXIS2_PLACEMENT_3D('',#37774,#29714,#29715);
#25893=AXIS2_PLACEMENT_3D('',#37776,#29717,#29718);
#25894=AXIS2_PLACEMENT_3D('',#37777,#29719,#29720);
#25895=AXIS2_PLACEMENT_3D('',#37779,#29722,#29723);
#25896=AXIS2_PLACEMENT_3D('',#37781,#29725,#29726);
#25897=AXIS2_PLACEMENT_3D('',#37783,#29728,#29729);
#25898=AXIS2_PLACEMENT_3D('',#37785,#29731,#29732);
#25899=AXIS2_PLACEMENT_3D('',#37787,#29734,#29735);
#25900=AXIS2_PLACEMENT_3D('',#37789,#29737,#29738);
#25901=AXIS2_PLACEMENT_3D('',#37791,#29740,#29741);
#25902=AXIS2_PLACEMENT_3D('',#37793,#29743,#29744);
#25903=AXIS2_PLACEMENT_3D('',#37795,#29746,#29747);
#25904=AXIS2_PLACEMENT_3D('',#37797,#29749,#29750);
#25905=AXIS2_PLACEMENT_3D('',#37799,#29752,#29753);
#25906=AXIS2_PLACEMENT_3D('',#37801,#29755,#29756);
#25907=AXIS2_PLACEMENT_3D('',#37803,#29758,#29759);
#25908=AXIS2_PLACEMENT_3D('',#37805,#29761,#29762);
#25909=AXIS2_PLACEMENT_3D('',#37807,#29764,#29765);
#25910=AXIS2_PLACEMENT_3D('',#37808,#29766,#29767);
#25911=AXIS2_PLACEMENT_3D('',#37810,#29769,#29770);
#25912=AXIS2_PLACEMENT_3D('',#37812,#29772,#29773);
#25913=AXIS2_PLACEMENT_3D('',#37814,#29775,#29776);
#25914=AXIS2_PLACEMENT_3D('',#37815,#29777,#29778);
#25915=AXIS2_PLACEMENT_3D('',#37817,#29780,#29781);
#25916=AXIS2_PLACEMENT_3D('',#37819,#29783,#29784);
#25917=AXIS2_PLACEMENT_3D('',#37821,#29786,#29787);
#25918=AXIS2_PLACEMENT_3D('',#37823,#29789,#29790);
#25919=AXIS2_PLACEMENT_3D('',#37825,#29792,#29793);
#25920=AXIS2_PLACEMENT_3D('',#37827,#29795,#29796);
#25921=AXIS2_PLACEMENT_3D('',#37829,#29798,#29799);
#25922=AXIS2_PLACEMENT_3D('',#37831,#29801,#29802);
#25923=AXIS2_PLACEMENT_3D('',#37833,#29804,#29805);
#25924=AXIS2_PLACEMENT_3D('',#37835,#29807,#29808);
#25925=AXIS2_PLACEMENT_3D('',#37837,#29810,#29811);
#25926=AXIS2_PLACEMENT_3D('',#37839,#29813,#29814);
#25927=AXIS2_PLACEMENT_3D('',#37841,#29816,#29817);
#25928=AXIS2_PLACEMENT_3D('',#37843,#29819,#29820);
#25929=AXIS2_PLACEMENT_3D('',#37845,#29822,#29823);
#25930=AXIS2_PLACEMENT_3D('',#37846,#29824,#29825);
#25931=AXIS2_PLACEMENT_3D('',#37848,#29827,#29828);
#25932=AXIS2_PLACEMENT_3D('',#37850,#29830,#29831);
#25933=AXIS2_PLACEMENT_3D('',#37852,#29833,#29834);
#25934=AXIS2_PLACEMENT_3D('',#37853,#29835,#29836);
#25935=AXIS2_PLACEMENT_3D('',#37855,#29838,#29839);
#25936=AXIS2_PLACEMENT_3D('',#37857,#29841,#29842);
#25937=AXIS2_PLACEMENT_3D('',#37859,#29844,#29845);
#25938=AXIS2_PLACEMENT_3D('',#37861,#29847,#29848);
#25939=AXIS2_PLACEMENT_3D('',#37863,#29850,#29851);
#25940=AXIS2_PLACEMENT_3D('',#37865,#29853,#29854);
#25941=AXIS2_PLACEMENT_3D('',#37867,#29856,#29857);
#25942=AXIS2_PLACEMENT_3D('',#37869,#29859,#29860);
#25943=AXIS2_PLACEMENT_3D('',#37871,#29862,#29863);
#25944=AXIS2_PLACEMENT_3D('',#37873,#29865,#29866);
#25945=AXIS2_PLACEMENT_3D('',#37875,#29868,#29869);
#25946=AXIS2_PLACEMENT_3D('',#37877,#29871,#29872);
#25947=AXIS2_PLACEMENT_3D('',#37879,#29874,#29875);
#25948=AXIS2_PLACEMENT_3D('',#37881,#29877,#29878);
#25949=AXIS2_PLACEMENT_3D('',#37883,#29880,#29881);
#25950=AXIS2_PLACEMENT_3D('',#37884,#29882,#29883);
#25951=AXIS2_PLACEMENT_3D('',#37886,#29885,#29886);
#25952=AXIS2_PLACEMENT_3D('',#37888,#29888,#29889);
#25953=AXIS2_PLACEMENT_3D('',#37890,#29891,#29892);
#25954=AXIS2_PLACEMENT_3D('',#37891,#29893,#29894);
#25955=AXIS2_PLACEMENT_3D('',#37893,#29896,#29897);
#25956=AXIS2_PLACEMENT_3D('',#37895,#29899,#29900);
#25957=AXIS2_PLACEMENT_3D('',#37897,#29902,#29903);
#25958=AXIS2_PLACEMENT_3D('',#37899,#29905,#29906);
#25959=AXIS2_PLACEMENT_3D('',#37901,#29908,#29909);
#25960=AXIS2_PLACEMENT_3D('',#37903,#29911,#29912);
#25961=AXIS2_PLACEMENT_3D('',#37905,#29914,#29915);
#25962=AXIS2_PLACEMENT_3D('',#37907,#29917,#29918);
#25963=AXIS2_PLACEMENT_3D('',#37909,#29920,#29921);
#25964=AXIS2_PLACEMENT_3D('',#37911,#29923,#29924);
#25965=AXIS2_PLACEMENT_3D('',#37913,#29926,#29927);
#25966=AXIS2_PLACEMENT_3D('',#37915,#29929,#29930);
#25967=AXIS2_PLACEMENT_3D('',#37917,#29932,#29933);
#25968=AXIS2_PLACEMENT_3D('',#37919,#29935,#29936);
#25969=AXIS2_PLACEMENT_3D('',#37921,#29938,#29939);
#25970=AXIS2_PLACEMENT_3D('',#37922,#29940,#29941);
#25971=AXIS2_PLACEMENT_3D('',#37924,#29943,#29944);
#25972=AXIS2_PLACEMENT_3D('',#37926,#29946,#29947);
#25973=AXIS2_PLACEMENT_3D('',#37928,#29949,#29950);
#25974=AXIS2_PLACEMENT_3D('',#37929,#29951,#29952);
#25975=AXIS2_PLACEMENT_3D('',#37931,#29954,#29955);
#25976=AXIS2_PLACEMENT_3D('',#37933,#29957,#29958);
#25977=AXIS2_PLACEMENT_3D('',#37935,#29960,#29961);
#25978=AXIS2_PLACEMENT_3D('',#37937,#29963,#29964);
#25979=AXIS2_PLACEMENT_3D('',#37939,#29966,#29967);
#25980=AXIS2_PLACEMENT_3D('',#37941,#29969,#29970);
#25981=AXIS2_PLACEMENT_3D('',#37943,#29972,#29973);
#25982=AXIS2_PLACEMENT_3D('',#37945,#29975,#29976);
#25983=AXIS2_PLACEMENT_3D('',#37947,#29978,#29979);
#25984=AXIS2_PLACEMENT_3D('',#37949,#29981,#29982);
#25985=AXIS2_PLACEMENT_3D('',#37951,#29984,#29985);
#25986=AXIS2_PLACEMENT_3D('',#37953,#29987,#29988);
#25987=AXIS2_PLACEMENT_3D('',#37955,#29990,#29991);
#25988=AXIS2_PLACEMENT_3D('',#37957,#29993,#29994);
#25989=AXIS2_PLACEMENT_3D('',#37959,#29996,#29997);
#25990=AXIS2_PLACEMENT_3D('',#37960,#29998,#29999);
#25991=AXIS2_PLACEMENT_3D('',#37962,#30001,#30002);
#25992=AXIS2_PLACEMENT_3D('',#37964,#30004,#30005);
#25993=AXIS2_PLACEMENT_3D('',#37966,#30007,#30008);
#25994=AXIS2_PLACEMENT_3D('',#37967,#30009,#30010);
#25995=AXIS2_PLACEMENT_3D('',#37969,#30012,#30013);
#25996=AXIS2_PLACEMENT_3D('',#37971,#30015,#30016);
#25997=AXIS2_PLACEMENT_3D('',#37973,#30018,#30019);
#25998=AXIS2_PLACEMENT_3D('',#37975,#30021,#30022);
#25999=AXIS2_PLACEMENT_3D('',#37977,#30024,#30025);
#26000=AXIS2_PLACEMENT_3D('',#37979,#30027,#30028);
#26001=AXIS2_PLACEMENT_3D('',#37981,#30030,#30031);
#26002=AXIS2_PLACEMENT_3D('',#37983,#30033,#30034);
#26003=AXIS2_PLACEMENT_3D('',#37985,#30036,#30037);
#26004=AXIS2_PLACEMENT_3D('',#37987,#30039,#30040);
#26005=AXIS2_PLACEMENT_3D('',#37989,#30042,#30043);
#26006=AXIS2_PLACEMENT_3D('',#37991,#30045,#30046);
#26007=AXIS2_PLACEMENT_3D('',#37993,#30048,#30049);
#26008=AXIS2_PLACEMENT_3D('',#37995,#30051,#30052);
#26009=AXIS2_PLACEMENT_3D('',#37997,#30054,#30055);
#26010=AXIS2_PLACEMENT_3D('',#37998,#30056,#30057);
#26011=AXIS2_PLACEMENT_3D('',#38000,#30059,#30060);
#26012=AXIS2_PLACEMENT_3D('',#38002,#30062,#30063);
#26013=AXIS2_PLACEMENT_3D('',#38004,#30065,#30066);
#26014=AXIS2_PLACEMENT_3D('',#38005,#30067,#30068);
#26015=AXIS2_PLACEMENT_3D('',#38007,#30070,#30071);
#26016=AXIS2_PLACEMENT_3D('',#38009,#30073,#30074);
#26017=AXIS2_PLACEMENT_3D('',#38011,#30076,#30077);
#26018=AXIS2_PLACEMENT_3D('',#38013,#30079,#30080);
#26019=AXIS2_PLACEMENT_3D('',#38015,#30082,#30083);
#26020=AXIS2_PLACEMENT_3D('',#38017,#30085,#30086);
#26021=AXIS2_PLACEMENT_3D('',#38019,#30088,#30089);
#26022=AXIS2_PLACEMENT_3D('',#38021,#30091,#30092);
#26023=AXIS2_PLACEMENT_3D('',#38023,#30094,#30095);
#26024=AXIS2_PLACEMENT_3D('',#38025,#30097,#30098);
#26025=AXIS2_PLACEMENT_3D('',#38027,#30100,#30101);
#26026=AXIS2_PLACEMENT_3D('',#38029,#30103,#30104);
#26027=AXIS2_PLACEMENT_3D('',#38031,#30106,#30107);
#26028=AXIS2_PLACEMENT_3D('',#38033,#30109,#30110);
#26029=AXIS2_PLACEMENT_3D('',#38035,#30112,#30113);
#26030=AXIS2_PLACEMENT_3D('',#38036,#30114,#30115);
#26031=AXIS2_PLACEMENT_3D('',#38038,#30117,#30118);
#26032=AXIS2_PLACEMENT_3D('',#38040,#30120,#30121);
#26033=AXIS2_PLACEMENT_3D('',#38042,#30123,#30124);
#26034=AXIS2_PLACEMENT_3D('',#38043,#30125,#30126);
#26035=AXIS2_PLACEMENT_3D('',#38045,#30128,#30129);
#26036=AXIS2_PLACEMENT_3D('',#38047,#30131,#30132);
#26037=AXIS2_PLACEMENT_3D('',#38049,#30134,#30135);
#26038=AXIS2_PLACEMENT_3D('',#38051,#30137,#30138);
#26039=AXIS2_PLACEMENT_3D('',#38053,#30140,#30141);
#26040=AXIS2_PLACEMENT_3D('',#38055,#30143,#30144);
#26041=AXIS2_PLACEMENT_3D('',#38057,#30146,#30147);
#26042=AXIS2_PLACEMENT_3D('',#38059,#30149,#30150);
#26043=AXIS2_PLACEMENT_3D('',#38061,#30152,#30153);
#26044=AXIS2_PLACEMENT_3D('',#38063,#30155,#30156);
#26045=AXIS2_PLACEMENT_3D('',#38065,#30158,#30159);
#26046=AXIS2_PLACEMENT_3D('',#38067,#30161,#30162);
#26047=AXIS2_PLACEMENT_3D('',#38069,#30164,#30165);
#26048=AXIS2_PLACEMENT_3D('',#38071,#30167,#30168);
#26049=AXIS2_PLACEMENT_3D('',#38073,#30170,#30171);
#26050=AXIS2_PLACEMENT_3D('',#38074,#30172,#30173);
#26051=AXIS2_PLACEMENT_3D('',#38075,#30174,#30175);
#26052=AXIS2_PLACEMENT_3D('',#38078,#30177,#30178);
#26053=AXIS2_PLACEMENT_3D('',#38079,#30179,#30180);
#26054=AXIS2_PLACEMENT_3D('',#38081,#30181,#30182);
#26055=AXIS2_PLACEMENT_3D('',#38082,#30183,#30184);
#26056=AXIS2_PLACEMENT_3D('',#38084,#30185,#30186);
#26057=AXIS2_PLACEMENT_3D('',#38086,#30188,#30189);
#26058=AXIS2_PLACEMENT_3D('',#38088,#30190,#30191);
#26059=AXIS2_PLACEMENT_3D('',#38090,#30193,#30194);
#26060=AXIS2_PLACEMENT_3D('',#38091,#30195,#30196);
#26061=AXIS2_PLACEMENT_3D('',#38093,#30197,#30198);
#26062=AXIS2_PLACEMENT_3D('',#38095,#30200,#30201);
#28460=DIRECTION('axis',(0.,0.,1.));
#28461=DIRECTION('refdir',(1.,0.,0.));
#28462=DIRECTION('center_axis',(-0.548644247294728,-0.70710678118655,0.446082380183749));
#28463=DIRECTION('ref_axis',(0.630855751991531,0.,0.775900135442185));
#28464=DIRECTION('',(-0.228100862670962,-0.386714295024757,-0.893544654996195));
#28465=DIRECTION('',(0.630855751991531,0.,0.775900135442185));
#28466=DIRECTION('',(0.525361147399585,-0.706639907076674,-0.473978592902317));
#28467=DIRECTION('',(-0.630855751991531,0.,-0.775900135442185));
#28468=DIRECTION('',(-0.473949429076065,-0.176491388068498,-0.862683446355688));
#28469=DIRECTION('',(-0.327151215534528,-0.309436927624306,-0.892872258498779));
#28470=DIRECTION('center_axis',(0.,1.,0.));
#28471=DIRECTION('ref_axis',(1.,0.,0.));
#28472=DIRECTION('',(0.742482951693498,0.,-0.669864961350055));
#28473=DIRECTION('',(-0.247344359222329,0.,-0.968927638144818));
#28474=DIRECTION('',(-0.165201002238474,0.,-0.986259919523958));
#28475=DIRECTION('',(-0.0915937869476479,0.,-0.995796454197638));
#28476=DIRECTION('',(-0.0238849697840824,0.,-0.999714713414989));
#28477=DIRECTION('',(0.0393519680027076,0.,-0.99922541131334));
#28478=DIRECTION('',(0.0989820318029304,0.,-0.995089220813975));
#28479=DIRECTION('',(0.854702313102447,0.,-0.51911844118402));
#28480=DIRECTION('',(0.862298277386214,0.,-0.506400711706418));
#28481=DIRECTION('',(0.869705019525388,0.,-0.493571858002809));
#28482=DIRECTION('',(0.876920914189556,0.,-0.480634695228043));
#28483=DIRECTION('',(0.911263560158432,0.,0.411823656347446));
#28484=DIRECTION('',(0.885030574305658,0.,0.465532901677419));
#28485=DIRECTION('',(0.85383585346242,0.,0.520542347309132));
#28486=DIRECTION('',(0.816588132859797,0.,0.577220773424303));
#28487=DIRECTION('',(0.771525643922909,0.,0.636198224431145));
#28488=DIRECTION('',(0.715443769451104,0.,0.69867031764173));
#28489=DIRECTION('',(-0.356521352096954,0.,-0.934287175069293));
#28490=DIRECTION('',(0.951361549480978,0.,-0.308076617368395));
#28491=DIRECTION('',(0.977941578718451,0.,-0.20887859778748));
#28492=DIRECTION('',(0.158387039627108,0.,0.987377104088484));
#28493=DIRECTION('',(0.270257320503068,0.,-0.962788128673439));
#28494=DIRECTION('',(0.350061695092817,0.,-0.936726646161378));
#28495=DIRECTION('',(0.418575680773335,0.,-0.908181919807446));
#28496=DIRECTION('',(0.479172366105872,0.,-0.877720823246493));
#28497=DIRECTION('',(0.533692509635919,0.,-0.845678606302959));
#28498=DIRECTION('',(0.583265564466523,0.,-0.812281528355501));
#28499=DIRECTION('',(0.99975313641205,0.,-0.0222186010871085));
#28500=DIRECTION('',(0.999972569709231,0.,-0.00740674213917776));
#28501=DIRECTION('',(0.999972569709231,0.,0.00740674213917776));
#28502=DIRECTION('',(0.99975313641205,0.,0.0222186010871084));
#28503=DIRECTION('',(0.583265564466523,0.,0.812281528355501));
#28504=DIRECTION('',(0.533692509635919,0.,0.845678606302959));
#28505=DIRECTION('',(0.479172366105872,0.,0.877720823246493));
#28506=DIRECTION('',(0.418575680773335,0.,0.908181919807446));
#28507=DIRECTION('',(0.350061695092817,0.,0.936726646161378));
#28508=DIRECTION('',(0.270257320503068,0.,0.962788128673439));
#28509=DIRECTION('',(0.158387039627108,0.,-0.987377104088484));
#28510=DIRECTION('',(0.977941578718451,0.,0.208878597787478));
#28511=DIRECTION('',(0.951361549480978,0.,0.308076617368396));
#28512=DIRECTION('',(-0.356521352096954,0.,0.934287175069293));
#28513=DIRECTION('',(0.715443769451087,0.,-0.698670317641747));
#28514=DIRECTION('',(0.771525643922913,0.,-0.63619822443114));
#28515=DIRECTION('',(0.816588132859796,0.,-0.577220773424304));
#28516=DIRECTION('',(0.853835853462428,0.,-0.520542347309119));
#28517=DIRECTION('',(0.885030574305657,0.,-0.465532901677421));
#28518=DIRECTION('',(0.911263560158431,0.,-0.411823656347449));
#28519=DIRECTION('',(0.876920914189562,0.,0.480634695228032));
#28520=DIRECTION('',(0.869705019525386,0.,0.493571858002812));
#28521=DIRECTION('',(0.862298277386212,0.,0.506400711706423));
#28522=DIRECTION('',(0.85470231310245,0.,0.519118441184015));
#28523=DIRECTION('',(0.0989820318029246,0.,0.995089220813975));
#28524=DIRECTION('',(0.0393519680027008,0.,0.999225411313341));
#28525=DIRECTION('',(-0.0238849697840649,0.,0.999714713414989));
#28526=DIRECTION('',(-0.0915937869476482,0.,0.995796454197638));
#28527=DIRECTION('',(-0.165201002238466,0.,0.986259919523959));
#28528=DIRECTION('',(-0.247344359222354,0.,0.968927638144812));
#28529=DIRECTION('',(0.63085575199153,0.,-0.775900135442185));
#28530=DIRECTION('',(0.742482951693498,0.,0.669864961350055));
#28531=DIRECTION('',(0.669864961350055,0.,0.742482951693498));
#28532=DIRECTION('',(-0.775900135442185,0.,0.63085575199153));
#28533=DIRECTION('',(0.968927638144813,0.,-0.247344359222349));
#28534=DIRECTION('',(0.986259919523959,0.,-0.165201002238466));
#28535=DIRECTION('',(0.995796454197638,0.,-0.0915937869476553));
#28536=DIRECTION('',(0.999714713414989,0.,-0.0238849697840649));
#28537=DIRECTION('',(0.99922541131334,0.,0.039351968002701));
#28538=DIRECTION('',(0.995089220813975,0.,0.0989820318029272));
#28539=DIRECTION('',(0.519118441184011,0.,0.854702313102452));
#28540=DIRECTION('',(0.506400711706425,0.,0.862298277386211));
#28541=DIRECTION('',(0.493571858002802,0.,0.869705019525391));
#28542=DIRECTION('',(0.480634695228039,0.,0.876920914189558));
#28543=DIRECTION('',(-0.411823656347455,0.,0.911263560158428));
#28544=DIRECTION('',(-0.465532901677421,0.,0.885030574305657));
#28545=DIRECTION('',(-0.520542347309117,0.,0.853835853462429));
#28546=DIRECTION('',(-0.577220773424305,0.,0.816588132859795));
#28547=DIRECTION('',(-0.636198224431141,0.,0.771525643922912));
#28548=DIRECTION('',(-0.698670317641746,0.,0.715443769451088));
#28549=DIRECTION('',(0.934287175069293,0.,-0.356521352096954));
#28550=DIRECTION('',(0.308076617368396,0.,0.951361549480978));
#28551=DIRECTION('',(0.208878597787478,0.,0.977941578718451));
#28552=DIRECTION('',(-0.987377104088484,0.,0.158387039627108));
#28553=DIRECTION('',(0.962788128673439,0.,0.270257320503068));
#28554=DIRECTION('',(0.936726646161378,0.,0.350061695092817));
#28555=DIRECTION('',(0.908181919807447,0.,0.418575680773333));
#28556=DIRECTION('',(0.877720823246493,0.,0.479172366105871));
#28557=DIRECTION('',(0.845678606302959,0.,0.533692509635919));
#28558=DIRECTION('',(0.812281528355501,0.,0.583265564466523));
#28559=DIRECTION('',(0.0222186010871084,0.,0.99975313641205));
#28560=DIRECTION('',(0.00740674213917775,0.,0.999972569709231));
#28561=DIRECTION('',(-0.00740674213917775,0.,0.999972569709231));
#28562=DIRECTION('',(-0.0222186010871084,0.,0.99975313641205));
#28563=DIRECTION('',(-0.812281528355501,0.,0.583265564466523));
#28564=DIRECTION('',(-0.845678606302959,0.,0.533692509635919));
#28565=DIRECTION('',(-0.877720823246493,0.,0.479172366105871));
#28566=DIRECTION('',(-0.908181919807447,0.,0.418575680773333));
#28567=DIRECTION('',(-0.936726646161378,0.,0.350061695092817));
#28568=DIRECTION('',(-0.962788128673439,0.,0.270257320503068));
#28569=DIRECTION('',(0.987377104088484,0.,0.158387039627108));
#28570=DIRECTION('',(-0.208878597787478,0.,0.977941578718451));
#28571=DIRECTION('',(-0.308076617368396,0.,0.951361549480978));
#28572=DIRECTION('',(-0.934287175069293,0.,-0.356521352096954));
#28573=DIRECTION('',(0.698670317641746,0.,0.715443769451088));
#28574=DIRECTION('',(0.636198224431141,0.,0.771525643922912));
#28575=DIRECTION('',(0.577220773424305,0.,0.816588132859795));
#28576=DIRECTION('',(0.520542347309117,0.,0.853835853462429));
#28577=DIRECTION('',(0.465532901677421,0.,0.885030574305657));
#28578=DIRECTION('',(0.411823656347455,0.,0.911263560158428));
#28579=DIRECTION('',(-0.480634695228039,0.,0.876920914189558));
#28580=DIRECTION('',(-0.493571858002802,0.,0.869705019525391));
#28581=DIRECTION('',(-0.506400711706425,0.,0.862298277386211));
#28582=DIRECTION('',(-0.519118441184011,0.,0.854702313102452));
#28583=DIRECTION('',(-0.995089220813975,0.,0.0989820318029272));
#28584=DIRECTION('',(-0.99922541131334,0.,0.039351968002701));
#28585=DIRECTION('',(-0.999714713414989,0.,-0.0238849697840649));
#28586=DIRECTION('',(-0.995796454197638,0.,-0.0915937869476553));
#28587=DIRECTION('',(-0.986259919523959,0.,-0.165201002238466));
#28588=DIRECTION('',(-0.968927638144813,0.,-0.247344359222349));
#28589=DIRECTION('',(0.775900135442185,0.,0.63085575199153));
#28590=DIRECTION('',(-0.669864961350055,0.,0.742482951693498));
#28591=DIRECTION('',(-0.742482951693498,0.,0.669864961350055));
#28592=DIRECTION('',(-0.63085575199153,0.,-0.775900135442185));
#28593=DIRECTION('',(0.247344359222354,0.,0.968927638144812));
#28594=DIRECTION('',(0.165201002238466,0.,0.986259919523959));
#28595=DIRECTION('',(0.0915937869476482,0.,0.995796454197638));
#28596=DIRECTION('',(0.0238849697840649,0.,0.999714713414989));
#28597=DIRECTION('',(-0.0393519680027008,0.,0.999225411313341));
#28598=DIRECTION('',(-0.0989820318029246,0.,0.995089220813975));
#28599=DIRECTION('',(-0.85470231310245,0.,0.519118441184015));
#28600=DIRECTION('',(-0.862298277386212,0.,0.506400711706423));
#28601=DIRECTION('',(-0.869705019525386,0.,0.493571858002812));
#28602=DIRECTION('',(-0.876920914189562,0.,0.480634695228032));
#28603=DIRECTION('',(-0.911263560158431,0.,-0.411823656347449));
#28604=DIRECTION('',(-0.885030574305657,0.,-0.465532901677421));
#28605=DIRECTION('',(-0.853835853462428,0.,-0.520542347309119));
#28606=DIRECTION('',(-0.816588132859796,0.,-0.577220773424304));
#28607=DIRECTION('',(-0.771525643922913,0.,-0.63619822443114));
#28608=DIRECTION('',(-0.715443769451087,0.,-0.698670317641747));
#28609=DIRECTION('',(0.356521352096954,0.,0.934287175069293));
#28610=DIRECTION('',(-0.951361549480978,0.,0.308076617368396));
#28611=DIRECTION('',(-0.977941578718451,0.,0.208878597787478));
#28612=DIRECTION('',(-0.158387039627108,0.,-0.987377104088484));
#28613=DIRECTION('',(-0.270257320503068,0.,0.962788128673439));
#28614=DIRECTION('',(-0.350061695092817,0.,0.936726646161378));
#28615=DIRECTION('',(-0.418575680773335,0.,0.908181919807446));
#28616=DIRECTION('',(-0.479172366105872,0.,0.877720823246493));
#28617=DIRECTION('',(-0.533692509635919,0.,0.845678606302959));
#28618=DIRECTION('',(-0.583265564466523,0.,0.812281528355501));
#28619=DIRECTION('',(-0.99975313641205,0.,0.0222186010871084));
#28620=DIRECTION('',(-0.999972569709231,0.,0.00740674213917776));
#28621=DIRECTION('',(-0.999972569709231,0.,-0.00740674213917776));
#28622=DIRECTION('',(-0.99975313641205,0.,-0.0222186010871085));
#28623=DIRECTION('',(-0.583265564466523,0.,-0.812281528355501));
#28624=DIRECTION('',(-0.533692509635919,0.,-0.845678606302959));
#28625=DIRECTION('',(-0.479172366105872,0.,-0.877720823246493));
#28626=DIRECTION('',(-0.418575680773335,0.,-0.908181919807446));
#28627=DIRECTION('',(-0.350061695092817,0.,-0.936726646161378));
#28628=DIRECTION('',(-0.270257320503068,0.,-0.962788128673439));
#28629=DIRECTION('',(-0.158387039627108,0.,0.987377104088484));
#28630=DIRECTION('',(-0.977941578718451,0.,-0.208878597787479));
#28631=DIRECTION('',(-0.951361549480978,0.,-0.308076617368397));
#28632=DIRECTION('',(0.356521352096954,0.,-0.934287175069293));
#28633=DIRECTION('',(-0.715443769451089,0.,0.698670317641745));
#28634=DIRECTION('',(-0.771525643922911,0.,0.636198224431142));
#28635=DIRECTION('',(-0.816588132859795,0.,0.577220773424306));
#28636=DIRECTION('',(-0.853835853462428,0.,0.520542347309119));
#28637=DIRECTION('',(-0.885030574305657,0.,0.46553290167742));
#28638=DIRECTION('',(-0.911263560158429,0.,0.411823656347453));
#28639=DIRECTION('',(-0.876920914189557,0.,-0.48063469522804));
#28640=DIRECTION('',(-0.86970501952539,0.,-0.493571858002805));
#28641=DIRECTION('',(-0.86229827738621,0.,-0.506400711706427));
#28642=DIRECTION('',(-0.85470231310245,0.,-0.519118441184015));
#28643=DIRECTION('',(-0.0989820318029307,0.,-0.995089220813975));
#28644=DIRECTION('',(-0.0393519680026975,0.,-0.999225411313341));
#28645=DIRECTION('',(0.0238849697840614,0.,-0.99971471341499));
#28646=DIRECTION('',(0.0915937869476591,0.,-0.995796454197637));
#28647=DIRECTION('',(0.165201002238462,0.,-0.98625991952396));
#28648=DIRECTION('',(0.247344359222349,0.,-0.968927638144813));
#28649=DIRECTION('',(-0.63085575199153,0.,0.775900135442185));
#28650=DIRECTION('',(-0.742482951693498,0.,-0.669864961350055));
#28651=DIRECTION('',(-0.669864961350055,0.,-0.742482951693498));
#28652=DIRECTION('',(0.775900135442185,0.,-0.63085575199153));
#28653=DIRECTION('',(-0.968927638144812,0.,0.247344359222352));
#28654=DIRECTION('',(-0.98625991952396,0.,0.165201002238459));
#28655=DIRECTION('',(-0.995796454197637,0.,0.0915937869476627));
#28656=DIRECTION('',(-0.99971471341499,0.,0.0238849697840613));
#28657=DIRECTION('',(-0.999225411313341,0.,-0.0393519680026977));
#28658=DIRECTION('',(-0.995089220813975,0.,-0.0989820318029304));
#28659=DIRECTION('',(-0.519118441184006,0.,-0.854702313102456));
#28660=DIRECTION('',(-0.506400711706431,0.,-0.862298277386207));
#28661=DIRECTION('',(-0.493571858002802,0.,-0.869705019525391));
#28662=DIRECTION('',(-0.480634695228042,0.,-0.876920914189556));
#28663=DIRECTION('',(0.41182365634745,0.,-0.91126356015843));
#28664=DIRECTION('',(0.465532901677425,0.,-0.885030574305655));
#28665=DIRECTION('',(0.520542347309115,0.,-0.85383585346243));
#28666=DIRECTION('',(0.577220773424311,0.,-0.816588132859791));
#28667=DIRECTION('',(0.636198224431136,0.,-0.771525643922916));
#28668=DIRECTION('',(0.698670317641747,0.,-0.715443769451087));
#28669=DIRECTION('',(-0.934287175069293,0.,0.356521352096954));
#28670=DIRECTION('',(-0.308076617368396,0.,-0.951361549480978));
#28671=DIRECTION('',(-0.20887859778748,0.,-0.977941578718451));
#28672=DIRECTION('',(0.987377104088484,0.,-0.158387039627109));
#28673=DIRECTION('',(-0.962788128673439,0.,-0.270257320503066));
#28674=DIRECTION('',(-0.936726646161376,0.,-0.350061695092823));
#28675=DIRECTION('',(-0.908181919807451,0.,-0.418575680773325));
#28676=DIRECTION('',(-0.87772082324649,0.,-0.479172366105876));
#28677=DIRECTION('',(-0.84567860630296,0.,-0.533692509635917));
#28678=DIRECTION('',(-0.8122815283555,0.,-0.583265564466524));
#28679=DIRECTION('',(-0.0222186010871084,0.,-0.99975313641205));
#28680=DIRECTION('',(-0.00740674213917776,0.,-0.999972569709231));
#28681=DIRECTION('',(0.00740674213917776,0.,-0.999972569709231));
#28682=DIRECTION('',(0.0222186010871084,0.,-0.99975313641205));
#28683=DIRECTION('',(0.812281528355498,0.,-0.583265564466527));
#28684=DIRECTION('',(0.845678606302961,0.,-0.533692509635915));
#28685=DIRECTION('',(0.87772082324649,0.,-0.479172366105876));
#28686=DIRECTION('',(0.908181919807451,0.,-0.418575680773326));
#28687=DIRECTION('',(0.936726646161376,0.,-0.350061695092823));
#28688=DIRECTION('',(0.962788128673439,0.,-0.270257320503067));
#28689=DIRECTION('',(-0.987377104088484,0.,-0.158387039627108));
#28690=DIRECTION('',(0.208878597787478,0.,-0.977941578718451));
#28691=DIRECTION('',(0.308076617368396,0.,-0.951361549480978));
#28692=DIRECTION('',(0.934287175069293,0.,0.356521352096954));
#28693=DIRECTION('',(-0.69867031764175,0.,-0.715443769451084));
#28694=DIRECTION('',(-0.636198224431135,0.,-0.771525643922917));
#28695=DIRECTION('',(-0.577220773424313,0.,-0.81658813285979));
#28696=DIRECTION('',(-0.520542347309115,0.,-0.85383585346243));
#28697=DIRECTION('',(-0.465532901677422,0.,-0.885030574305656));
#28698=DIRECTION('',(-0.411823656347447,0.,-0.911263560158432));
#28699=DIRECTION('',(0.48063469522803,0.,-0.876920914189563));
#28700=DIRECTION('',(0.493571858002814,0.,-0.869705019525385));
#28701=DIRECTION('',(0.506400711706419,0.,-0.862298277386214));
#28702=DIRECTION('',(0.519118441184019,0.,-0.854702313102448));
#28703=DIRECTION('',(0.995089220813975,0.,-0.0989820318029307));
#28704=DIRECTION('',(0.999225411313341,0.,-0.0393519680026942));
#28705=DIRECTION('',(0.99971471341499,0.,0.023884969784058));
#28706=DIRECTION('',(0.995796454197637,0.,0.091593786947663));
#28707=DIRECTION('',(0.986259919523961,0.,0.165201002238458));
#28708=DIRECTION('',(0.968927638144812,0.,0.247344359222354));
#28709=DIRECTION('',(-0.775900135442185,0.,-0.630855751991531));
#28710=DIRECTION('',(0.669864961350053,0.,-0.742482951693499));
#28711=DIRECTION('center_axis',(0.,-1.,0.));
#28712=DIRECTION('ref_axis',(0.,0.,1.));
#28713=DIRECTION('center_axis',(-0.968927638144818,0.,0.247344359222329));
#28714=DIRECTION('ref_axis',(0.247344359222329,0.,0.968927638144818));
#28715=DIRECTION('',(0.,1.,0.));
#28716=DIRECTION('',(0.228100862670962,-0.386714295024757,0.893544654996195));
#28717=DIRECTION('',(0.247344359222329,0.,0.968927638144818));
#28718=DIRECTION('',(0.,1.,0.));
#28719=DIRECTION('center_axis',(-0.938956260693934,0.,0.344036539489144));
#28720=DIRECTION('ref_axis',(0.344036539489144,0.,0.938956260693934));
#28721=DIRECTION('',(0.,1.,0.));
#28722=DIRECTION('',(0.327151215534528,-0.309436927624306,0.892872258498779));
#28723=DIRECTION('center_axis',(-0.252098665705552,-0.707106781186548,0.660640797067119));
#28724=DIRECTION('ref_axis',(0.934287175069293,0.,0.356521352096954));
#28725=DIRECTION('',(-0.64431346919632,-0.386714295024737,-0.659781939307013));
#28726=DIRECTION('',(0.217986803358223,-0.706639907076675,-0.673158076003201));
#28727=DIRECTION('',(-0.934287175069293,0.,-0.356521352096954));
#28728=DIRECTION('',(-0.841793968866839,-0.176491388068509,-0.510131065430313));
#28729=DIRECTION('',(-0.729757392781244,-0.309436927624312,-0.609674450427068));
#28730=DIRECTION('center_axis',(-0.715443769451084,0.,0.69867031764175));
#28731=DIRECTION('ref_axis',(0.69867031764175,0.,0.715443769451084));
#28732=DIRECTION('',(0.,1.,0.));
#28733=DIRECTION('',(0.64431346919632,-0.386714295024737,0.659781939307013));
#28734=DIRECTION('',(0.69867031764175,0.,0.715443769451084));
#28735=DIRECTION('',(0.,1.,0.));
#28736=DIRECTION('center_axis',(-0.641141705058825,0.,0.767422513374649));
#28737=DIRECTION('ref_axis',(0.767422513374649,0.,0.641141705058824));
#28738=DIRECTION('',(0.,1.,0.));
#28739=DIRECTION('',(0.729757392781244,-0.309436927624312,0.609674450427068));
#28740=DIRECTION('center_axis',(0.111996549772391,-0.707106781186548,0.698181045889302));
#28741=DIRECTION('ref_axis',(0.987377104088484,0.,-0.158387039627109));
#28742=DIRECTION('',(-0.887882801977999,-0.386714295024741,-0.24923118579988));
#28743=DIRECTION('',(-0.147796928603617,-0.706639907076676,-0.691965396260539));
#28744=DIRECTION('',(-0.987377104088484,0.,0.158387039627109));
#28745=DIRECTION('',(-0.984080494506366,-0.176491388068509,-0.0208894774888531));
#28746=DIRECTION('',(-0.936825665961593,-0.309436927624307,-0.16311486571753));
#28747=DIRECTION('center_axis',(-0.270257320503066,0.,0.962788128673439));
#28748=DIRECTION('ref_axis',(0.962788128673439,0.,0.270257320503066));
#28749=DIRECTION('',(0.,1.,0.));
#28750=DIRECTION('',(0.887882801977999,-0.386714295024741,0.24923118579988));
#28751=DIRECTION('',(0.962788128673439,0.,0.270257320503066));
#28752=DIRECTION('',(0.,1.,0.));
#28753=DIRECTION('center_axis',(-0.171533747319281,0.,0.985178244547963));
#28754=DIRECTION('ref_axis',(0.985178244547962,0.,0.171533747319281));
#28755=DIRECTION('',(0.,1.,0.));
#28756=DIRECTION('',(0.936825665961593,-0.309436927624307,0.16311486571753));
#28757=DIRECTION('center_axis',(0.446082380183749,-0.70710678118655,0.548644247294728));
#28758=DIRECTION('ref_axis',(0.775900135442185,0.,-0.63085575199153));
#28759=DIRECTION('',(-0.893544654996196,-0.386714295024739,0.228100862670985));
#28760=DIRECTION('',(-0.473978592902318,-0.706639907076674,-0.525361147399585));
#28761=DIRECTION('',(-0.775900135442185,0.,0.63085575199153));
#28762=DIRECTION('',(-0.862683446355692,-0.176491388068509,0.473949429076052));
#28763=DIRECTION('',(-0.892872258498779,-0.309436927624306,0.327151215534528));
#28764=DIRECTION('center_axis',(0.247344359222352,0.,0.968927638144812));
#28765=DIRECTION('ref_axis',(0.968927638144812,0.,-0.247344359222352));
#28766=DIRECTION('',(0.,1.,0.));
#28767=DIRECTION('',(0.893544654996196,-0.386714295024739,-0.228100862670985));
#28768=DIRECTION('',(0.968927638144812,0.,-0.247344359222352));
#28769=DIRECTION('',(0.,1.,0.));
#28770=DIRECTION('center_axis',(0.344036539489143,0.,0.938956260693934));
#28771=DIRECTION('ref_axis',(0.938956260693934,0.,-0.344036539489143));
#28772=DIRECTION('',(0.,1.,0.));
#28773=DIRECTION('',(0.892872258498779,-0.309436927624306,-0.327151215534528));
#28774=DIRECTION('center_axis',(0.660640797067119,-0.707106781186549,0.252098665705552));
#28775=DIRECTION('ref_axis',(0.356521352096954,0.,-0.934287175069293));
#28776=DIRECTION('',(-0.659781939307016,-0.386714295024741,0.644313469196315));
#28777=DIRECTION('',(-0.673158076003201,-0.706639907076675,-0.217986803358224));
#28778=DIRECTION('',(-0.356521352096954,0.,0.934287175069293));
#28779=DIRECTION('',(-0.510131065430304,-0.176491388068498,0.841793968866847));
#28780=DIRECTION('',(-0.609674450427068,-0.309436927624311,0.729757392781245));
#28781=DIRECTION('center_axis',(0.698670317641745,0.,0.715443769451089));
#28782=DIRECTION('ref_axis',(0.715443769451089,0.,-0.698670317641745));
#28783=DIRECTION('',(0.,1.,0.));
#28784=DIRECTION('',(0.659781939307016,-0.386714295024741,-0.644313469196315));
#28785=DIRECTION('',(0.715443769451089,0.,-0.698670317641745));
#28786=DIRECTION('',(0.,1.,0.));
#28787=DIRECTION('center_axis',(0.76742251337465,0.,0.641141705058824));
#28788=DIRECTION('ref_axis',(0.641141705058824,0.,-0.76742251337465));
#28789=DIRECTION('',(0.,1.,0.));
#28790=DIRECTION('',(0.609674450427068,-0.309436927624311,-0.729757392781245));
#28791=DIRECTION('center_axis',(0.698181045889302,-0.707106781186549,-0.11199654977239));
#28792=DIRECTION('ref_axis',(-0.158387039627108,0.,-0.987377104088484));
#28793=DIRECTION('',(-0.249231185799881,-0.386714295024742,0.887882801977999));
#28794=DIRECTION('',(-0.691965396260539,-0.706639907076675,0.147796928603616));
#28795=DIRECTION('',(0.158387039627108,0.,0.987377104088484));
#28796=DIRECTION('',(-0.0208894774888416,-0.176491388068498,0.984080494506368));
#28797=DIRECTION('',(-0.163114865717534,-0.309436927624311,0.936825665961591));
#28798=DIRECTION('center_axis',(0.962788128673439,0.,0.270257320503068));
#28799=DIRECTION('ref_axis',(0.270257320503068,0.,-0.962788128673439));
#28800=DIRECTION('',(0.,1.,0.));
#28801=DIRECTION('',(0.249231185799881,-0.386714295024742,-0.887882801977999));
#28802=DIRECTION('',(0.270257320503068,0.,-0.962788128673439));
#28803=DIRECTION('',(0.,1.,0.));
#28804=DIRECTION('center_axis',(0.985178244547962,0.,0.171533747319286));
#28805=DIRECTION('ref_axis',(0.171533747319286,0.,-0.985178244547962));
#28806=DIRECTION('',(0.,1.,0.));
#28807=DIRECTION('',(0.163114865717534,-0.309436927624311,-0.936825665961591));
#28808=DIRECTION('center_axis',(0.548644247294728,-0.70710678118655,-0.446082380183749));
#28809=DIRECTION('ref_axis',(-0.63085575199153,0.,-0.775900135442185));
#28810=DIRECTION('',(0.228100862670987,-0.386714295024738,0.893544654996197));
#28811=DIRECTION('',(-0.525361147399585,-0.706639907076674,0.473978592902318));
#28812=DIRECTION('',(0.63085575199153,0.,0.775900135442185));
#28813=DIRECTION('',(0.473949429076065,-0.176491388068497,0.862683446355688));
#28814=DIRECTION('',(0.327151215534519,-0.309436927624313,0.89287225849878));
#28815=DIRECTION('center_axis',(0.968927638144812,0.,-0.247344359222354));
#28816=DIRECTION('ref_axis',(-0.247344359222354,0.,-0.968927638144812));
#28817=DIRECTION('',(0.,1.,0.));
#28818=DIRECTION('',(-0.228100862670987,-0.386714295024738,-0.893544654996197));
#28819=DIRECTION('',(-0.247344359222354,0.,-0.968927638144812));
#28820=DIRECTION('',(0.,1.,0.));
#28821=DIRECTION('center_axis',(0.938956260693937,0.,-0.344036539489135));
#28822=DIRECTION('ref_axis',(-0.344036539489135,0.,-0.938956260693937));
#28823=DIRECTION('',(0.,1.,0.));
#28824=DIRECTION('',(-0.327151215534519,-0.309436927624313,-0.89287225849878));
#28825=DIRECTION('center_axis',(0.252098665705552,-0.707106781186548,-0.660640797067119));
#28826=DIRECTION('ref_axis',(-0.934287175069293,0.,-0.356521352096954));
#28827=DIRECTION('',(0.644313469196316,-0.386714295024741,0.659781939307015));
#28828=DIRECTION('',(-0.217986803358223,-0.706639907076675,0.673158076003201));
#28829=DIRECTION('',(0.934287175069293,0.,0.356521352096954));
#28830=DIRECTION('',(0.841793968866845,-0.1764913880685,0.510131065430306));
#28831=DIRECTION('',(0.729757392781242,-0.309436927624314,0.609674450427069));
#28832=DIRECTION('center_axis',(0.715443769451088,0.,-0.698670317641746));
#28833=DIRECTION('ref_axis',(-0.698670317641746,0.,-0.715443769451088));
#28834=DIRECTION('',(0.,1.,0.));
#28835=DIRECTION('',(-0.644313469196316,-0.386714295024741,-0.659781939307015));
#28836=DIRECTION('',(-0.698670317641746,0.,-0.715443769451088));
#28837=DIRECTION('',(0.,1.,0.));
#28838=DIRECTION('center_axis',(0.641141705058826,0.,-0.767422513374648));
#28839=DIRECTION('ref_axis',(-0.767422513374648,0.,-0.641141705058826));
#28840=DIRECTION('',(0.,1.,0.));
#28841=DIRECTION('',(-0.729757392781242,-0.309436927624314,-0.609674450427069));
#28842=DIRECTION('center_axis',(-0.11199654977239,-0.707106781186549,-0.698181045889302));
#28843=DIRECTION('ref_axis',(-0.987377104088484,0.,0.158387039627108));
#28844=DIRECTION('',(0.887882801977998,-0.386714295024742,0.249231185799882));
#28845=DIRECTION('',(0.147796928603616,-0.706639907076675,0.691965396260539));
#28846=DIRECTION('',(0.987377104088484,0.,-0.158387039627108));
#28847=DIRECTION('',(0.984080494506367,-0.176491388068501,0.0208894774888451));
#28848=DIRECTION('',(0.936825665961591,-0.309436927624309,0.163114865717533));
#28849=DIRECTION('center_axis',(0.270257320503069,0.,-0.962788128673439));
#28850=DIRECTION('ref_axis',(-0.962788128673439,0.,-0.270257320503069));
#28851=DIRECTION('',(0.,1.,0.));
#28852=DIRECTION('',(-0.887882801977998,-0.386714295024742,-0.249231185799882));
#28853=DIRECTION('',(-0.962788128673439,0.,-0.270257320503068));
#28854=DIRECTION('',(0.,1.,0.));
#28855=DIRECTION('center_axis',(0.171533747319284,0.,-0.985178244547962));
#28856=DIRECTION('ref_axis',(-0.985178244547962,0.,-0.171533747319284));
#28857=DIRECTION('',(0.,1.,0.));
#28858=DIRECTION('',(-0.936825665961591,-0.309436927624309,-0.163114865717533));
#28859=DIRECTION('center_axis',(-0.446082380183748,-0.707106781186549,-0.548644247294729));
#28860=DIRECTION('ref_axis',(-0.775900135442186,0.,0.63085575199153));
#28861=DIRECTION('',(0.893544654996196,-0.386714295024742,-0.228100862670982));
#28862=DIRECTION('',(0.473978592902317,-0.706639907076675,0.525361147399585));
#28863=DIRECTION('',(0.775900135442185,0.,-0.63085575199153));
#28864=DIRECTION('',(0.862683446355689,-0.176491388068498,-0.473949429076063));
#28865=DIRECTION('',(0.89287225849878,-0.30943692762431,-0.327151215534523));
#28866=DIRECTION('center_axis',(-0.247344359222349,0.,-0.968927638144813));
#28867=DIRECTION('ref_axis',(-0.968927638144813,0.,0.247344359222349));
#28868=DIRECTION('',(0.,1.,0.));
#28869=DIRECTION('',(-0.893544654996196,-0.386714295024742,0.228100862670982));
#28870=DIRECTION('',(-0.968927638144813,0.,0.247344359222349));
#28871=DIRECTION('',(0.,1.,0.));
#28872=DIRECTION('center_axis',(-0.344036539489138,0.,-0.938956260693936));
#28873=DIRECTION('ref_axis',(-0.938956260693936,0.,0.344036539489138));
#28874=DIRECTION('',(0.,1.,0.));
#28875=DIRECTION('',(-0.89287225849878,-0.30943692762431,0.327151215534523));
#28876=DIRECTION('center_axis',(-0.660640797067119,-0.707106781186548,-0.252098665705553));
#28877=DIRECTION('ref_axis',(-0.356521352096954,0.,0.934287175069293));
#28878=DIRECTION('',(0.659781939307015,-0.386714295024739,-0.644313469196317));
#28879=DIRECTION('',(0.673158076003201,-0.706639907076675,0.217986803358222));
#28880=DIRECTION('',(0.356521352096954,0.,-0.934287175069293));
#28881=DIRECTION('',(0.510131065430303,-0.176491388068496,-0.841793968866848));
#28882=DIRECTION('',(0.60967445042707,-0.309436927624314,-0.729757392781241));
#28883=DIRECTION('center_axis',(-0.698670317641747,0.,-0.715443769451087));
#28884=DIRECTION('ref_axis',(-0.715443769451087,0.,0.698670317641747));
#28885=DIRECTION('',(0.,1.,0.));
#28886=DIRECTION('',(-0.659781939307015,-0.386714295024739,0.644313469196317));
#28887=DIRECTION('',(-0.715443769451087,0.,0.698670317641747));
#28888=DIRECTION('',(0.,1.,0.));
#28889=DIRECTION('center_axis',(-0.767422513374647,0.,-0.641141705058827));
#28890=DIRECTION('ref_axis',(-0.641141705058827,0.,0.767422513374647));
#28891=DIRECTION('',(0.,1.,0.));
#28892=DIRECTION('',(-0.60967445042707,-0.309436927624314,0.729757392781241));
#28893=DIRECTION('center_axis',(-0.698181045889302,-0.707106781186549,0.111996549772391));
#28894=DIRECTION('ref_axis',(0.158387039627108,0.,0.987377104088484));
#28895=DIRECTION('',(0.249231185799882,-0.386714295024742,-0.887882801977999));
#28896=DIRECTION('',(0.691965396260539,-0.706639907076675,-0.147796928603617));
#28897=DIRECTION('',(-0.158387039627108,0.,-0.987377104088484));
#28898=DIRECTION('',(0.0208894774888421,-0.176491388068498,-0.984080494506368));
#28899=DIRECTION('',(0.163114865717534,-0.309436927624311,-0.936825665961591));
#28900=DIRECTION('center_axis',(-0.962788128673439,0.,-0.270257320503068));
#28901=DIRECTION('ref_axis',(-0.270257320503068,0.,0.962788128673439));
#28902=DIRECTION('',(0.,1.,0.));
#28903=DIRECTION('',(-0.249231185799882,-0.386714295024742,0.887882801977999));
#28904=DIRECTION('',(-0.270257320503068,0.,0.962788128673439));
#28905=DIRECTION('',(0.,1.,0.));
#28906=DIRECTION('center_axis',(-0.985178244547962,0.,-0.171533747319286));
#28907=DIRECTION('ref_axis',(-0.171533747319286,0.,0.985178244547962));
#28908=DIRECTION('',(0.,1.,0.));
#28909=DIRECTION('',(-0.163114865717534,-0.309436927624311,0.936825665961591));
#28910=DIRECTION('center_axis',(0.660640797067119,-0.707106781186549,-0.252098665705553));
#28911=DIRECTION('ref_axis',(-0.356521352096954,0.,-0.934287175069293));
#28912=DIRECTION('',(0.510131065430303,0.176491388068496,0.841793968866848));
#28913=DIRECTION('',(0.356521352096954,0.,0.934287175069293));
#28914=DIRECTION('',(0.673158076003201,0.706639907076675,-0.217986803358222));
#28915=DIRECTION('',(0.659781939307025,0.386714295024756,0.644313469196296));
#28916=DIRECTION('',(0.609674450427067,0.309436927624308,0.729757392781247));
#28917=DIRECTION('center_axis',(0.934287175069293,0.,-0.356521352096954));
#28918=DIRECTION('ref_axis',(-0.356521352096954,0.,-0.934287175069293));
#28919=DIRECTION('',(0.,1.,0.));
#28920=DIRECTION('',(-0.356521352096954,0.,-0.934287175069293));
#28921=DIRECTION('',(0.,1.,0.));
#28922=DIRECTION('center_axis',(0.855219039771101,0.,-0.518266720919833));
#28923=DIRECTION('ref_axis',(-0.518266720919833,0.,-0.855219039771101));
#28924=DIRECTION('',(0.,1.,0.));
#28925=DIRECTION('',(-0.510131065430303,0.176491388068496,-0.841793968866848));
#28926=DIRECTION('center_axis',(0.446082380183749,-0.70710678118655,-0.548644247294728));
#28927=DIRECTION('ref_axis',(-0.775900135442185,0.,-0.630855751991531));
#28928=DIRECTION('',(0.862683446355692,0.176491388068508,0.473949429076054));
#28929=DIRECTION('',(0.775900135442185,0.,0.630855751991531));
#28930=DIRECTION('',(0.473978592902316,0.706639907076674,-0.525361147399586));
#28931=DIRECTION('',(0.893544654996196,0.386714295024738,0.228100862670987));
#28932=DIRECTION('',(0.892872258498779,0.309436927624308,0.327151215534526));
#28933=DIRECTION('center_axis',(0.630855751991531,0.,-0.775900135442185));
#28934=DIRECTION('ref_axis',(-0.775900135442185,0.,-0.630855751991531));
#28935=DIRECTION('',(0.,1.,0.));
#28936=DIRECTION('',(-0.775900135442185,0.,-0.630855751991531));
#28937=DIRECTION('',(0.,1.,0.));
#28938=DIRECTION('center_axis',(0.481508053781981,0.,-0.876441666138191));
#28939=DIRECTION('ref_axis',(-0.876441666138191,0.,-0.481508053781981));
#28940=DIRECTION('',(0.,1.,0.));
#28941=DIRECTION('',(-0.862683446355692,0.176491388068508,-0.473949429076054));
#28942=DIRECTION('center_axis',(0.11199654977239,-0.707106781186549,-0.698181045889302));
#28943=DIRECTION('ref_axis',(-0.987377104088484,0.,-0.158387039627108));
#28944=DIRECTION('',(0.984080494506366,0.17649138806851,-0.020889477488854));
#28945=DIRECTION('',(0.987377104088484,0.,0.158387039627108));
#28946=DIRECTION('',(0.147796928603616,0.706639907076675,-0.691965396260539));
#28947=DIRECTION('',(0.887882801977999,0.386714295024741,-0.249231185799881));
#28948=DIRECTION('',(0.936825665961593,0.309436927624307,-0.16311486571753));
#28949=DIRECTION('center_axis',(0.158387039627108,0.,-0.987377104088484));
#28950=DIRECTION('ref_axis',(-0.987377104088484,0.,-0.158387039627108));
#28951=DIRECTION('',(0.,1.,0.));
#28952=DIRECTION('',(-0.987377104088484,0.,-0.158387039627108));
#28953=DIRECTION('',(0.,1.,0.));
#28954=DIRECTION('center_axis',(-0.0212226263670982,0.,-0.999774774701824));
#28955=DIRECTION('ref_axis',(-0.999774774701824,0.,0.0212226263670982));
#28956=DIRECTION('',(0.,1.,0.));
#28957=DIRECTION('',(-0.984080494506366,0.17649138806851,0.020889477488854));
#28958=DIRECTION('center_axis',(-0.252098665705553,-0.707106781186548,-0.66064079706712));
#28959=DIRECTION('ref_axis',(-0.934287175069293,0.,0.356521352096954));
#28960=DIRECTION('',(0.84179396886684,0.176491388068507,-0.510131065430311));
#28961=DIRECTION('',(0.934287175069293,0.,-0.356521352096954));
#28962=DIRECTION('',(-0.217986803358222,0.706639907076676,-0.6731580760032));
#28963=DIRECTION('',(0.644313469196317,0.38671429502474,-0.659781939307015));
#28964=DIRECTION('',(0.729757392781247,0.309436927624309,-0.609674450427066));
#28965=DIRECTION('center_axis',(-0.356521352096954,0.,-0.934287175069293));
#28966=DIRECTION('ref_axis',(-0.934287175069293,0.,0.356521352096954));
#28967=DIRECTION('',(0.,1.,0.));
#28968=DIRECTION('',(-0.934287175069293,0.,0.356521352096954));
#28969=DIRECTION('',(0.,1.,0.));
#28970=DIRECTION('center_axis',(-0.518266720919842,0.,-0.855219039771096));
#28971=DIRECTION('ref_axis',(-0.855219039771096,0.,0.518266720919842));
#28972=DIRECTION('',(0.,1.,0.));
#28973=DIRECTION('',(-0.84179396886684,0.176491388068507,0.510131065430311));
#28974=DIRECTION('center_axis',(-0.54864424729473,-0.707106781186548,-0.446082380183749));
#28975=DIRECTION('ref_axis',(-0.63085575199153,0.,0.775900135442186));
#28976=DIRECTION('',(0.473949429076053,0.176491388068509,-0.862683446355692));
#28977=DIRECTION('',(0.63085575199153,0.,-0.775900135442185));
#28978=DIRECTION('',(-0.525361147399584,0.706639907076676,-0.473978592902316));
#28979=DIRECTION('',(0.228100862670983,0.386714295024742,-0.893544654996196));
#28980=DIRECTION('',(0.327151215534528,0.309436927624306,-0.892872258498779));
#28981=DIRECTION('center_axis',(-0.775900135442186,0.,-0.63085575199153));
#28982=DIRECTION('ref_axis',(-0.63085575199153,0.,0.775900135442185));
#28983=DIRECTION('',(0.,1.,0.));
#28984=DIRECTION('',(-0.63085575199153,0.,0.775900135442185));
#28985=DIRECTION('',(0.,1.,0.));
#28986=DIRECTION('center_axis',(-0.876441666138192,0.,-0.48150805378198));
#28987=DIRECTION('ref_axis',(-0.48150805378198,0.,0.876441666138192));
#28988=DIRECTION('',(0.,1.,0.));
#28989=DIRECTION('',(-0.473949429076053,0.176491388068509,0.862683446355692));
#28990=DIRECTION('center_axis',(-0.698181045889302,-0.707106781186549,-0.111996549772391));
#28991=DIRECTION('ref_axis',(-0.158387039627108,0.,0.987377104088484));
#28992=DIRECTION('',(-0.0208894774888421,0.176491388068498,-0.984080494506368));
#28993=DIRECTION('',(0.158387039627108,0.,-0.987377104088484));
#28994=DIRECTION('',(-0.691965396260539,0.706639907076675,-0.147796928603617));
#28995=DIRECTION('',(-0.249231185799882,0.386714295024742,-0.887882801977999));
#28996=DIRECTION('',(-0.163114865717534,0.309436927624311,-0.936825665961591));
#28997=DIRECTION('center_axis',(-0.987377104088484,0.,-0.158387039627108));
#28998=DIRECTION('ref_axis',(-0.158387039627108,0.,0.987377104088484));
#28999=DIRECTION('',(0.,1.,0.));
#29000=DIRECTION('',(-0.158387039627108,0.,0.987377104088484));
#29001=DIRECTION('',(0.,1.,0.));
#29002=DIRECTION('center_axis',(-0.999774774701824,0.,0.0212226263670861));
#29003=DIRECTION('ref_axis',(0.0212226263670861,0.,0.999774774701824));
#29004=DIRECTION('',(0.,1.,0.));
#29005=DIRECTION('',(0.0208894774888421,0.176491388068498,0.984080494506368));
#29006=DIRECTION('center_axis',(-0.66064079706712,-0.707106781186548,0.252098665705553));
#29007=DIRECTION('ref_axis',(0.356521352096954,0.,0.934287175069293));
#29008=DIRECTION('',(-0.510131065430303,0.176491388068496,-0.841793968866848));
#29009=DIRECTION('',(-0.356521352096954,0.,-0.934287175069293));
#29010=DIRECTION('',(-0.673158076003201,0.706639907076676,0.217986803358222));
#29011=DIRECTION('',(-0.659781939307015,0.38671429502474,-0.644313469196317));
#29012=DIRECTION('',(-0.60967445042707,0.309436927624314,-0.729757392781241));
#29013=DIRECTION('center_axis',(-0.934287175069293,0.,0.356521352096954));
#29014=DIRECTION('ref_axis',(0.356521352096954,0.,0.934287175069293));
#29015=DIRECTION('',(0.,1.,0.));
#29016=DIRECTION('',(0.356521352096954,0.,0.934287175069293));
#29017=DIRECTION('',(0.,1.,0.));
#29018=DIRECTION('center_axis',(-0.855219039771101,0.,0.518266720919832));
#29019=DIRECTION('ref_axis',(0.518266720919832,0.,0.855219039771102));
#29020=DIRECTION('',(0.,1.,0.));
#29021=DIRECTION('',(0.510131065430303,0.176491388068496,0.841793968866848));
#29022=DIRECTION('center_axis',(-0.446082380183749,-0.707106781186548,0.54864424729473));
#29023=DIRECTION('ref_axis',(0.775900135442186,0.,0.63085575199153));
#29024=DIRECTION('',(-0.862683446355689,0.176491388068498,-0.473949429076063));
#29025=DIRECTION('',(-0.775900135442185,0.,-0.63085575199153));
#29026=DIRECTION('',(-0.473978592902316,0.706639907076676,0.525361147399584));
#29027=DIRECTION('',(-0.893544654996196,0.386714295024742,-0.228100862670982));
#29028=DIRECTION('',(-0.89287225849878,0.30943692762431,-0.327151215534523));
#29029=DIRECTION('center_axis',(-0.63085575199153,0.,0.775900135442186));
#29030=DIRECTION('ref_axis',(0.775900135442185,0.,0.63085575199153));
#29031=DIRECTION('',(0.,1.,0.));
#29032=DIRECTION('',(0.775900135442185,0.,0.63085575199153));
#29033=DIRECTION('',(0.,1.,0.));
#29034=DIRECTION('center_axis',(-0.481508053781989,0.,0.876441666138187));
#29035=DIRECTION('ref_axis',(0.876441666138187,0.,0.481508053781989));
#29036=DIRECTION('',(0.,1.,0.));
#29037=DIRECTION('',(0.862683446355689,0.176491388068498,0.473949429076063));
#29038=DIRECTION('center_axis',(-0.11199654977239,-0.707106781186549,0.698181045889302));
#29039=DIRECTION('ref_axis',(0.987377104088484,0.,0.158387039627108));
#29040=DIRECTION('',(-0.984080494506367,0.176491388068501,0.0208894774888451));
#29041=DIRECTION('',(-0.987377104088484,0.,-0.158387039627108));
#29042=DIRECTION('',(-0.147796928603616,0.706639907076675,0.69196539626054));
#29043=DIRECTION('',(-0.887882801977998,0.386714295024742,0.249231185799882));
#29044=DIRECTION('',(-0.936825665961591,0.309436927624309,0.163114865717533));
#29045=DIRECTION('center_axis',(-0.158387039627108,0.,0.987377104088484));
#29046=DIRECTION('ref_axis',(0.987377104088484,0.,0.158387039627108));
#29047=DIRECTION('',(0.,1.,0.));
#29048=DIRECTION('',(0.987377104088484,0.,0.158387039627108));
#29049=DIRECTION('',(0.,1.,0.));
#29050=DIRECTION('center_axis',(0.0212226263670891,0.,0.999774774701824));
#29051=DIRECTION('ref_axis',(0.999774774701824,0.,-0.0212226263670891));
#29052=DIRECTION('',(0.,1.,0.));
#29053=DIRECTION('',(0.984080494506367,0.176491388068501,-0.0208894774888451));
#29054=DIRECTION('center_axis',(0.252098665705552,-0.707106781186548,0.66064079706712));
#29055=DIRECTION('ref_axis',(0.934287175069293,0.,-0.356521352096954));
#29056=DIRECTION('',(-0.841793968866845,0.1764913880685,0.510131065430306));
#29057=DIRECTION('',(-0.934287175069293,0.,0.356521352096954));
#29058=DIRECTION('',(0.217986803358223,0.706639907076676,0.673158076003201));
#29059=DIRECTION('',(-0.644313469196316,0.386714295024741,0.659781939307015));
#29060=DIRECTION('',(-0.729757392781242,0.309436927624314,0.609674450427069));
#29061=DIRECTION('center_axis',(0.356521352096954,0.,0.934287175069293));
#29062=DIRECTION('ref_axis',(0.934287175069293,0.,-0.356521352096954));
#29063=DIRECTION('',(0.,1.,0.));
#29064=DIRECTION('',(0.934287175069293,0.,-0.356521352096954));
#29065=DIRECTION('',(0.,1.,0.));
#29066=DIRECTION('center_axis',(0.518266720919835,0.,0.855219039771099));
#29067=DIRECTION('ref_axis',(0.855219039771099,0.,-0.518266720919835));
#29068=DIRECTION('',(0.,1.,0.));
#29069=DIRECTION('',(0.841793968866845,0.1764913880685,-0.510131065430306));
#29070=DIRECTION('center_axis',(0.548644247294729,-0.707106781186549,0.446082380183749));
#29071=DIRECTION('ref_axis',(0.63085575199153,0.,-0.775900135442185));
#29072=DIRECTION('',(-0.473949429076064,0.176491388068498,0.862683446355688));
#29073=DIRECTION('',(-0.63085575199153,0.,0.775900135442185));
#29074=DIRECTION('',(0.525361147399584,0.706639907076675,0.473978592902317));
#29075=DIRECTION('',(-0.228100862670987,0.386714295024739,0.893544654996196));
#29076=DIRECTION('',(-0.327151215534519,0.309436927624314,0.89287225849878));
#29077=DIRECTION('center_axis',(0.775900135442185,0.,0.630855751991531));
#29078=DIRECTION('ref_axis',(0.63085575199153,0.,-0.775900135442185));
#29079=DIRECTION('',(0.,1.,0.));
#29080=DIRECTION('',(0.63085575199153,0.,-0.775900135442185));
#29081=DIRECTION('',(0.,1.,0.));
#29082=DIRECTION('center_axis',(0.876441666138186,0.,0.481508053781991));
#29083=DIRECTION('ref_axis',(0.481508053781991,0.,-0.876441666138186));
#29084=DIRECTION('',(0.,1.,0.));
#29085=DIRECTION('',(0.473949429076064,0.176491388068498,-0.862683446355688));
#29086=DIRECTION('center_axis',(0.698181045889302,-0.707106781186549,0.11199654977239));
#29087=DIRECTION('ref_axis',(0.158387039627108,0.,-0.987377104088484));
#29088=DIRECTION('',(0.0208894774888416,0.176491388068498,0.984080494506368));
#29089=DIRECTION('',(-0.158387039627108,0.,0.987377104088484));
#29090=DIRECTION('',(0.69196539626054,0.706639907076675,0.147796928603616));
#29091=DIRECTION('',(0.249231185799881,0.386714295024741,0.887882801977999));
#29092=DIRECTION('',(0.163114865717534,0.309436927624311,0.936825665961591));
#29093=DIRECTION('center_axis',(0.987377104088484,0.,0.158387039627108));
#29094=DIRECTION('ref_axis',(0.158387039627108,0.,-0.987377104088484));
#29095=DIRECTION('',(0.,1.,0.));
#29096=DIRECTION('',(0.158387039627108,0.,-0.987377104088484));
#29097=DIRECTION('',(0.,1.,0.));
#29098=DIRECTION('center_axis',(0.999774774701824,0.,-0.0212226263670855));
#29099=DIRECTION('ref_axis',(-0.0212226263670855,0.,-0.999774774701824));
#29100=DIRECTION('',(0.,1.,0.));
#29101=DIRECTION('',(-0.0208894774888416,0.176491388068498,-0.984080494506368));
#29102=DIRECTION('center_axis',(-0.698181045889302,0.707106781186549,0.111996549772391));
#29103=DIRECTION('ref_axis',(0.158387039627108,0.,0.987377104088484));
#29104=DIRECTION('',(-0.0208894774888421,-0.176491388068498,0.984080494506368));
#29105=DIRECTION('',(0.158387039627108,0.,0.987377104088484));
#29106=DIRECTION('',(-0.691965396260539,-0.706639907076675,0.147796928603617));
#29107=DIRECTION('',(-0.158387039627108,0.,-0.987377104088484));
#29108=DIRECTION('center_axis',(0.,1.,0.));
#29109=DIRECTION('ref_axis',(0.,0.,1.));
#29110=DIRECTION('',(-0.977941578718451,0.,0.20887859778748));
#29111=DIRECTION('',(-0.951361549480978,0.,0.308076617368395));
#29112=DIRECTION('',(0.356521352096954,0.,0.934287175069293));
#29113=DIRECTION('',(-0.715443769451104,0.,-0.69867031764173));
#29114=DIRECTION('',(-0.771525643922909,0.,-0.636198224431145));
#29115=DIRECTION('',(-0.816588132859797,0.,-0.577220773424303));
#29116=DIRECTION('',(-0.85383585346242,0.,-0.520542347309132));
#29117=DIRECTION('',(-0.885030574305658,0.,-0.465532901677419));
#29118=DIRECTION('',(-0.911263560158432,0.,-0.411823656347446));
#29119=DIRECTION('',(-0.876920914189556,0.,0.480634695228043));
#29120=DIRECTION('',(-0.869705019525388,0.,0.493571858002809));
#29121=DIRECTION('',(-0.862298277386214,0.,0.506400711706418));
#29122=DIRECTION('',(-0.854702313102447,0.,0.51911844118402));
#29123=DIRECTION('',(-0.0989820318029304,0.,0.995089220813975));
#29124=DIRECTION('',(-0.0393519680027076,0.,0.99922541131334));
#29125=DIRECTION('',(0.0238849697840824,0.,0.999714713414989));
#29126=DIRECTION('',(0.0915937869476479,0.,0.995796454197638));
#29127=DIRECTION('',(0.165201002238474,0.,0.986259919523958));
#29128=DIRECTION('',(-0.630855751991531,0.,-0.775900135442185));
#29129=DIRECTION('',(-0.742482951693498,0.,0.669864961350055));
#29130=DIRECTION('',(-0.669864961350053,0.,0.742482951693499));
#29131=DIRECTION('',(0.775900135442185,0.,0.630855751991531));
#29132=DIRECTION('',(-0.968927638144812,0.,-0.247344359222354));
#29133=DIRECTION('',(-0.986259919523961,0.,-0.165201002238458));
#29134=DIRECTION('',(-0.995796454197637,0.,-0.091593786947663));
#29135=DIRECTION('',(-0.99971471341499,0.,-0.023884969784058));
#29136=DIRECTION('',(-0.999225411313341,0.,0.0393519680026942));
#29137=DIRECTION('',(-0.995089220813975,0.,0.0989820318029307));
#29138=DIRECTION('',(-0.519118441184019,0.,0.854702313102448));
#29139=DIRECTION('',(-0.506400711706419,0.,0.862298277386214));
#29140=DIRECTION('',(-0.493571858002814,0.,0.869705019525385));
#29141=DIRECTION('',(-0.48063469522803,0.,0.876920914189563));
#29142=DIRECTION('',(0.411823656347447,0.,0.911263560158432));
#29143=DIRECTION('',(0.465532901677422,0.,0.885030574305656));
#29144=DIRECTION('',(0.520542347309115,0.,0.85383585346243));
#29145=DIRECTION('',(0.577220773424313,0.,0.81658813285979));
#29146=DIRECTION('',(0.636198224431135,0.,0.771525643922917));
#29147=DIRECTION('',(-0.934287175069293,0.,-0.356521352096954));
#29148=DIRECTION('',(-0.308076617368396,0.,0.951361549480978));
#29149=DIRECTION('',(-0.208878597787478,0.,0.977941578718451));
#29150=DIRECTION('',(0.987377104088484,0.,0.158387039627108));
#29151=DIRECTION('',(-0.962788128673439,0.,0.270257320503067));
#29152=DIRECTION('',(-0.936726646161376,0.,0.350061695092823));
#29153=DIRECTION('',(-0.908181919807451,0.,0.418575680773326));
#29154=DIRECTION('',(-0.87772082324649,0.,0.479172366105876));
#29155=DIRECTION('',(-0.845678606302961,0.,0.533692509635915));
#29156=DIRECTION('',(-0.812281528355498,0.,0.583265564466527));
#29157=DIRECTION('',(-0.0222186010871084,0.,0.99975313641205));
#29158=DIRECTION('',(-0.00740674213917776,0.,0.999972569709231));
#29159=DIRECTION('',(0.00740674213917776,0.,0.999972569709231));
#29160=DIRECTION('',(0.0222186010871084,0.,0.99975313641205));
#29161=DIRECTION('',(0.8122815283555,0.,0.583265564466524));
#29162=DIRECTION('',(0.84567860630296,0.,0.533692509635917));
#29163=DIRECTION('',(0.87772082324649,0.,0.479172366105876));
#29164=DIRECTION('',(0.908181919807451,0.,0.418575680773325));
#29165=DIRECTION('',(0.936726646161376,0.,0.350061695092823));
#29166=DIRECTION('',(-0.987377104088484,0.,0.158387039627109));
#29167=DIRECTION('',(0.20887859778748,0.,0.977941578718451));
#29168=DIRECTION('',(0.308076617368396,0.,0.951361549480978));
#29169=DIRECTION('',(0.934287175069293,0.,-0.356521352096954));
#29170=DIRECTION('',(-0.698670317641747,0.,0.715443769451087));
#29171=DIRECTION('',(-0.636198224431136,0.,0.771525643922916));
#29172=DIRECTION('',(-0.577220773424311,0.,0.816588132859791));
#29173=DIRECTION('',(-0.520542347309115,0.,0.85383585346243));
#29174=DIRECTION('',(-0.465532901677425,0.,0.885030574305655));
#29175=DIRECTION('',(-0.41182365634745,0.,0.91126356015843));
#29176=DIRECTION('',(0.480634695228042,0.,0.876920914189556));
#29177=DIRECTION('',(0.493571858002802,0.,0.869705019525391));
#29178=DIRECTION('',(0.506400711706431,0.,0.862298277386207));
#29179=DIRECTION('',(0.519118441184006,0.,0.854702313102456));
#29180=DIRECTION('',(0.995089220813975,0.,0.0989820318029304));
#29181=DIRECTION('',(0.999225411313341,0.,0.0393519680026977));
#29182=DIRECTION('',(0.99971471341499,0.,-0.0238849697840613));
#29183=DIRECTION('',(0.995796454197637,0.,-0.0915937869476627));
#29184=DIRECTION('',(0.98625991952396,0.,-0.165201002238459));
#29185=DIRECTION('',(-0.775900135442185,0.,0.63085575199153));
#29186=DIRECTION('',(0.669864961350055,0.,0.742482951693498));
#29187=DIRECTION('',(0.742482951693498,0.,0.669864961350055));
#29188=DIRECTION('',(0.63085575199153,0.,-0.775900135442185));
#29189=DIRECTION('',(-0.247344359222349,0.,0.968927638144813));
#29190=DIRECTION('',(-0.165201002238462,0.,0.98625991952396));
#29191=DIRECTION('',(-0.0915937869476591,0.,0.995796454197637));
#29192=DIRECTION('',(-0.0238849697840614,0.,0.99971471341499));
#29193=DIRECTION('',(0.0393519680026975,0.,0.999225411313341));
#29194=DIRECTION('',(0.0989820318029307,0.,0.995089220813975));
#29195=DIRECTION('',(0.85470231310245,0.,0.519118441184015));
#29196=DIRECTION('',(0.86229827738621,0.,0.506400711706427));
#29197=DIRECTION('',(0.86970501952539,0.,0.493571858002805));
#29198=DIRECTION('',(0.876920914189557,0.,0.48063469522804));
#29199=DIRECTION('',(0.911263560158429,0.,-0.411823656347453));
#29200=DIRECTION('',(0.885030574305657,0.,-0.46553290167742));
#29201=DIRECTION('',(0.853835853462428,0.,-0.520542347309119));
#29202=DIRECTION('',(0.816588132859795,0.,-0.577220773424306));
#29203=DIRECTION('',(0.771525643922911,0.,-0.636198224431142));
#29204=DIRECTION('',(-0.356521352096954,0.,0.934287175069293));
#29205=DIRECTION('',(0.951361549480978,0.,0.308076617368397));
#29206=DIRECTION('',(0.977941578718451,0.,0.208878597787479));
#29207=DIRECTION('',(0.158387039627108,0.,-0.987377104088484));
#29208=DIRECTION('',(0.270257320503068,0.,0.962788128673439));
#29209=DIRECTION('',(0.350061695092817,0.,0.936726646161378));
#29210=DIRECTION('',(0.418575680773335,0.,0.908181919807446));
#29211=DIRECTION('',(0.479172366105872,0.,0.877720823246493));
#29212=DIRECTION('',(0.533692509635919,0.,0.845678606302959));
#29213=DIRECTION('',(0.583265564466523,0.,0.812281528355501));
#29214=DIRECTION('',(0.99975313641205,0.,0.0222186010871085));
#29215=DIRECTION('',(0.999972569709231,0.,0.00740674213917776));
#29216=DIRECTION('',(0.999972569709231,0.,-0.00740674213917776));
#29217=DIRECTION('',(0.99975313641205,0.,-0.0222186010871084));
#29218=DIRECTION('',(0.583265564466523,0.,-0.812281528355501));
#29219=DIRECTION('',(0.533692509635919,0.,-0.845678606302959));
#29220=DIRECTION('',(0.479172366105872,0.,-0.877720823246493));
#29221=DIRECTION('',(0.418575680773335,0.,-0.908181919807446));
#29222=DIRECTION('',(0.350061695092817,0.,-0.936726646161378));
#29223=DIRECTION('',(0.158387039627108,0.,0.987377104088484));
#29224=DIRECTION('',(0.977941578718451,0.,-0.208878597787478));
#29225=DIRECTION('',(0.951361549480978,0.,-0.308076617368396));
#29226=DIRECTION('',(-0.356521352096954,0.,-0.934287175069293));
#29227=DIRECTION('',(0.715443769451087,0.,0.698670317641747));
#29228=DIRECTION('',(0.771525643922913,0.,0.63619822443114));
#29229=DIRECTION('',(0.816588132859796,0.,0.577220773424304));
#29230=DIRECTION('',(0.853835853462428,0.,0.520542347309119));
#29231=DIRECTION('',(0.885030574305657,0.,0.465532901677421));
#29232=DIRECTION('',(0.911263560158431,0.,0.411823656347449));
#29233=DIRECTION('',(0.876920914189562,0.,-0.480634695228032));
#29234=DIRECTION('',(0.869705019525386,0.,-0.493571858002812));
#29235=DIRECTION('',(0.862298277386212,0.,-0.506400711706423));
#29236=DIRECTION('',(0.85470231310245,0.,-0.519118441184015));
#29237=DIRECTION('',(0.0989820318029246,0.,-0.995089220813975));
#29238=DIRECTION('',(0.0393519680027008,0.,-0.999225411313341));
#29239=DIRECTION('',(-0.0238849697840649,0.,-0.999714713414989));
#29240=DIRECTION('',(-0.0915937869476482,0.,-0.995796454197638));
#29241=DIRECTION('',(-0.165201002238466,0.,-0.986259919523959));
#29242=DIRECTION('',(0.63085575199153,0.,0.775900135442185));
#29243=DIRECTION('',(0.742482951693498,0.,-0.669864961350055));
#29244=DIRECTION('',(0.669864961350055,0.,-0.742482951693498));
#29245=DIRECTION('',(-0.775900135442185,0.,-0.63085575199153));
#29246=DIRECTION('',(0.968927638144813,0.,0.247344359222349));
#29247=DIRECTION('',(0.986259919523959,0.,0.165201002238466));
#29248=DIRECTION('',(0.995796454197638,0.,0.0915937869476553));
#29249=DIRECTION('',(0.999714713414989,0.,0.0238849697840649));
#29250=DIRECTION('',(0.99922541131334,0.,-0.039351968002701));
#29251=DIRECTION('',(0.995089220813975,0.,-0.0989820318029272));
#29252=DIRECTION('',(0.519118441184011,0.,-0.854702313102452));
#29253=DIRECTION('',(0.506400711706425,0.,-0.862298277386211));
#29254=DIRECTION('',(0.493571858002802,0.,-0.869705019525391));
#29255=DIRECTION('',(0.480634695228039,0.,-0.876920914189558));
#29256=DIRECTION('',(-0.411823656347455,0.,-0.911263560158428));
#29257=DIRECTION('',(-0.465532901677421,0.,-0.885030574305657));
#29258=DIRECTION('',(-0.520542347309117,0.,-0.853835853462429));
#29259=DIRECTION('',(-0.577220773424305,0.,-0.816588132859795));
#29260=DIRECTION('',(-0.636198224431141,0.,-0.771525643922912));
#29261=DIRECTION('',(0.934287175069293,0.,0.356521352096954));
#29262=DIRECTION('',(0.308076617368396,0.,-0.951361549480978));
#29263=DIRECTION('',(0.208878597787478,0.,-0.977941578718451));
#29264=DIRECTION('',(-0.987377104088484,0.,-0.158387039627108));
#29265=DIRECTION('',(0.962788128673439,0.,-0.270257320503068));
#29266=DIRECTION('',(0.936726646161378,0.,-0.350061695092817));
#29267=DIRECTION('',(0.908181919807447,0.,-0.418575680773333));
#29268=DIRECTION('',(0.877720823246493,0.,-0.479172366105871));
#29269=DIRECTION('',(0.845678606302959,0.,-0.533692509635919));
#29270=DIRECTION('',(0.812281528355501,0.,-0.583265564466523));
#29271=DIRECTION('',(0.0222186010871084,0.,-0.99975313641205));
#29272=DIRECTION('',(0.00740674213917775,0.,-0.999972569709231));
#29273=DIRECTION('',(-0.00740674213917775,0.,-0.999972569709231));
#29274=DIRECTION('',(-0.0222186010871084,0.,-0.99975313641205));
#29275=DIRECTION('',(-0.812281528355501,0.,-0.583265564466523));
#29276=DIRECTION('',(-0.845678606302959,0.,-0.533692509635919));
#29277=DIRECTION('',(-0.877720823246493,0.,-0.479172366105871));
#29278=DIRECTION('',(-0.908181919807447,0.,-0.418575680773333));
#29279=DIRECTION('',(-0.936726646161378,0.,-0.350061695092817));
#29280=DIRECTION('',(0.987377104088484,0.,-0.158387039627108));
#29281=DIRECTION('',(-0.208878597787478,0.,-0.977941578718451));
#29282=DIRECTION('',(-0.308076617368396,0.,-0.951361549480978));
#29283=DIRECTION('',(-0.934287175069293,0.,0.356521352096954));
#29284=DIRECTION('',(0.698670317641746,0.,-0.715443769451088));
#29285=DIRECTION('',(0.636198224431141,0.,-0.771525643922912));
#29286=DIRECTION('',(0.577220773424305,0.,-0.816588132859795));
#29287=DIRECTION('',(0.520542347309117,0.,-0.853835853462429));
#29288=DIRECTION('',(0.465532901677421,0.,-0.885030574305657));
#29289=DIRECTION('',(0.411823656347455,0.,-0.911263560158428));
#29290=DIRECTION('',(-0.480634695228039,0.,-0.876920914189558));
#29291=DIRECTION('',(-0.493571858002802,0.,-0.869705019525391));
#29292=DIRECTION('',(-0.506400711706425,0.,-0.862298277386211));
#29293=DIRECTION('',(-0.519118441184011,0.,-0.854702313102452));
#29294=DIRECTION('',(-0.995089220813975,0.,-0.0989820318029272));
#29295=DIRECTION('',(-0.99922541131334,0.,-0.039351968002701));
#29296=DIRECTION('',(-0.999714713414989,0.,0.0238849697840649));
#29297=DIRECTION('',(-0.995796454197638,0.,0.0915937869476553));
#29298=DIRECTION('',(-0.986259919523959,0.,0.165201002238466));
#29299=DIRECTION('',(0.775900135442185,0.,-0.63085575199153));
#29300=DIRECTION('',(-0.669864961350055,0.,-0.742482951693498));
#29301=DIRECTION('',(-0.742482951693498,0.,-0.669864961350055));
#29302=DIRECTION('',(-0.63085575199153,0.,0.775900135442185));
#29303=DIRECTION('',(0.247344359222354,0.,-0.968927638144812));
#29304=DIRECTION('',(0.165201002238466,0.,-0.986259919523959));
#29305=DIRECTION('',(0.0915937869476482,0.,-0.995796454197638));
#29306=DIRECTION('',(0.0238849697840649,0.,-0.999714713414989));
#29307=DIRECTION('',(-0.0393519680027008,0.,-0.999225411313341));
#29308=DIRECTION('',(-0.0989820318029246,0.,-0.995089220813975));
#29309=DIRECTION('',(-0.85470231310245,0.,-0.519118441184015));
#29310=DIRECTION('',(-0.862298277386212,0.,-0.506400711706423));
#29311=DIRECTION('',(-0.869705019525386,0.,-0.493571858002812));
#29312=DIRECTION('',(-0.876920914189562,0.,-0.480634695228032));
#29313=DIRECTION('',(-0.911263560158431,0.,0.411823656347449));
#29314=DIRECTION('',(-0.885030574305657,0.,0.465532901677421));
#29315=DIRECTION('',(-0.853835853462428,0.,0.520542347309119));
#29316=DIRECTION('',(-0.816588132859796,0.,0.577220773424304));
#29317=DIRECTION('',(-0.771525643922913,0.,0.63619822443114));
#29318=DIRECTION('',(0.356521352096954,0.,-0.934287175069293));
#29319=DIRECTION('',(-0.951361549480978,0.,-0.308076617368396));
#29320=DIRECTION('',(-0.977941578718451,0.,-0.208878597787478));
#29321=DIRECTION('',(-0.158387039627108,0.,0.987377104088484));
#29322=DIRECTION('',(-0.270257320503068,0.,-0.962788128673439));
#29323=DIRECTION('',(-0.350061695092817,0.,-0.936726646161378));
#29324=DIRECTION('',(-0.418575680773335,0.,-0.908181919807446));
#29325=DIRECTION('',(-0.479172366105872,0.,-0.877720823246493));
#29326=DIRECTION('',(-0.533692509635919,0.,-0.845678606302959));
#29327=DIRECTION('',(-0.583265564466523,0.,-0.812281528355501));
#29328=DIRECTION('',(-0.99975313641205,0.,-0.0222186010871084));
#29329=DIRECTION('',(-0.999972569709231,0.,-0.00740674213917776));
#29330=DIRECTION('',(-0.999972569709231,0.,0.00740674213917776));
#29331=DIRECTION('',(-0.99975313641205,0.,0.0222186010871085));
#29332=DIRECTION('',(-0.583265564466523,0.,0.812281528355501));
#29333=DIRECTION('',(-0.533692509635919,0.,0.845678606302959));
#29334=DIRECTION('',(-0.479172366105872,0.,0.877720823246493));
#29335=DIRECTION('',(-0.418575680773335,0.,0.908181919807446));
#29336=DIRECTION('',(-0.350061695092817,0.,0.936726646161378));
#29337=DIRECTION('center_axis',(0.,1.,0.));
#29338=DIRECTION('ref_axis',(0.,0.,1.));
#29339=DIRECTION('center_axis',(0.698181045889302,0.707106781186549,0.11199654977239));
#29340=DIRECTION('ref_axis',(0.158387039627108,0.,-0.987377104088484));
#29341=DIRECTION('',(-0.249231185799881,0.386714295024741,-0.887882801977999));
#29342=DIRECTION('',(-0.69196539626054,0.706639907076675,-0.147796928603616));
#29343=DIRECTION('',(-0.163114865717534,0.309436927624311,-0.936825665961591));
#29344=DIRECTION('center_axis',(-0.660640797067119,0.707106781186548,-0.252098665705553));
#29345=DIRECTION('ref_axis',(-0.356521352096954,0.,0.934287175069293));
#29346=DIRECTION('',(-0.510131065430303,-0.176491388068496,0.841793968866848));
#29347=DIRECTION('',(-0.356521352096954,0.,0.934287175069293));
#29348=DIRECTION('',(-0.673158076003201,-0.706639907076675,-0.217986803358222));
#29349=DIRECTION('center_axis',(0.548644247294729,0.707106781186549,0.446082380183749));
#29350=DIRECTION('ref_axis',(0.63085575199153,0.,-0.775900135442185));
#29351=DIRECTION('',(0.228100862670987,0.386714295024739,-0.893544654996196));
#29352=DIRECTION('',(-0.525361147399584,0.706639907076675,-0.473978592902317));
#29353=DIRECTION('',(0.327151215534519,0.309436927624314,-0.89287225849878));
#29354=DIRECTION('center_axis',(-0.446082380183748,0.707106781186549,-0.548644247294729));
#29355=DIRECTION('ref_axis',(-0.775900135442186,0.,0.63085575199153));
#29356=DIRECTION('',(-0.862683446355689,-0.176491388068498,0.473949429076063));
#29357=DIRECTION('',(-0.775900135442185,0.,0.63085575199153));
#29358=DIRECTION('',(-0.473978592902317,-0.706639907076675,-0.525361147399585));
#29359=DIRECTION('center_axis',(0.252098665705552,0.707106781186548,0.66064079706712));
#29360=DIRECTION('ref_axis',(0.934287175069293,0.,-0.356521352096954));
#29361=DIRECTION('',(0.644313469196316,0.386714295024741,-0.659781939307015));
#29362=DIRECTION('',(-0.217986803358223,0.706639907076676,-0.673158076003201));
#29363=DIRECTION('',(0.729757392781242,0.309436927624314,-0.609674450427069));
#29364=DIRECTION('center_axis',(-0.11199654977239,0.707106781186549,-0.698181045889302));
#29365=DIRECTION('ref_axis',(-0.987377104088484,0.,0.158387039627108));
#29366=DIRECTION('',(-0.984080494506367,-0.176491388068501,-0.0208894774888451));
#29367=DIRECTION('',(-0.987377104088484,0.,0.158387039627108));
#29368=DIRECTION('',(-0.147796928603616,-0.706639907076675,-0.691965396260539));
#29369=DIRECTION('center_axis',(-0.11199654977239,0.707106781186549,0.698181045889302));
#29370=DIRECTION('ref_axis',(0.987377104088484,0.,0.158387039627108));
#29371=DIRECTION('',(0.887882801977998,0.386714295024742,-0.249231185799882));
#29372=DIRECTION('',(0.147796928603616,0.706639907076675,-0.69196539626054));
#29373=DIRECTION('',(0.936825665961591,0.309436927624309,-0.163114865717533));
#29374=DIRECTION('center_axis',(0.252098665705552,0.707106781186548,-0.660640797067119));
#29375=DIRECTION('ref_axis',(-0.934287175069293,0.,-0.356521352096954));
#29376=DIRECTION('',(-0.841793968866845,-0.1764913880685,-0.510131065430306));
#29377=DIRECTION('',(-0.934287175069293,0.,-0.356521352096954));
#29378=DIRECTION('',(0.217986803358223,-0.706639907076675,-0.673158076003201));
#29379=DIRECTION('center_axis',(-0.446082380183749,0.707106781186548,0.54864424729473));
#29380=DIRECTION('ref_axis',(0.775900135442186,0.,0.63085575199153));
#29381=DIRECTION('',(0.893544654996196,0.386714295024742,0.228100862670982));
#29382=DIRECTION('',(0.473978592902316,0.706639907076676,-0.525361147399584));
#29383=DIRECTION('',(0.89287225849878,0.30943692762431,0.327151215534523));
#29384=DIRECTION('center_axis',(0.548644247294728,0.70710678118655,-0.446082380183749));
#29385=DIRECTION('ref_axis',(-0.63085575199153,0.,-0.775900135442185));
#29386=DIRECTION('',(-0.473949429076065,-0.176491388068497,-0.862683446355688));
#29387=DIRECTION('',(-0.63085575199153,0.,-0.775900135442185));
#29388=DIRECTION('',(0.525361147399585,-0.706639907076674,-0.473978592902318));
#29389=DIRECTION('center_axis',(-0.66064079706712,0.707106781186548,0.252098665705553));
#29390=DIRECTION('ref_axis',(0.356521352096954,0.,0.934287175069293));
#29391=DIRECTION('',(0.659781939307015,0.38671429502474,0.644313469196317));
#29392=DIRECTION('',(0.673158076003201,0.706639907076676,-0.217986803358222));
#29393=DIRECTION('',(0.60967445042707,0.309436927624314,0.729757392781241));
#29394=DIRECTION('center_axis',(0.698181045889302,0.707106781186549,-0.11199654977239));
#29395=DIRECTION('ref_axis',(-0.158387039627108,0.,-0.987377104088484));
#29396=DIRECTION('',(0.0208894774888416,-0.176491388068498,-0.984080494506368));
#29397=DIRECTION('',(-0.158387039627108,0.,-0.987377104088484));
#29398=DIRECTION('',(0.691965396260539,-0.706639907076675,-0.147796928603616));
#29399=DIRECTION('center_axis',(-0.698181045889302,0.707106781186549,-0.111996549772391));
#29400=DIRECTION('ref_axis',(-0.158387039627108,0.,0.987377104088484));
#29401=DIRECTION('',(0.249231185799882,0.386714295024742,0.887882801977999));
#29402=DIRECTION('',(0.691965396260539,0.706639907076675,0.147796928603617));
#29403=DIRECTION('',(0.163114865717534,0.309436927624311,0.936825665961591));
#29404=DIRECTION('center_axis',(0.660640797067119,0.707106781186549,0.252098665705552));
#29405=DIRECTION('ref_axis',(0.356521352096954,0.,-0.934287175069293));
#29406=DIRECTION('',(0.510131065430304,-0.176491388068498,-0.841793968866847));
#29407=DIRECTION('',(0.356521352096954,0.,-0.934287175069293));
#29408=DIRECTION('',(0.673158076003201,-0.706639907076675,0.217986803358224));
#29409=DIRECTION('center_axis',(-0.54864424729473,0.707106781186548,-0.446082380183749));
#29410=DIRECTION('ref_axis',(-0.63085575199153,0.,0.775900135442186));
#29411=DIRECTION('',(-0.228100862670983,0.386714295024742,0.893544654996196));
#29412=DIRECTION('',(0.525361147399584,0.706639907076676,0.473978592902316));
#29413=DIRECTION('',(-0.327151215534528,0.309436927624306,0.892872258498779));
#29414=DIRECTION('center_axis',(0.446082380183749,0.70710678118655,0.548644247294728));
#29415=DIRECTION('ref_axis',(0.775900135442185,0.,-0.63085575199153));
#29416=DIRECTION('',(0.862683446355692,-0.176491388068509,-0.473949429076052));
#29417=DIRECTION('',(0.775900135442185,0.,-0.63085575199153));
#29418=DIRECTION('',(0.473978592902318,-0.706639907076674,0.525361147399585));
#29419=DIRECTION('center_axis',(-0.252098665705553,0.707106781186548,-0.66064079706712));
#29420=DIRECTION('ref_axis',(-0.934287175069293,0.,0.356521352096954));
#29421=DIRECTION('',(-0.644313469196317,0.38671429502474,0.659781939307015));
#29422=DIRECTION('',(0.217986803358222,0.706639907076676,0.6731580760032));
#29423=DIRECTION('',(-0.729757392781247,0.309436927624309,0.609674450427066));
#29424=DIRECTION('center_axis',(0.111996549772391,0.707106781186548,0.698181045889302));
#29425=DIRECTION('ref_axis',(0.987377104088484,0.,-0.158387039627109));
#29426=DIRECTION('',(0.984080494506366,-0.176491388068509,0.0208894774888531));
#29427=DIRECTION('',(0.987377104088484,0.,-0.158387039627109));
#29428=DIRECTION('',(0.147796928603617,-0.706639907076676,0.691965396260539));
#29429=DIRECTION('center_axis',(0.11199654977239,0.707106781186549,-0.698181045889302));
#29430=DIRECTION('ref_axis',(-0.987377104088484,0.,-0.158387039627108));
#29431=DIRECTION('',(-0.887882801977999,0.386714295024741,0.249231185799881));
#29432=DIRECTION('',(-0.147796928603616,0.706639907076675,0.691965396260539));
#29433=DIRECTION('',(-0.936825665961593,0.309436927624307,0.16311486571753));
#29434=DIRECTION('center_axis',(-0.252098665705552,0.707106781186548,0.660640797067119));
#29435=DIRECTION('ref_axis',(0.934287175069293,0.,0.356521352096954));
#29436=DIRECTION('',(0.841793968866839,-0.176491388068509,0.510131065430313));
#29437=DIRECTION('',(0.934287175069293,0.,0.356521352096954));
#29438=DIRECTION('',(-0.217986803358223,-0.706639907076675,0.673158076003201));
#29439=DIRECTION('center_axis',(0.446082380183749,0.70710678118655,-0.548644247294728));
#29440=DIRECTION('ref_axis',(-0.775900135442185,0.,-0.630855751991531));
#29441=DIRECTION('',(-0.893544654996196,0.386714295024738,-0.228100862670987));
#29442=DIRECTION('',(-0.473978592902316,0.706639907076674,0.525361147399586));
#29443=DIRECTION('',(-0.892872258498779,0.309436927624308,-0.327151215534526));
#29444=DIRECTION('center_axis',(-0.548644247294728,0.70710678118655,0.446082380183749));
#29445=DIRECTION('ref_axis',(0.630855751991531,0.,0.775900135442185));
#29446=DIRECTION('',(0.473949429076065,-0.176491388068498,0.862683446355688));
#29447=DIRECTION('',(0.630855751991531,0.,0.775900135442185));
#29448=DIRECTION('',(-0.525361147399585,-0.706639907076674,0.473978592902317));
#29449=DIRECTION('center_axis',(0.660640797067119,0.707106781186549,-0.252098665705553));
#29450=DIRECTION('ref_axis',(-0.356521352096954,0.,-0.934287175069293));
#29451=DIRECTION('',(-0.659781939307025,0.386714295024756,-0.644313469196296));
#29452=DIRECTION('',(-0.673158076003201,0.706639907076675,0.217986803358222));
#29453=DIRECTION('',(-0.609674450427067,0.309436927624308,-0.729757392781247));
#29454=DIRECTION('center_axis',(0.,-1.,0.));
#29455=DIRECTION('ref_axis',(-1.,0.,0.));
#29456=DIRECTION('center_axis',(0.,-1.,0.));
#29457=DIRECTION('ref_axis',(0.,0.,1.));
#29458=DIRECTION('',(0.,0.,-1.));
#29459=DIRECTION('',(-1.,0.,0.));
#29460=DIRECTION('',(0.,0.,-1.));
#29461=DIRECTION('center_axis',(-1.,0.,0.));
#29462=DIRECTION('ref_axis',(0.,1.,0.));
#29463=DIRECTION('',(0.,1.,0.));
#29464=DIRECTION('',(0.,1.,0.));
#29465=DIRECTION('',(0.,0.,-1.));
#29466=DIRECTION('center_axis',(1.,0.,0.));
#29467=DIRECTION('ref_axis',(0.,-1.,0.));
#29468=DIRECTION('',(0.,-1.,0.));
#29469=DIRECTION('',(0.,0.,-1.));
#29470=DIRECTION('',(0.,-1.,0.));
#29471=DIRECTION('center_axis',(0.,1.,0.));
#29472=DIRECTION('ref_axis',(1.,0.,0.));
#29473=DIRECTION('center_axis',(0.,1.,0.));
#29474=DIRECTION('ref_axis',(0.,0.,1.));
#29475=DIRECTION('',(1.,0.,0.));
#29476=DIRECTION('center_axis',(0.,0.,-1.));
#29477=DIRECTION('ref_axis',(-1.,0.,0.));
#29478=DIRECTION('center_axis',(-0.20887859778748,0.,-0.977941578718451));
#29479=DIRECTION('ref_axis',(-0.977941578718451,0.,0.20887859778748));
#29480=DIRECTION('',(0.,1.,0.));
#29481=DIRECTION('',(0.,1.,0.));
#29482=DIRECTION('center_axis',(-0.987377104088484,0.,0.158387039627108));
#29483=DIRECTION('ref_axis',(0.158387039627108,0.,0.987377104088484));
#29484=DIRECTION('',(0.,1.,0.));
#29485=DIRECTION('center_axis',(-0.999774774701824,0.,-0.0212226263670861));
#29486=DIRECTION('ref_axis',(-0.0212226263670861,0.,0.999774774701824));
#29487=DIRECTION('center_axis',(-0.936726646161378,0.,-0.350061695092817));
#29488=DIRECTION('ref_axis',(-0.350061695092817,0.,0.936726646161378));
#29489=DIRECTION('',(0.,1.,0.));
#29490=DIRECTION('center_axis',(-0.908181919807446,0.,-0.418575680773336));
#29491=DIRECTION('ref_axis',(-0.418575680773336,0.,0.908181919807446));
#29492=DIRECTION('',(0.,1.,0.));
#29493=DIRECTION('center_axis',(-0.877720823246492,0.,-0.479172366105872));
#29494=DIRECTION('ref_axis',(-0.479172366105872,0.,0.877720823246493));
#29495=DIRECTION('',(0.,1.,0.));
#29496=DIRECTION('center_axis',(-0.845678606302959,0.,-0.533692509635919));
#29497=DIRECTION('ref_axis',(-0.533692509635919,0.,0.845678606302959));
#29498=DIRECTION('',(0.,1.,0.));
#29499=DIRECTION('center_axis',(-0.812281528355501,0.,-0.583265564466523));
#29500=DIRECTION('ref_axis',(-0.583265564466523,0.,0.812281528355501));
#29501=DIRECTION('',(0.,1.,0.));
#29502=DIRECTION('center_axis',(-0.0222186010871085,0.,-0.999753136412051));
#29503=DIRECTION('ref_axis',(-0.99975313641205,0.,0.0222186010871085));
#29504=DIRECTION('',(0.,1.,0.));
#29505=DIRECTION('center_axis',(-0.00740674213917776,0.,-0.999972569709231));
#29506=DIRECTION('ref_axis',(-0.999972569709231,0.,0.00740674213917776));
#29507=DIRECTION('',(0.,1.,0.));
#29508=DIRECTION('center_axis',(0.00740674213917776,0.,-0.999972569709231));
#29509=DIRECTION('ref_axis',(-0.999972569709231,0.,-0.00740674213917776));
#29510=DIRECTION('',(0.,1.,0.));
#29511=DIRECTION('center_axis',(0.0222186010871084,0.,-0.999753136412051));
#29512=DIRECTION('ref_axis',(-0.99975313641205,0.,-0.0222186010871084));
#29513=DIRECTION('',(0.,1.,0.));
#29514=DIRECTION('center_axis',(0.812281528355501,0.,-0.583265564466523));
#29515=DIRECTION('ref_axis',(-0.583265564466523,0.,-0.812281528355501));
#29516=DIRECTION('',(0.,1.,0.));
#29517=DIRECTION('center_axis',(0.845678606302959,0.,-0.533692509635919));
#29518=DIRECTION('ref_axis',(-0.533692509635919,0.,-0.845678606302959));
#29519=DIRECTION('',(0.,1.,0.));
#29520=DIRECTION('center_axis',(0.877720823246492,0.,-0.479172366105872));
#29521=DIRECTION('ref_axis',(-0.479172366105872,0.,-0.877720823246493));
#29522=DIRECTION('',(0.,1.,0.));
#29523=DIRECTION('center_axis',(0.908181919807446,0.,-0.418575680773335));
#29524=DIRECTION('ref_axis',(-0.418575680773335,0.,-0.908181919807446));
#29525=DIRECTION('',(0.,1.,0.));
#29526=DIRECTION('center_axis',(0.936726646161378,0.,-0.350061695092817));
#29527=DIRECTION('ref_axis',(-0.350061695092817,0.,-0.936726646161378));
#29528=DIRECTION('',(0.,1.,0.));
#29529=DIRECTION('center_axis',(0.962788128673439,0.,-0.270257320503068));
#29530=DIRECTION('ref_axis',(-0.270257320503068,0.,-0.962788128673439));
#29531=DIRECTION('',(0.,1.,0.));
#29532=DIRECTION('center_axis',(0.985178244547962,0.,-0.171533747319286));
#29533=DIRECTION('ref_axis',(-0.171533747319286,0.,-0.985178244547962));
#29534=DIRECTION('center_axis',(0.208878597787478,0.,-0.977941578718451));
#29535=DIRECTION('ref_axis',(-0.977941578718451,0.,-0.208878597787478));
#29536=DIRECTION('',(0.,1.,0.));
#29537=DIRECTION('center_axis',(0.308076617368396,0.,-0.951361549480978));
#29538=DIRECTION('ref_axis',(-0.951361549480978,0.,-0.308076617368396));
#29539=DIRECTION('',(0.,1.,0.));
#29540=DIRECTION('center_axis',(-0.934287175069293,0.,-0.356521352096954));
#29541=DIRECTION('ref_axis',(-0.356521352096954,0.,0.934287175069293));
#29542=DIRECTION('',(0.,1.,0.));
#29543=DIRECTION('center_axis',(-0.855219039771101,0.,-0.518266720919832));
#29544=DIRECTION('ref_axis',(-0.518266720919832,0.,0.855219039771102));
#29545=DIRECTION('center_axis',(-0.63619822443114,0.,-0.771525643922913));
#29546=DIRECTION('ref_axis',(-0.771525643922913,0.,0.63619822443114));
#29547=DIRECTION('',(0.,1.,0.));
#29548=DIRECTION('center_axis',(-0.577220773424304,0.,-0.816588132859796));
#29549=DIRECTION('ref_axis',(-0.816588132859796,0.,0.577220773424304));
#29550=DIRECTION('',(0.,1.,0.));
#29551=DIRECTION('center_axis',(-0.520542347309119,0.,-0.853835853462428));
#29552=DIRECTION('ref_axis',(-0.853835853462428,0.,0.520542347309119));
#29553=DIRECTION('',(0.,1.,0.));
#29554=DIRECTION('center_axis',(-0.465532901677421,0.,-0.885030574305657));
#29555=DIRECTION('ref_axis',(-0.885030574305657,0.,0.465532901677421));
#29556=DIRECTION('',(0.,1.,0.));
#29557=DIRECTION('center_axis',(-0.411823656347449,0.,-0.911263560158431));
#29558=DIRECTION('ref_axis',(-0.911263560158431,0.,0.411823656347449));
#29559=DIRECTION('',(0.,1.,0.));
#29560=DIRECTION('center_axis',(0.480634695228032,0.,-0.876920914189562));
#29561=DIRECTION('ref_axis',(-0.876920914189562,0.,-0.480634695228032));
#29562=DIRECTION('',(0.,1.,0.));
#29563=DIRECTION('center_axis',(0.493571858002813,0.,-0.869705019525386));
#29564=DIRECTION('ref_axis',(-0.869705019525386,0.,-0.493571858002812));
#29565=DIRECTION('',(0.,1.,0.));
#29566=DIRECTION('center_axis',(0.506400711706423,0.,-0.862298277386212));
#29567=DIRECTION('ref_axis',(-0.862298277386212,0.,-0.506400711706423));
#29568=DIRECTION('',(0.,1.,0.));
#29569=DIRECTION('center_axis',(0.519118441184015,0.,-0.85470231310245));
#29570=DIRECTION('ref_axis',(-0.85470231310245,0.,-0.519118441184015));
#29571=DIRECTION('',(0.,1.,0.));
#29572=DIRECTION('center_axis',(0.995089220813976,0.,-0.0989820318029246));
#29573=DIRECTION('ref_axis',(-0.0989820318029246,0.,-0.995089220813976));
#29574=DIRECTION('',(0.,1.,0.));
#29575=DIRECTION('center_axis',(0.999225411313341,0.,-0.0393519680027008));
#29576=DIRECTION('ref_axis',(-0.0393519680027008,0.,-0.999225411313341));
#29577=DIRECTION('',(0.,1.,0.));
#29578=DIRECTION('center_axis',(0.999714713414989,0.,0.0238849697840649));
#29579=DIRECTION('ref_axis',(0.0238849697840649,0.,-0.99971471341499));
#29580=DIRECTION('',(0.,1.,0.));
#29581=DIRECTION('center_axis',(0.995796454197638,0.,0.0915937869476482));
#29582=DIRECTION('ref_axis',(0.0915937869476482,0.,-0.995796454197638));
#29583=DIRECTION('',(0.,1.,0.));
#29584=DIRECTION('center_axis',(0.986259919523959,0.,0.165201002238466));
#29585=DIRECTION('ref_axis',(0.165201002238466,0.,-0.986259919523959));
#29586=DIRECTION('',(0.,1.,0.));
#29587=DIRECTION('center_axis',(0.968927638144812,0.,0.247344359222354));
#29588=DIRECTION('ref_axis',(0.247344359222354,0.,-0.968927638144812));
#29589=DIRECTION('',(0.,1.,0.));
#29590=DIRECTION('center_axis',(0.938956260693937,0.,0.344036539489135));
#29591=DIRECTION('ref_axis',(0.344036539489135,0.,-0.938956260693937));
#29592=DIRECTION('center_axis',(0.669864961350055,0.,-0.742482951693498));
#29593=DIRECTION('ref_axis',(-0.742482951693498,0.,-0.669864961350055));
#29594=DIRECTION('',(0.,1.,0.));
#29595=DIRECTION('center_axis',(0.742482951693498,0.,-0.669864961350055));
#29596=DIRECTION('ref_axis',(-0.669864961350055,0.,-0.742482951693498));
#29597=DIRECTION('',(0.,1.,0.));
#29598=DIRECTION('center_axis',(-0.63085575199153,0.,-0.775900135442186));
#29599=DIRECTION('ref_axis',(-0.775900135442185,0.,0.63085575199153));
#29600=DIRECTION('',(0.,1.,0.));
#29601=DIRECTION('center_axis',(-0.481508053781989,0.,-0.876441666138187));
#29602=DIRECTION('ref_axis',(-0.876441666138187,0.,0.481508053781989));
#29603=DIRECTION('center_axis',(-0.165201002238466,0.,-0.986259919523959));
#29604=DIRECTION('ref_axis',(-0.986259919523959,0.,0.165201002238466));
#29605=DIRECTION('',(0.,1.,0.));
#29606=DIRECTION('center_axis',(-0.0915937869476553,0.,-0.995796454197638));
#29607=DIRECTION('ref_axis',(-0.995796454197638,0.,0.0915937869476553));
#29608=DIRECTION('',(0.,1.,0.));
#29609=DIRECTION('center_axis',(-0.0238849697840649,0.,-0.999714713414989));
#29610=DIRECTION('ref_axis',(-0.99971471341499,0.,0.0238849697840649));
#29611=DIRECTION('',(0.,1.,0.));
#29612=DIRECTION('center_axis',(0.039351968002701,0.,-0.999225411313341));
#29613=DIRECTION('ref_axis',(-0.99922541131334,0.,-0.039351968002701));
#29614=DIRECTION('',(0.,1.,0.));
#29615=DIRECTION('center_axis',(0.0989820318029272,0.,-0.995089220813975));
#29616=DIRECTION('ref_axis',(-0.995089220813975,0.,-0.0989820318029272));
#29617=DIRECTION('',(0.,1.,0.));
#29618=DIRECTION('center_axis',(0.854702313102452,0.,-0.519118441184011));
#29619=DIRECTION('ref_axis',(-0.519118441184011,0.,-0.854702313102452));
#29620=DIRECTION('',(0.,1.,0.));
#29621=DIRECTION('center_axis',(0.862298277386211,0.,-0.506400711706425));
#29622=DIRECTION('ref_axis',(-0.506400711706425,0.,-0.862298277386211));
#29623=DIRECTION('',(0.,1.,0.));
#29624=DIRECTION('center_axis',(0.869705019525391,0.,-0.493571858002802));
#29625=DIRECTION('ref_axis',(-0.493571858002802,0.,-0.869705019525391));
#29626=DIRECTION('',(0.,1.,0.));
#29627=DIRECTION('center_axis',(0.876920914189558,0.,-0.480634695228039));
#29628=DIRECTION('ref_axis',(-0.480634695228039,0.,-0.876920914189558));
#29629=DIRECTION('',(0.,1.,0.));
#29630=DIRECTION('center_axis',(0.911263560158428,0.,0.411823656347455));
#29631=DIRECTION('ref_axis',(0.411823656347455,0.,-0.911263560158428));
#29632=DIRECTION('',(0.,1.,0.));
#29633=DIRECTION('center_axis',(0.885030574305657,0.,0.465532901677421));
#29634=DIRECTION('ref_axis',(0.465532901677421,0.,-0.885030574305657));
#29635=DIRECTION('',(0.,1.,0.));
#29636=DIRECTION('center_axis',(0.853835853462429,0.,0.520542347309117));
#29637=DIRECTION('ref_axis',(0.520542347309117,0.,-0.853835853462429));
#29638=DIRECTION('',(0.,1.,0.));
#29639=DIRECTION('center_axis',(0.816588132859795,0.,0.577220773424305));
#29640=DIRECTION('ref_axis',(0.577220773424305,0.,-0.816588132859795));
#29641=DIRECTION('',(0.,1.,0.));
#29642=DIRECTION('center_axis',(0.771525643922912,0.,0.636198224431141));
#29643=DIRECTION('ref_axis',(0.636198224431141,0.,-0.771525643922912));
#29644=DIRECTION('',(0.,1.,0.));
#29645=DIRECTION('center_axis',(0.715443769451088,0.,0.698670317641746));
#29646=DIRECTION('ref_axis',(0.698670317641746,0.,-0.715443769451088));
#29647=DIRECTION('',(0.,1.,0.));
#29648=DIRECTION('center_axis',(0.641141705058826,0.,0.767422513374648));
#29649=DIRECTION('ref_axis',(0.767422513374648,0.,-0.641141705058826));
#29650=DIRECTION('center_axis',(0.951361549480978,0.,-0.308076617368396));
#29651=DIRECTION('ref_axis',(-0.308076617368396,0.,-0.951361549480978));
#29652=DIRECTION('',(0.,1.,0.));
#29653=DIRECTION('center_axis',(0.977941578718451,0.,-0.208878597787478));
#29654=DIRECTION('ref_axis',(-0.208878597787478,0.,-0.977941578718451));
#29655=DIRECTION('',(0.,1.,0.));
#29656=DIRECTION('center_axis',(-0.158387039627108,0.,-0.987377104088484));
#29657=DIRECTION('ref_axis',(-0.987377104088484,0.,0.158387039627108));
#29658=DIRECTION('',(0.,1.,0.));
#29659=DIRECTION('center_axis',(0.0212226263670891,0.,-0.999774774701824));
#29660=DIRECTION('ref_axis',(-0.999774774701824,0.,-0.0212226263670891));
#29661=DIRECTION('center_axis',(0.350061695092817,0.,-0.936726646161378));
#29662=DIRECTION('ref_axis',(-0.936726646161378,0.,-0.350061695092817));
#29663=DIRECTION('',(0.,1.,0.));
#29664=DIRECTION('center_axis',(0.418575680773333,0.,-0.908181919807447));
#29665=DIRECTION('ref_axis',(-0.908181919807447,0.,-0.418575680773333));
#29666=DIRECTION('',(0.,1.,0.));
#29667=DIRECTION('center_axis',(0.479172366105871,0.,-0.877720823246493));
#29668=DIRECTION('ref_axis',(-0.877720823246493,0.,-0.479172366105871));
#29669=DIRECTION('',(0.,1.,0.));
#29670=DIRECTION('center_axis',(0.533692509635919,0.,-0.845678606302959));
#29671=DIRECTION('ref_axis',(-0.845678606302959,0.,-0.533692509635919));
#29672=DIRECTION('',(0.,1.,0.));
#29673=DIRECTION('center_axis',(0.583265564466523,0.,-0.812281528355501));
#29674=DIRECTION('ref_axis',(-0.812281528355501,0.,-0.583265564466523));
#29675=DIRECTION('',(0.,1.,0.));
#29676=DIRECTION('center_axis',(0.999753136412051,0.,-0.0222186010871084));
#29677=DIRECTION('ref_axis',(-0.0222186010871084,0.,-0.99975313641205));
#29678=DIRECTION('',(0.,1.,0.));
#29679=DIRECTION('center_axis',(0.999972569709232,0.,-0.00740674213917775));
#29680=DIRECTION('ref_axis',(-0.00740674213917775,0.,-0.999972569709231));
#29681=DIRECTION('',(0.,1.,0.));
#29682=DIRECTION('center_axis',(0.999972569709232,0.,0.00740674213917775));
#29683=DIRECTION('ref_axis',(0.00740674213917775,0.,-0.999972569709231));
#29684=DIRECTION('',(0.,1.,0.));
#29685=DIRECTION('center_axis',(0.999753136412051,0.,0.0222186010871084));
#29686=DIRECTION('ref_axis',(0.0222186010871084,0.,-0.99975313641205));
#29687=DIRECTION('',(0.,1.,0.));
#29688=DIRECTION('center_axis',(0.583265564466523,0.,0.812281528355501));
#29689=DIRECTION('ref_axis',(0.812281528355501,0.,-0.583265564466523));
#29690=DIRECTION('',(0.,1.,0.));
#29691=DIRECTION('center_axis',(0.533692509635919,0.,0.845678606302959));
#29692=DIRECTION('ref_axis',(0.845678606302959,0.,-0.533692509635919));
#29693=DIRECTION('',(0.,1.,0.));
#29694=DIRECTION('center_axis',(0.479172366105871,0.,0.877720823246493));
#29695=DIRECTION('ref_axis',(0.877720823246493,0.,-0.479172366105871));
#29696=DIRECTION('',(0.,1.,0.));
#29697=DIRECTION('center_axis',(0.418575680773333,0.,0.908181919807447));
#29698=DIRECTION('ref_axis',(0.908181919807447,0.,-0.418575680773333));
#29699=DIRECTION('',(0.,1.,0.));
#29700=DIRECTION('center_axis',(0.350061695092817,0.,0.936726646161378));
#29701=DIRECTION('ref_axis',(0.936726646161378,0.,-0.350061695092817));
#29702=DIRECTION('',(0.,1.,0.));
#29703=DIRECTION('center_axis',(0.270257320503069,0.,0.962788128673439));
#29704=DIRECTION('ref_axis',(0.962788128673439,0.,-0.270257320503069));
#29705=DIRECTION('',(0.,1.,0.));
#29706=DIRECTION('center_axis',(0.171533747319284,0.,0.985178244547962));
#29707=DIRECTION('ref_axis',(0.985178244547962,0.,-0.171533747319284));
#29708=DIRECTION('center_axis',(0.977941578718451,0.,0.208878597787478));
#29709=DIRECTION('ref_axis',(0.208878597787478,0.,-0.977941578718451));
#29710=DIRECTION('',(0.,1.,0.));
#29711=DIRECTION('center_axis',(0.951361549480978,0.,0.308076617368396));
#29712=DIRECTION('ref_axis',(0.308076617368396,0.,-0.951361549480978));
#29713=DIRECTION('',(0.,1.,0.));
#29714=DIRECTION('center_axis',(0.356521352096954,0.,-0.934287175069293));
#29715=DIRECTION('ref_axis',(-0.934287175069293,0.,-0.356521352096954));
#29716=DIRECTION('',(0.,1.,0.));
#29717=DIRECTION('center_axis',(0.518266720919835,0.,-0.855219039771099));
#29718=DIRECTION('ref_axis',(-0.855219039771099,0.,-0.518266720919835));
#29719=DIRECTION('center_axis',(0.771525643922912,0.,-0.636198224431141));
#29720=DIRECTION('ref_axis',(-0.636198224431141,0.,-0.771525643922912));
#29721=DIRECTION('',(0.,1.,0.));
#29722=DIRECTION('center_axis',(0.816588132859795,0.,-0.577220773424305));
#29723=DIRECTION('ref_axis',(-0.577220773424305,0.,-0.816588132859795));
#29724=DIRECTION('',(0.,1.,0.));
#29725=DIRECTION('center_axis',(0.853835853462429,0.,-0.520542347309117));
#29726=DIRECTION('ref_axis',(-0.520542347309117,0.,-0.853835853462429));
#29727=DIRECTION('',(0.,1.,0.));
#29728=DIRECTION('center_axis',(0.885030574305657,0.,-0.465532901677421));
#29729=DIRECTION('ref_axis',(-0.465532901677421,0.,-0.885030574305657));
#29730=DIRECTION('',(0.,1.,0.));
#29731=DIRECTION('center_axis',(0.911263560158428,0.,-0.411823656347455));
#29732=DIRECTION('ref_axis',(-0.411823656347455,0.,-0.911263560158428));
#29733=DIRECTION('',(0.,1.,0.));
#29734=DIRECTION('center_axis',(0.876920914189558,0.,0.480634695228039));
#29735=DIRECTION('ref_axis',(0.480634695228039,0.,-0.876920914189558));
#29736=DIRECTION('',(0.,1.,0.));
#29737=DIRECTION('center_axis',(0.869705019525391,0.,0.493571858002802));
#29738=DIRECTION('ref_axis',(0.493571858002802,0.,-0.869705019525391));
#29739=DIRECTION('',(0.,1.,0.));
#29740=DIRECTION('center_axis',(0.862298277386211,0.,0.506400711706425));
#29741=DIRECTION('ref_axis',(0.506400711706425,0.,-0.862298277386211));
#29742=DIRECTION('',(0.,1.,0.));
#29743=DIRECTION('center_axis',(0.854702313102452,0.,0.519118441184011));
#29744=DIRECTION('ref_axis',(0.519118441184011,0.,-0.854702313102452));
#29745=DIRECTION('',(0.,1.,0.));
#29746=DIRECTION('center_axis',(0.0989820318029272,0.,0.995089220813975));
#29747=DIRECTION('ref_axis',(0.995089220813975,0.,-0.0989820318029272));
#29748=DIRECTION('',(0.,1.,0.));
#29749=DIRECTION('center_axis',(0.039351968002701,0.,0.999225411313341));
#29750=DIRECTION('ref_axis',(0.99922541131334,0.,-0.039351968002701));
#29751=DIRECTION('',(0.,1.,0.));
#29752=DIRECTION('center_axis',(-0.0238849697840649,0.,0.999714713414989));
#29753=DIRECTION('ref_axis',(0.99971471341499,0.,0.0238849697840649));
#29754=DIRECTION('',(0.,1.,0.));
#29755=DIRECTION('center_axis',(-0.0915937869476553,0.,0.995796454197638));
#29756=DIRECTION('ref_axis',(0.995796454197638,0.,0.0915937869476553));
#29757=DIRECTION('',(0.,1.,0.));
#29758=DIRECTION('center_axis',(-0.165201002238466,0.,0.986259919523959));
#29759=DIRECTION('ref_axis',(0.986259919523959,0.,0.165201002238466));
#29760=DIRECTION('',(0.,1.,0.));
#29761=DIRECTION('center_axis',(-0.247344359222349,0.,0.968927638144813));
#29762=DIRECTION('ref_axis',(0.968927638144813,0.,0.247344359222349));
#29763=DIRECTION('',(0.,1.,0.));
#29764=DIRECTION('center_axis',(-0.344036539489138,0.,0.938956260693936));
#29765=DIRECTION('ref_axis',(0.938956260693936,0.,0.344036539489138));
#29766=DIRECTION('center_axis',(0.742482951693498,0.,0.669864961350055));
#29767=DIRECTION('ref_axis',(0.669864961350055,0.,-0.742482951693498));
#29768=DIRECTION('',(0.,1.,0.));
#29769=DIRECTION('center_axis',(0.669864961350055,0.,0.742482951693498));
#29770=DIRECTION('ref_axis',(0.742482951693498,0.,-0.669864961350055));
#29771=DIRECTION('',(0.,1.,0.));
#29772=DIRECTION('center_axis',(0.775900135442185,0.,-0.630855751991531));
#29773=DIRECTION('ref_axis',(-0.63085575199153,0.,-0.775900135442185));
#29774=DIRECTION('',(0.,1.,0.));
#29775=DIRECTION('center_axis',(0.876441666138186,0.,-0.481508053781991));
#29776=DIRECTION('ref_axis',(-0.481508053781991,0.,-0.876441666138186));
#29777=DIRECTION('center_axis',(0.986259919523959,0.,-0.165201002238466));
#29778=DIRECTION('ref_axis',(-0.165201002238466,0.,-0.986259919523959));
#29779=DIRECTION('',(0.,1.,0.));
#29780=DIRECTION('center_axis',(0.995796454197638,0.,-0.0915937869476482));
#29781=DIRECTION('ref_axis',(-0.0915937869476482,0.,-0.995796454197638));
#29782=DIRECTION('',(0.,1.,0.));
#29783=DIRECTION('center_axis',(0.999714713414989,0.,-0.0238849697840649));
#29784=DIRECTION('ref_axis',(-0.0238849697840649,0.,-0.99971471341499));
#29785=DIRECTION('',(0.,1.,0.));
#29786=DIRECTION('center_axis',(0.999225411313341,0.,0.0393519680027008));
#29787=DIRECTION('ref_axis',(0.0393519680027008,0.,-0.999225411313341));
#29788=DIRECTION('',(0.,1.,0.));
#29789=DIRECTION('center_axis',(0.995089220813976,0.,0.0989820318029246));
#29790=DIRECTION('ref_axis',(0.0989820318029246,0.,-0.995089220813976));
#29791=DIRECTION('',(0.,1.,0.));
#29792=DIRECTION('center_axis',(0.519118441184015,0.,0.85470231310245));
#29793=DIRECTION('ref_axis',(0.85470231310245,0.,-0.519118441184015));
#29794=DIRECTION('',(0.,1.,0.));
#29795=DIRECTION('center_axis',(0.506400711706423,0.,0.862298277386212));
#29796=DIRECTION('ref_axis',(0.862298277386212,0.,-0.506400711706423));
#29797=DIRECTION('',(0.,1.,0.));
#29798=DIRECTION('center_axis',(0.493571858002813,0.,0.869705019525386));
#29799=DIRECTION('ref_axis',(0.869705019525386,0.,-0.493571858002812));
#29800=DIRECTION('',(0.,1.,0.));
#29801=DIRECTION('center_axis',(0.480634695228032,0.,0.876920914189562));
#29802=DIRECTION('ref_axis',(0.876920914189562,0.,-0.480634695228032));
#29803=DIRECTION('',(0.,1.,0.));
#29804=DIRECTION('center_axis',(-0.411823656347449,0.,0.911263560158431));
#29805=DIRECTION('ref_axis',(0.911263560158431,0.,0.411823656347449));
#29806=DIRECTION('',(0.,1.,0.));
#29807=DIRECTION('center_axis',(-0.465532901677421,0.,0.885030574305657));
#29808=DIRECTION('ref_axis',(0.885030574305657,0.,0.465532901677421));
#29809=DIRECTION('',(0.,1.,0.));
#29810=DIRECTION('center_axis',(-0.520542347309119,0.,0.853835853462428));
#29811=DIRECTION('ref_axis',(0.853835853462428,0.,0.520542347309119));
#29812=DIRECTION('',(0.,1.,0.));
#29813=DIRECTION('center_axis',(-0.577220773424304,0.,0.816588132859796));
#29814=DIRECTION('ref_axis',(0.816588132859796,0.,0.577220773424304));
#29815=DIRECTION('',(0.,1.,0.));
#29816=DIRECTION('center_axis',(-0.63619822443114,0.,0.771525643922913));
#29817=DIRECTION('ref_axis',(0.771525643922913,0.,0.63619822443114));
#29818=DIRECTION('',(0.,1.,0.));
#29819=DIRECTION('center_axis',(-0.698670317641747,0.,0.715443769451087));
#29820=DIRECTION('ref_axis',(0.715443769451087,0.,0.698670317641747));
#29821=DIRECTION('',(0.,1.,0.));
#29822=DIRECTION('center_axis',(-0.767422513374647,0.,0.641141705058827));
#29823=DIRECTION('ref_axis',(0.641141705058827,0.,0.767422513374647));
#29824=DIRECTION('center_axis',(0.308076617368396,0.,0.951361549480978));
#29825=DIRECTION('ref_axis',(0.951361549480978,0.,-0.308076617368396));
#29826=DIRECTION('',(0.,1.,0.));
#29827=DIRECTION('center_axis',(0.208878597787478,0.,0.977941578718451));
#29828=DIRECTION('ref_axis',(0.977941578718451,0.,-0.208878597787478));
#29829=DIRECTION('',(0.,1.,0.));
#29830=DIRECTION('center_axis',(0.987377104088484,0.,-0.158387039627108));
#29831=DIRECTION('ref_axis',(-0.158387039627108,0.,-0.987377104088484));
#29832=DIRECTION('',(0.,1.,0.));
#29833=DIRECTION('center_axis',(0.999774774701824,0.,0.0212226263670855));
#29834=DIRECTION('ref_axis',(0.0212226263670855,0.,-0.999774774701824));
#29835=DIRECTION('center_axis',(0.936726646161378,0.,0.350061695092817));
#29836=DIRECTION('ref_axis',(0.350061695092817,0.,-0.936726646161378));
#29837=DIRECTION('',(0.,1.,0.));
#29838=DIRECTION('center_axis',(0.908181919807446,0.,0.418575680773335));
#29839=DIRECTION('ref_axis',(0.418575680773335,0.,-0.908181919807446));
#29840=DIRECTION('',(0.,1.,0.));
#29841=DIRECTION('center_axis',(0.877720823246492,0.,0.479172366105872));
#29842=DIRECTION('ref_axis',(0.479172366105872,0.,-0.877720823246493));
#29843=DIRECTION('',(0.,1.,0.));
#29844=DIRECTION('center_axis',(0.845678606302959,0.,0.533692509635919));
#29845=DIRECTION('ref_axis',(0.533692509635919,0.,-0.845678606302959));
#29846=DIRECTION('',(0.,1.,0.));
#29847=DIRECTION('center_axis',(0.812281528355501,0.,0.583265564466523));
#29848=DIRECTION('ref_axis',(0.583265564466523,0.,-0.812281528355501));
#29849=DIRECTION('',(0.,1.,0.));
#29850=DIRECTION('center_axis',(0.0222186010871084,0.,0.999753136412051));
#29851=DIRECTION('ref_axis',(0.99975313641205,0.,-0.0222186010871084));
#29852=DIRECTION('',(0.,1.,0.));
#29853=DIRECTION('center_axis',(0.00740674213917776,0.,0.999972569709231));
#29854=DIRECTION('ref_axis',(0.999972569709231,0.,-0.00740674213917776));
#29855=DIRECTION('',(0.,1.,0.));
#29856=DIRECTION('center_axis',(-0.00740674213917776,0.,0.999972569709231));
#29857=DIRECTION('ref_axis',(0.999972569709231,0.,0.00740674213917776));
#29858=DIRECTION('',(0.,1.,0.));
#29859=DIRECTION('center_axis',(-0.0222186010871085,0.,0.999753136412051));
#29860=DIRECTION('ref_axis',(0.99975313641205,0.,0.0222186010871085));
#29861=DIRECTION('',(0.,1.,0.));
#29862=DIRECTION('center_axis',(-0.812281528355501,0.,0.583265564466523));
#29863=DIRECTION('ref_axis',(0.583265564466523,0.,0.812281528355501));
#29864=DIRECTION('',(0.,1.,0.));
#29865=DIRECTION('center_axis',(-0.845678606302959,0.,0.533692509635919));
#29866=DIRECTION('ref_axis',(0.533692509635919,0.,0.845678606302959));
#29867=DIRECTION('',(0.,1.,0.));
#29868=DIRECTION('center_axis',(-0.877720823246492,0.,0.479172366105872));
#29869=DIRECTION('ref_axis',(0.479172366105872,0.,0.877720823246493));
#29870=DIRECTION('',(0.,1.,0.));
#29871=DIRECTION('center_axis',(-0.908181919807446,0.,0.418575680773336));
#29872=DIRECTION('ref_axis',(0.418575680773336,0.,0.908181919807446));
#29873=DIRECTION('',(0.,1.,0.));
#29874=DIRECTION('center_axis',(-0.936726646161378,0.,0.350061695092817));
#29875=DIRECTION('ref_axis',(0.350061695092817,0.,0.936726646161378));
#29876=DIRECTION('',(0.,1.,0.));
#29877=DIRECTION('center_axis',(-0.962788128673439,0.,0.270257320503068));
#29878=DIRECTION('ref_axis',(0.270257320503068,0.,0.962788128673439));
#29879=DIRECTION('',(0.,1.,0.));
#29880=DIRECTION('center_axis',(-0.985178244547962,0.,0.171533747319286));
#29881=DIRECTION('ref_axis',(0.171533747319286,0.,0.985178244547962));
#29882=DIRECTION('center_axis',(-0.208878597787479,0.,0.977941578718451));
#29883=DIRECTION('ref_axis',(0.977941578718451,0.,0.208878597787479));
#29884=DIRECTION('',(0.,1.,0.));
#29885=DIRECTION('center_axis',(-0.308076617368397,0.,0.951361549480978));
#29886=DIRECTION('ref_axis',(0.951361549480978,0.,0.308076617368397));
#29887=DIRECTION('',(0.,1.,0.));
#29888=DIRECTION('center_axis',(0.934287175069293,0.,0.356521352096954));
#29889=DIRECTION('ref_axis',(0.356521352096954,0.,-0.934287175069293));
#29890=DIRECTION('',(0.,1.,0.));
#29891=DIRECTION('center_axis',(0.8552190397711,0.,0.518266720919834));
#29892=DIRECTION('ref_axis',(0.518266720919834,0.,-0.8552190397711));
#29893=DIRECTION('center_axis',(0.636198224431142,0.,0.771525643922911));
#29894=DIRECTION('ref_axis',(0.771525643922911,0.,-0.636198224431142));
#29895=DIRECTION('',(0.,1.,0.));
#29896=DIRECTION('center_axis',(0.577220773424306,0.,0.816588132859795));
#29897=DIRECTION('ref_axis',(0.816588132859795,0.,-0.577220773424306));
#29898=DIRECTION('',(0.,1.,0.));
#29899=DIRECTION('center_axis',(0.520542347309119,0.,0.853835853462428));
#29900=DIRECTION('ref_axis',(0.853835853462428,0.,-0.520542347309119));
#29901=DIRECTION('',(0.,1.,0.));
#29902=DIRECTION('center_axis',(0.46553290167742,0.,0.885030574305657));
#29903=DIRECTION('ref_axis',(0.885030574305657,0.,-0.46553290167742));
#29904=DIRECTION('',(0.,1.,0.));
#29905=DIRECTION('center_axis',(0.411823656347453,0.,0.911263560158429));
#29906=DIRECTION('ref_axis',(0.911263560158429,0.,-0.411823656347453));
#29907=DIRECTION('',(0.,1.,0.));
#29908=DIRECTION('center_axis',(-0.48063469522804,0.,0.876920914189557));
#29909=DIRECTION('ref_axis',(0.876920914189557,0.,0.48063469522804));
#29910=DIRECTION('',(0.,1.,0.));
#29911=DIRECTION('center_axis',(-0.493571858002805,0.,0.86970501952539));
#29912=DIRECTION('ref_axis',(0.86970501952539,0.,0.493571858002805));
#29913=DIRECTION('',(0.,1.,0.));
#29914=DIRECTION('center_axis',(-0.506400711706427,0.,0.86229827738621));
#29915=DIRECTION('ref_axis',(0.86229827738621,0.,0.506400711706427));
#29916=DIRECTION('',(0.,1.,0.));
#29917=DIRECTION('center_axis',(-0.519118441184015,0.,0.85470231310245));
#29918=DIRECTION('ref_axis',(0.85470231310245,0.,0.519118441184015));
#29919=DIRECTION('',(0.,1.,0.));
#29920=DIRECTION('center_axis',(-0.995089220813975,0.,0.0989820318029307));
#29921=DIRECTION('ref_axis',(0.0989820318029307,0.,0.995089220813975));
#29922=DIRECTION('',(0.,1.,0.));
#29923=DIRECTION('center_axis',(-0.999225411313341,0.,0.0393519680026976));
#29924=DIRECTION('ref_axis',(0.0393519680026975,0.,0.999225411313341));
#29925=DIRECTION('',(0.,1.,0.));
#29926=DIRECTION('center_axis',(-0.99971471341499,0.,-0.0238849697840614));
#29927=DIRECTION('ref_axis',(-0.0238849697840614,0.,0.99971471341499));
#29928=DIRECTION('',(0.,1.,0.));
#29929=DIRECTION('center_axis',(-0.995796454197637,0.,-0.0915937869476591));
#29930=DIRECTION('ref_axis',(-0.0915937869476591,0.,0.995796454197637));
#29931=DIRECTION('',(0.,1.,0.));
#29932=DIRECTION('center_axis',(-0.98625991952396,0.,-0.165201002238462));
#29933=DIRECTION('ref_axis',(-0.165201002238462,0.,0.98625991952396));
#29934=DIRECTION('',(0.,1.,0.));
#29935=DIRECTION('center_axis',(-0.968927638144813,0.,-0.247344359222349));
#29936=DIRECTION('ref_axis',(-0.247344359222349,0.,0.968927638144813));
#29937=DIRECTION('',(0.,1.,0.));
#29938=DIRECTION('center_axis',(-0.938956260693934,0.,-0.344036539489144));
#29939=DIRECTION('ref_axis',(-0.344036539489144,0.,0.938956260693934));
#29940=DIRECTION('center_axis',(-0.669864961350055,0.,0.742482951693498));
#29941=DIRECTION('ref_axis',(0.742482951693498,0.,0.669864961350055));
#29942=DIRECTION('',(0.,1.,0.));
#29943=DIRECTION('center_axis',(-0.742482951693498,0.,0.669864961350055));
#29944=DIRECTION('ref_axis',(0.669864961350055,0.,0.742482951693498));
#29945=DIRECTION('',(0.,1.,0.));
#29946=DIRECTION('center_axis',(0.630855751991531,0.,0.775900135442185));
#29947=DIRECTION('ref_axis',(0.775900135442185,0.,-0.63085575199153));
#29948=DIRECTION('',(0.,1.,0.));
#29949=DIRECTION('center_axis',(0.48150805378198,0.,0.876441666138192));
#29950=DIRECTION('ref_axis',(0.876441666138192,0.,-0.48150805378198));
#29951=DIRECTION('center_axis',(0.165201002238459,0.,0.98625991952396));
#29952=DIRECTION('ref_axis',(0.98625991952396,0.,-0.165201002238459));
#29953=DIRECTION('',(0.,1.,0.));
#29954=DIRECTION('center_axis',(0.0915937869476627,0.,0.995796454197637));
#29955=DIRECTION('ref_axis',(0.995796454197637,0.,-0.0915937869476627));
#29956=DIRECTION('',(0.,1.,0.));
#29957=DIRECTION('center_axis',(0.0238849697840613,0.,0.99971471341499));
#29958=DIRECTION('ref_axis',(0.99971471341499,0.,-0.0238849697840613));
#29959=DIRECTION('',(0.,1.,0.));
#29960=DIRECTION('center_axis',(-0.0393519680026977,0.,0.999225411313341));
#29961=DIRECTION('ref_axis',(0.999225411313341,0.,0.0393519680026977));
#29962=DIRECTION('',(0.,1.,0.));
#29963=DIRECTION('center_axis',(-0.0989820318029304,0.,0.995089220813975));
#29964=DIRECTION('ref_axis',(0.995089220813975,0.,0.0989820318029304));
#29965=DIRECTION('',(0.,1.,0.));
#29966=DIRECTION('center_axis',(-0.854702313102456,0.,0.519118441184006));
#29967=DIRECTION('ref_axis',(0.519118441184006,0.,0.854702313102456));
#29968=DIRECTION('',(0.,1.,0.));
#29969=DIRECTION('center_axis',(-0.862298277386207,0.,0.506400711706431));
#29970=DIRECTION('ref_axis',(0.506400711706431,0.,0.862298277386207));
#29971=DIRECTION('',(0.,1.,0.));
#29972=DIRECTION('center_axis',(-0.869705019525391,0.,0.493571858002802));
#29973=DIRECTION('ref_axis',(0.493571858002802,0.,0.869705019525391));
#29974=DIRECTION('',(0.,1.,0.));
#29975=DIRECTION('center_axis',(-0.876920914189556,0.,0.480634695228042));
#29976=DIRECTION('ref_axis',(0.480634695228042,0.,0.876920914189556));
#29977=DIRECTION('',(0.,1.,0.));
#29978=DIRECTION('center_axis',(-0.91126356015843,0.,-0.41182365634745));
#29979=DIRECTION('ref_axis',(-0.41182365634745,0.,0.91126356015843));
#29980=DIRECTION('',(0.,1.,0.));
#29981=DIRECTION('center_axis',(-0.885030574305655,0.,-0.465532901677425));
#29982=DIRECTION('ref_axis',(-0.465532901677425,0.,0.885030574305655));
#29983=DIRECTION('',(0.,1.,0.));
#29984=DIRECTION('center_axis',(-0.85383585346243,0.,-0.520542347309115));
#29985=DIRECTION('ref_axis',(-0.520542347309115,0.,0.85383585346243));
#29986=DIRECTION('',(0.,1.,0.));
#29987=DIRECTION('center_axis',(-0.816588132859791,0.,-0.577220773424311));
#29988=DIRECTION('ref_axis',(-0.577220773424311,0.,0.816588132859791));
#29989=DIRECTION('',(0.,1.,0.));
#29990=DIRECTION('center_axis',(-0.771525643922916,0.,-0.636198224431136));
#29991=DIRECTION('ref_axis',(-0.636198224431136,0.,0.771525643922916));
#29992=DIRECTION('',(0.,1.,0.));
#29993=DIRECTION('center_axis',(-0.715443769451087,0.,-0.698670317641747));
#29994=DIRECTION('ref_axis',(-0.698670317641747,0.,0.715443769451087));
#29995=DIRECTION('',(0.,1.,0.));
#29996=DIRECTION('center_axis',(-0.641141705058821,0.,-0.767422513374652));
#29997=DIRECTION('ref_axis',(-0.767422513374652,0.,0.641141705058821));
#29998=DIRECTION('center_axis',(-0.951361549480978,0.,0.308076617368396));
#29999=DIRECTION('ref_axis',(0.308076617368396,0.,0.951361549480978));
#30000=DIRECTION('',(0.,1.,0.));
#30001=DIRECTION('center_axis',(-0.977941578718451,0.,0.20887859778748));
#30002=DIRECTION('ref_axis',(0.20887859778748,0.,0.977941578718451));
#30003=DIRECTION('',(0.,1.,0.));
#30004=DIRECTION('center_axis',(0.158387039627109,0.,0.987377104088484));
#30005=DIRECTION('ref_axis',(0.987377104088484,0.,-0.158387039627109));
#30006=DIRECTION('',(0.,1.,0.));
#30007=DIRECTION('center_axis',(-0.0212226263670972,0.,0.999774774701824));
#30008=DIRECTION('ref_axis',(0.999774774701824,0.,0.0212226263670972));
#30009=DIRECTION('center_axis',(-0.350061695092823,0.,0.936726646161376));
#30010=DIRECTION('ref_axis',(0.936726646161376,0.,0.350061695092823));
#30011=DIRECTION('',(0.,1.,0.));
#30012=DIRECTION('center_axis',(-0.418575680773325,0.,0.908181919807451));
#30013=DIRECTION('ref_axis',(0.908181919807451,0.,0.418575680773325));
#30014=DIRECTION('',(0.,1.,0.));
#30015=DIRECTION('center_axis',(-0.479172366105876,0.,0.87772082324649));
#30016=DIRECTION('ref_axis',(0.87772082324649,0.,0.479172366105876));
#30017=DIRECTION('',(0.,1.,0.));
#30018=DIRECTION('center_axis',(-0.533692509635917,0.,0.84567860630296));
#30019=DIRECTION('ref_axis',(0.84567860630296,0.,0.533692509635917));
#30020=DIRECTION('',(0.,1.,0.));
#30021=DIRECTION('center_axis',(-0.583265564466524,0.,0.8122815283555));
#30022=DIRECTION('ref_axis',(0.8122815283555,0.,0.583265564466524));
#30023=DIRECTION('',(0.,1.,0.));
#30024=DIRECTION('center_axis',(-0.999753136412051,0.,0.0222186010871084));
#30025=DIRECTION('ref_axis',(0.0222186010871084,0.,0.99975313641205));
#30026=DIRECTION('',(0.,1.,0.));
#30027=DIRECTION('center_axis',(-0.999972569709231,0.,0.00740674213917776));
#30028=DIRECTION('ref_axis',(0.00740674213917776,0.,0.999972569709231));
#30029=DIRECTION('',(0.,1.,0.));
#30030=DIRECTION('center_axis',(-0.999972569709231,0.,-0.00740674213917776));
#30031=DIRECTION('ref_axis',(-0.00740674213917776,0.,0.999972569709231));
#30032=DIRECTION('',(0.,1.,0.));
#30033=DIRECTION('center_axis',(-0.999753136412051,0.,-0.0222186010871084));
#30034=DIRECTION('ref_axis',(-0.0222186010871084,0.,0.99975313641205));
#30035=DIRECTION('',(0.,1.,0.));
#30036=DIRECTION('center_axis',(-0.583265564466527,0.,-0.812281528355498));
#30037=DIRECTION('ref_axis',(-0.812281528355498,0.,0.583265564466527));
#30038=DIRECTION('',(0.,1.,0.));
#30039=DIRECTION('center_axis',(-0.533692509635915,0.,-0.845678606302962));
#30040=DIRECTION('ref_axis',(-0.845678606302961,0.,0.533692509635915));
#30041=DIRECTION('',(0.,1.,0.));
#30042=DIRECTION('center_axis',(-0.479172366105876,0.,-0.87772082324649));
#30043=DIRECTION('ref_axis',(-0.87772082324649,0.,0.479172366105876));
#30044=DIRECTION('',(0.,1.,0.));
#30045=DIRECTION('center_axis',(-0.418575680773326,0.,-0.908181919807451));
#30046=DIRECTION('ref_axis',(-0.908181919807451,0.,0.418575680773326));
#30047=DIRECTION('',(0.,1.,0.));
#30048=DIRECTION('center_axis',(-0.350061695092823,0.,-0.936726646161376));
#30049=DIRECTION('ref_axis',(-0.936726646161376,0.,0.350061695092823));
#30050=DIRECTION('',(0.,1.,0.));
#30051=DIRECTION('center_axis',(-0.270257320503067,0.,-0.962788128673439));
#30052=DIRECTION('ref_axis',(-0.962788128673439,0.,0.270257320503067));
#30053=DIRECTION('',(0.,1.,0.));
#30054=DIRECTION('center_axis',(-0.171533747319281,0.,-0.985178244547963));
#30055=DIRECTION('ref_axis',(-0.985178244547962,0.,0.171533747319281));
#30056=DIRECTION('center_axis',(-0.977941578718451,0.,-0.208878597787478));
#30057=DIRECTION('ref_axis',(-0.208878597787478,0.,0.977941578718451));
#30058=DIRECTION('',(0.,1.,0.));
#30059=DIRECTION('center_axis',(-0.951361549480978,0.,-0.308076617368396));
#30060=DIRECTION('ref_axis',(-0.308076617368396,0.,0.951361549480978));
#30061=DIRECTION('',(0.,1.,0.));
#30062=DIRECTION('center_axis',(-0.356521352096954,0.,0.934287175069293));
#30063=DIRECTION('ref_axis',(0.934287175069293,0.,0.356521352096954));
#30064=DIRECTION('',(0.,1.,0.));
#30065=DIRECTION('center_axis',(-0.518266720919843,0.,0.855219039771095));
#30066=DIRECTION('ref_axis',(0.855219039771095,0.,0.518266720919843));
#30067=DIRECTION('center_axis',(-0.771525643922917,0.,0.636198224431135));
#30068=DIRECTION('ref_axis',(0.636198224431135,0.,0.771525643922917));
#30069=DIRECTION('',(0.,1.,0.));
#30070=DIRECTION('center_axis',(-0.81658813285979,0.,0.577220773424313));
#30071=DIRECTION('ref_axis',(0.577220773424313,0.,0.81658813285979));
#30072=DIRECTION('',(0.,1.,0.));
#30073=DIRECTION('center_axis',(-0.85383585346243,0.,0.520542347309115));
#30074=DIRECTION('ref_axis',(0.520542347309115,0.,0.85383585346243));
#30075=DIRECTION('',(0.,1.,0.));
#30076=DIRECTION('center_axis',(-0.885030574305656,0.,0.465532901677422));
#30077=DIRECTION('ref_axis',(0.465532901677422,0.,0.885030574305656));
#30078=DIRECTION('',(0.,1.,0.));
#30079=DIRECTION('center_axis',(-0.911263560158432,0.,0.411823656347447));
#30080=DIRECTION('ref_axis',(0.411823656347447,0.,0.911263560158432));
#30081=DIRECTION('',(0.,1.,0.));
#30082=DIRECTION('center_axis',(-0.876920914189563,0.,-0.48063469522803));
#30083=DIRECTION('ref_axis',(-0.48063469522803,0.,0.876920914189563));
#30084=DIRECTION('',(0.,1.,0.));
#30085=DIRECTION('center_axis',(-0.869705019525385,0.,-0.493571858002814));
#30086=DIRECTION('ref_axis',(-0.493571858002814,0.,0.869705019525385));
#30087=DIRECTION('',(0.,1.,0.));
#30088=DIRECTION('center_axis',(-0.862298277386214,0.,-0.506400711706419));
#30089=DIRECTION('ref_axis',(-0.506400711706419,0.,0.862298277386214));
#30090=DIRECTION('',(0.,1.,0.));
#30091=DIRECTION('center_axis',(-0.854702313102448,0.,-0.519118441184019));
#30092=DIRECTION('ref_axis',(-0.519118441184019,0.,0.854702313102448));
#30093=DIRECTION('',(0.,1.,0.));
#30094=DIRECTION('center_axis',(-0.0989820318029307,0.,-0.995089220813975));
#30095=DIRECTION('ref_axis',(-0.995089220813975,0.,0.0989820318029307));
#30096=DIRECTION('',(0.,1.,0.));
#30097=DIRECTION('center_axis',(-0.0393519680026942,0.,-0.999225411313341));
#30098=DIRECTION('ref_axis',(-0.999225411313341,0.,0.0393519680026942));
#30099=DIRECTION('',(0.,1.,0.));
#30100=DIRECTION('center_axis',(0.023884969784058,0.,-0.99971471341499));
#30101=DIRECTION('ref_axis',(-0.99971471341499,0.,-0.023884969784058));
#30102=DIRECTION('',(0.,1.,0.));
#30103=DIRECTION('center_axis',(0.091593786947663,0.,-0.995796454197637));
#30104=DIRECTION('ref_axis',(-0.995796454197637,0.,-0.091593786947663));
#30105=DIRECTION('',(0.,1.,0.));
#30106=DIRECTION('center_axis',(0.165201002238458,0.,-0.986259919523961));
#30107=DIRECTION('ref_axis',(-0.986259919523961,0.,-0.165201002238458));
#30108=DIRECTION('',(0.,1.,0.));
#30109=DIRECTION('center_axis',(0.247344359222354,0.,-0.968927638144812));
#30110=DIRECTION('ref_axis',(-0.968927638144812,0.,-0.247344359222354));
#30111=DIRECTION('',(0.,1.,0.));
#30112=DIRECTION('center_axis',(0.344036539489142,0.,-0.938956260693935));
#30113=DIRECTION('ref_axis',(-0.938956260693935,0.,-0.344036539489142));
#30114=DIRECTION('center_axis',(-0.742482951693499,0.,-0.669864961350053));
#30115=DIRECTION('ref_axis',(-0.669864961350053,0.,0.742482951693499));
#30116=DIRECTION('',(0.,1.,0.));
#30117=DIRECTION('center_axis',(-0.669864961350055,0.,-0.742482951693498));
#30118=DIRECTION('ref_axis',(-0.742482951693498,0.,0.669864961350055));
#30119=DIRECTION('',(0.,1.,0.));
#30120=DIRECTION('center_axis',(-0.775900135442185,0.,0.630855751991531));
#30121=DIRECTION('ref_axis',(0.630855751991531,0.,0.775900135442185));
#30122=DIRECTION('',(0.,1.,0.));
#30123=DIRECTION('center_axis',(-0.876441666138186,0.,0.481508053781991));
#30124=DIRECTION('ref_axis',(0.481508053781991,0.,0.876441666138186));
#30125=DIRECTION('center_axis',(-0.986259919523958,0.,0.165201002238474));
#30126=DIRECTION('ref_axis',(0.165201002238474,0.,0.986259919523958));
#30127=DIRECTION('',(0.,1.,0.));
#30128=DIRECTION('center_axis',(-0.995796454197638,0.,0.0915937869476479));
#30129=DIRECTION('ref_axis',(0.0915937869476479,0.,0.995796454197638));
#30130=DIRECTION('',(0.,1.,0.));
#30131=DIRECTION('center_axis',(-0.999714713414989,0.,0.0238849697840824));
#30132=DIRECTION('ref_axis',(0.0238849697840824,0.,0.999714713414989));
#30133=DIRECTION('',(0.,1.,0.));
#30134=DIRECTION('center_axis',(-0.99922541131334,0.,-0.0393519680027076));
#30135=DIRECTION('ref_axis',(-0.0393519680027076,0.,0.99922541131334));
#30136=DIRECTION('',(0.,1.,0.));
#30137=DIRECTION('center_axis',(-0.995089220813975,0.,-0.0989820318029304));
#30138=DIRECTION('ref_axis',(-0.0989820318029304,0.,0.995089220813975));
#30139=DIRECTION('',(0.,1.,0.));
#30140=DIRECTION('center_axis',(-0.51911844118402,0.,-0.854702313102447));
#30141=DIRECTION('ref_axis',(-0.854702313102447,0.,0.51911844118402));
#30142=DIRECTION('',(0.,1.,0.));
#30143=DIRECTION('center_axis',(-0.506400711706418,0.,-0.862298277386215));
#30144=DIRECTION('ref_axis',(-0.862298277386214,0.,0.506400711706418));
#30145=DIRECTION('',(0.,1.,0.));
#30146=DIRECTION('center_axis',(-0.493571858002809,0.,-0.869705019525388));
#30147=DIRECTION('ref_axis',(-0.869705019525388,0.,0.493571858002809));
#30148=DIRECTION('',(0.,1.,0.));
#30149=DIRECTION('center_axis',(-0.480634695228043,0.,-0.876920914189556));
#30150=DIRECTION('ref_axis',(-0.876920914189556,0.,0.480634695228043));
#30151=DIRECTION('',(0.,1.,0.));
#30152=DIRECTION('center_axis',(0.411823656347446,0.,-0.911263560158432));
#30153=DIRECTION('ref_axis',(-0.911263560158432,0.,-0.411823656347446));
#30154=DIRECTION('',(0.,1.,0.));
#30155=DIRECTION('center_axis',(0.465532901677419,0.,-0.885030574305658));
#30156=DIRECTION('ref_axis',(-0.885030574305658,0.,-0.465532901677419));
#30157=DIRECTION('',(0.,1.,0.));
#30158=DIRECTION('center_axis',(0.520542347309132,0.,-0.85383585346242));
#30159=DIRECTION('ref_axis',(-0.85383585346242,0.,-0.520542347309132));
#30160=DIRECTION('',(0.,1.,0.));
#30161=DIRECTION('center_axis',(0.577220773424303,0.,-0.816588132859797));
#30162=DIRECTION('ref_axis',(-0.816588132859797,0.,-0.577220773424303));
#30163=DIRECTION('',(0.,1.,0.));
#30164=DIRECTION('center_axis',(0.636198224431145,0.,-0.771525643922909));
#30165=DIRECTION('ref_axis',(-0.771525643922909,0.,-0.636198224431145));
#30166=DIRECTION('',(0.,1.,0.));
#30167=DIRECTION('center_axis',(0.69867031764173,0.,-0.715443769451104));
#30168=DIRECTION('ref_axis',(-0.715443769451104,0.,-0.69867031764173));
#30169=DIRECTION('',(0.,1.,0.));
#30170=DIRECTION('center_axis',(0.767422513374652,0.,-0.641141705058821));
#30171=DIRECTION('ref_axis',(-0.641141705058821,0.,-0.767422513374652));
#30172=DIRECTION('center_axis',(-0.308076617368395,0.,-0.951361549480978));
#30173=DIRECTION('ref_axis',(-0.951361549480978,0.,0.308076617368395));
#30174=DIRECTION('center_axis',(0.,1.,0.));
#30175=DIRECTION('ref_axis',(0.,0.,1.));
#30176=DIRECTION('',(0.,-1.,0.));
#30177=DIRECTION('center_axis',(0.,1.,0.));
#30178=DIRECTION('ref_axis',(1.,0.,0.));
#30179=DIRECTION('center_axis',(0.,-1.,0.));
#30180=DIRECTION('ref_axis',(0.,0.,-1.));
#30181=DIRECTION('center_axis',(0.,1.,0.));
#30182=DIRECTION('ref_axis',(1.,0.,0.));
#30183=DIRECTION('center_axis',(0.,1.,0.));
#30184=DIRECTION('ref_axis',(0.,0.,1.));
#30185=DIRECTION('center_axis',(0.,1.,0.));
#30186=DIRECTION('ref_axis',(1.,0.,0.));
#30187=DIRECTION('',(8.65956056235491E-17,-0.707106781186549,0.707106781186546));
#30188=DIRECTION('center_axis',(0.,1.,0.));
#30189=DIRECTION('ref_axis',(0.,0.,1.));
#30190=DIRECTION('center_axis',(0.,1.,0.));
#30191=DIRECTION('ref_axis',(1.,0.,0.));
#30192=DIRECTION('',(0.,-1.,0.));
#30193=DIRECTION('center_axis',(0.,-1.,0.));
#30194=DIRECTION('ref_axis',(0.,0.,-1.));
#30195=DIRECTION('center_axis',(0.,1.,0.));
#30196=DIRECTION('ref_axis',(0.,0.,1.));
#30197=DIRECTION('center_axis',(0.,1.,0.));
#30198=DIRECTION('ref_axis',(1.,0.,0.));
#30199=DIRECTION('',(0.,-1.,0.));
#30200=DIRECTION('center_axis',(0.,1.,0.));
#30201=DIRECTION('ref_axis',(0.,0.,1.));
#36027=CARTESIAN_POINT('',(0.,0.,0.));
#36028=CARTESIAN_POINT('Origin',(-4.52295818048544,37.28,-5.95914969938874));
#36029=CARTESIAN_POINT('',(-9.89112836854344,37.2481324154382,-12.6120676561534));
#36030=CARTESIAN_POINT('',(-10.0197923273836,37.03,-13.1160858846074));
#36031=CARTESIAN_POINT('',(-9.14322579460993,38.5161005118286,-9.68229203158593));
#36032=CARTESIAN_POINT('',(-7.86882139091927,37.03,-10.47057043093));
#36033=CARTESIAN_POINT('',(-4.32898314662489,37.03,-6.11686363738662));
#36034=CARTESIAN_POINT('',(-8.24055326038937,37.53,-10.1351955192135));
#36035=CARTESIAN_POINT('',(-8.10824010307448,37.3520314584495,-10.2545678870352));
#36036=CARTESIAN_POINT('',(-9.43386642869197,37.53,-11.6028715227817));
#36037=CARTESIAN_POINT('',(-4.71693321434598,37.53,-5.80143576139086));
#36038=CARTESIAN_POINT('',(-9.69653989065522,37.4321844925501,-12.0809901437375));
#36039=CARTESIAN_POINT('',(-7.88714667228405,38.1059743550985,-8.78752995225675));
#36040=CARTESIAN_POINT('',(-8.64161158510598,38.4299914950389,-9.20184382239172));
#36041=CARTESIAN_POINT('Origin',(0.,37.03,0.));
#36042=CARTESIAN_POINT('',(-9.23658232924928,37.03,-9.23658232924928));
#36043=CARTESIAN_POINT('',(-9.23658232924928,37.03,-9.23658232924928));
#36044=CARTESIAN_POINT('',(-10.0358241714444,37.03,-13.1788877890042));
#36045=CARTESIAN_POINT('',(-9.89112836854344,37.03,-12.6120676561534));
#36046=CARTESIAN_POINT('',(-10.1356594341564,37.03,-13.7749103120746));
#36047=CARTESIAN_POINT('',(-10.0358241714444,37.03,-13.1788877890042));
#36048=CARTESIAN_POINT('',(-10.192780409838,37.03,-14.3959225765489));
#36049=CARTESIAN_POINT('',(-10.1356594341564,37.03,-13.7749103120746));
#36050=CARTESIAN_POINT('',(-10.208136822609,37.03,-15.0386712143394));
#36051=CARTESIAN_POINT('',(-10.192780409838,37.03,-14.3959225765489));
#36052=CARTESIAN_POINT('',(-10.1820769523934,37.03,-15.7003835976467));
#36053=CARTESIAN_POINT('',(-10.208136822609,37.03,-15.0386712143394));
#36054=CARTESIAN_POINT('',(-10.1146191541229,37.03,-16.3785524197668));
#36055=CARTESIAN_POINT('',(-10.1820769523934,37.03,-15.7003835976467));
#36056=CARTESIAN_POINT('',(-9.87089260802487,37.03,-16.5265840124582));
#36057=CARTESIAN_POINT('',(-10.1146191541229,37.03,-16.3785524197668));
#36058=CARTESIAN_POINT('',(-9.62500000000001,37.03,-16.6709890228504));
#36059=CARTESIAN_POINT('',(-9.87089260802487,37.03,-16.5265840124582));
#36060=CARTESIAN_POINT('',(-9.37699528855417,37.03,-16.8117357628067));
#36061=CARTESIAN_POINT('',(-9.62500000000001,37.03,-16.6709890228504));
#36062=CARTESIAN_POINT('',(-9.12693289567173,37.03,-16.9487933469585));
#36063=CARTESIAN_POINT('',(-9.37699528855417,37.03,-16.8117357628067));
#36064=CARTESIAN_POINT('',(-8.50589256852587,37.03,-16.6681291028841));
#36065=CARTESIAN_POINT('',(-9.12693289567173,37.03,-16.9487933469585));
#36066=CARTESIAN_POINT('',(-7.91980289947518,37.03,-16.3598414208564));
#36067=CARTESIAN_POINT('',(-8.50589256852587,37.03,-16.6681291028841));
#36068=CARTESIAN_POINT('',(-7.37084445728623,37.03,-16.0251680583905));
#36069=CARTESIAN_POINT('',(-7.91980289947518,37.03,-16.3598414208564));
#36070=CARTESIAN_POINT('',(-6.86159254803069,37.03,-15.6651937101241));
#36071=CARTESIAN_POINT('',(-7.37084445728623,37.03,-16.0251680583905));
#36072=CARTESIAN_POINT('',(-6.39533953317998,37.03,-15.2807225748869));
#36073=CARTESIAN_POINT('',(-6.86159254803069,37.03,-15.6651937101241));
#36074=CARTESIAN_POINT('',(-6.34896741059669,37.03,-15.2354376384622));
#36075=CARTESIAN_POINT('',(-6.39533953317998,37.03,-15.2807225748869));
#36076=CARTESIAN_POINT('',(-5.13336928983992,37.03,-12.0498844378435));
#36077=CARTESIAN_POINT('',(-2.79567366841787,37.03,-5.92380243612285));
#36078=CARTESIAN_POINT('',(-3.38082377665168,37.03,-12.617406105901));
#36079=CARTESIAN_POINT('',(-4.65706016176646,37.03,-12.2041262243426));
#36080=CARTESIAN_POINT('',(-1.57931400691349,37.03,-13.0021906807592));
#36081=CARTESIAN_POINT('',(-3.38082377665168,37.03,-12.617406105901));
#36082=CARTESIAN_POINT('',(-2.11935175385489,37.03,-16.3687597379803));
#36083=CARTESIAN_POINT('',(-0.690577558838534,37.03,-7.46185087477454));
#36084=CARTESIAN_POINT('',(-2.10183478588267,37.03,-16.4311637046244));
#36085=CARTESIAN_POINT('',(-2.25993461117485,37.03,-15.8679351687486));
#36086=CARTESIAN_POINT('',(-1.8902833980495,37.03,-16.997251982187));
#36087=CARTESIAN_POINT('',(-2.10183478588267,37.03,-16.4311637046244));
#36088=CARTESIAN_POINT('',(-1.62924548184168,37.03,-17.5636248671243));
#36089=CARTESIAN_POINT('',(-1.8902833980495,37.03,-16.997251982187));
#36090=CARTESIAN_POINT('',(-1.32117020651705,37.03,-18.1279397220842));
#36091=CARTESIAN_POINT('',(-1.62924548184168,37.03,-17.5636248671243));
#36092=CARTESIAN_POINT('',(-0.967745505237382,37.03,-18.6879695209193));
#36093=CARTESIAN_POINT('',(-1.32117020651705,37.03,-18.1279397220842));
#36094=CARTESIAN_POINT('',(-0.57024092719168,37.03,-19.2415520497946));
#36095=CARTESIAN_POINT('',(-0.967745505237382,37.03,-18.6879695209193));
#36096=CARTESIAN_POINT('',(-0.285151750348432,37.03,-19.247887896579));
#36097=CARTESIAN_POINT('',(-0.57024092719168,37.03,-19.2415520497946));
#36098=CARTESIAN_POINT('',(1.17872254417933E-15,37.03,-19.25));
#36099=CARTESIAN_POINT('',(-0.285151750348432,37.03,-19.247887896579));
#36100=CARTESIAN_POINT('',(0.285151750348434,37.03,-19.247887896579));
#36101=CARTESIAN_POINT('',(1.17872254417933E-15,37.03,-19.25));
#36102=CARTESIAN_POINT('',(0.570240927191682,37.03,-19.2415520497946));
#36103=CARTESIAN_POINT('',(0.285151750348434,37.03,-19.247887896579));
#36104=CARTESIAN_POINT('',(0.967745505237385,37.03,-18.6879695209193));
#36105=CARTESIAN_POINT('',(0.570240927191682,37.03,-19.2415520497946));
#36106=CARTESIAN_POINT('',(1.32117020651705,37.03,-18.1279397220842));
#36107=CARTESIAN_POINT('',(0.967745505237385,37.03,-18.6879695209193));
#36108=CARTESIAN_POINT('',(1.62924548184168,37.03,-17.5636248671243));
#36109=CARTESIAN_POINT('',(1.32117020651705,37.03,-18.1279397220842));
#36110=CARTESIAN_POINT('',(1.8902833980495,37.03,-16.997251982187));
#36111=CARTESIAN_POINT('',(1.62924548184168,37.03,-17.5636248671243));
#36112=CARTESIAN_POINT('',(2.10183478588268,37.03,-16.4311637046244));
#36113=CARTESIAN_POINT('',(1.8902833980495,37.03,-16.997251982187));
#36114=CARTESIAN_POINT('',(2.11935175385489,37.03,-16.3687597379803));
#36115=CARTESIAN_POINT('',(2.10183478588268,37.03,-16.4311637046244));
#36116=CARTESIAN_POINT('',(1.57931400691349,37.03,-13.0021906807592));
#36117=CARTESIAN_POINT('',(0.540776800520309,37.03,-6.52800023089146));
#36118=CARTESIAN_POINT('',(3.38082377665168,37.03,-12.617406105901));
#36119=CARTESIAN_POINT('',(2.0689307051291,37.03,-12.8976134221558));
#36120=CARTESIAN_POINT('',(5.13336928983992,37.03,-12.0498844378435));
#36121=CARTESIAN_POINT('',(3.38082377665168,37.03,-12.617406105901));
#36122=CARTESIAN_POINT('',(6.34896741059669,37.03,-15.2354376384623));
#36123=CARTESIAN_POINT('',(3.13286772814966,37.03,-6.80744119622516));
#36124=CARTESIAN_POINT('',(6.39533953317997,37.03,-15.2807225748869));
#36125=CARTESIAN_POINT('',(5.97680680020517,37.03,-14.8720022673282));
#36126=CARTESIAN_POINT('',(6.86159254803069,37.03,-15.6651937101241));
#36127=CARTESIAN_POINT('',(6.39533953317997,37.03,-15.2807225748869));
#36128=CARTESIAN_POINT('',(7.37084445728622,37.03,-16.0251680583905));
#36129=CARTESIAN_POINT('',(6.86159254803069,37.03,-15.6651937101241));
#36130=CARTESIAN_POINT('',(7.91980289947518,37.03,-16.3598414208564));
#36131=CARTESIAN_POINT('',(7.37084445728622,37.03,-16.0251680583905));
#36132=CARTESIAN_POINT('',(8.50589256852587,37.03,-16.6681291028841));
#36133=CARTESIAN_POINT('',(7.91980289947518,37.03,-16.3598414208564));
#36134=CARTESIAN_POINT('',(9.12693289567173,37.03,-16.9487933469585));
#36135=CARTESIAN_POINT('',(8.50589256852587,37.03,-16.6681291028841));
#36136=CARTESIAN_POINT('',(9.37699528855417,37.03,-16.8117357628067));
#36137=CARTESIAN_POINT('',(9.12693289567173,37.03,-16.9487933469585));
#36138=CARTESIAN_POINT('',(9.625,37.03,-16.6709890228504));
#36139=CARTESIAN_POINT('',(9.37699528855417,37.03,-16.8117357628067));
#36140=CARTESIAN_POINT('',(9.87089260802485,37.03,-16.5265840124582));
#36141=CARTESIAN_POINT('',(9.625,37.03,-16.6709890228504));
#36142=CARTESIAN_POINT('',(10.1146191541229,37.03,-16.3785524197668));
#36143=CARTESIAN_POINT('',(9.87089260802485,37.03,-16.5265840124582));
#36144=CARTESIAN_POINT('',(10.1820769523934,37.03,-15.7003835976467));
#36145=CARTESIAN_POINT('',(10.1146191541229,37.03,-16.3785524197668));
#36146=CARTESIAN_POINT('',(10.208136822609,37.03,-15.0386712143394));
#36147=CARTESIAN_POINT('',(10.1820769523934,37.03,-15.7003835976467));
#36148=CARTESIAN_POINT('',(10.192780409838,37.03,-14.3959225765489));
#36149=CARTESIAN_POINT('',(10.208136822609,37.03,-15.0386712143394));
#36150=CARTESIAN_POINT('',(10.1356594341564,37.03,-13.7749103120746));
#36151=CARTESIAN_POINT('',(10.192780409838,37.03,-14.3959225765489));
#36152=CARTESIAN_POINT('',(10.0358241714444,37.03,-13.1788877890042));
#36153=CARTESIAN_POINT('',(10.1356594341564,37.03,-13.7749103120746));
#36154=CARTESIAN_POINT('',(10.0197923273836,37.03,-13.1160858846074));
#36155=CARTESIAN_POINT('',(10.0358241714444,37.03,-13.1788877890042));
#36156=CARTESIAN_POINT('',(7.86882139091926,37.03,-10.47057043093));
#36157=CARTESIAN_POINT('',(3.73232656247359,37.03,-5.38302563560254));
#36158=CARTESIAN_POINT('',(9.23658232924928,37.03,-9.23658232924928));
#36159=CARTESIAN_POINT('',(8.24055326038937,37.03,-10.1351955192135));
#36160=CARTESIAN_POINT('',(10.47057043093,37.03,-7.86882139091926));
#36161=CARTESIAN_POINT('',(9.23658232924928,37.03,-9.23658232924928));
#36162=CARTESIAN_POINT('',(13.1160858846074,37.03,-10.0197923273836));
#36163=CARTESIAN_POINT('',(6.11686363738662,37.03,-4.32898314662489));
#36164=CARTESIAN_POINT('',(13.1788877890042,37.03,-10.0358241714444));
#36165=CARTESIAN_POINT('',(12.6120676561534,37.03,-9.89112836854343));
#36166=CARTESIAN_POINT('',(13.7749103120746,37.03,-10.1356594341564));
#36167=CARTESIAN_POINT('',(13.1788877890042,37.03,-10.0358241714444));
#36168=CARTESIAN_POINT('',(14.3959225765489,37.03,-10.192780409838));
#36169=CARTESIAN_POINT('',(13.7749103120746,37.03,-10.1356594341564));
#36170=CARTESIAN_POINT('',(15.0386712143394,37.03,-10.208136822609));
#36171=CARTESIAN_POINT('',(14.3959225765489,37.03,-10.192780409838));
#36172=CARTESIAN_POINT('',(15.7003835976467,37.03,-10.1820769523934));
#36173=CARTESIAN_POINT('',(15.0386712143394,37.03,-10.208136822609));
#36174=CARTESIAN_POINT('',(16.3785524197668,37.03,-10.1146191541229));
#36175=CARTESIAN_POINT('',(15.7003835976467,37.03,-10.1820769523934));
#36176=CARTESIAN_POINT('',(16.5265840124582,37.03,-9.87089260802485));
#36177=CARTESIAN_POINT('',(16.3785524197668,37.03,-10.1146191541229));
#36178=CARTESIAN_POINT('',(16.6709890228504,37.03,-9.625));
#36179=CARTESIAN_POINT('',(16.5265840124582,37.03,-9.87089260802485));
#36180=CARTESIAN_POINT('',(16.8117357628067,37.03,-9.37699528855417));
#36181=CARTESIAN_POINT('',(16.6709890228504,37.03,-9.625));
#36182=CARTESIAN_POINT('',(16.9487933469585,37.03,-9.12693289567172));
#36183=CARTESIAN_POINT('',(16.8117357628067,37.03,-9.37699528855417));
#36184=CARTESIAN_POINT('',(16.6681291028841,37.03,-8.50589256852586));
#36185=CARTESIAN_POINT('',(16.9487933469585,37.03,-9.12693289567172));
#36186=CARTESIAN_POINT('',(16.3598414208564,37.03,-7.91980289947517));
#36187=CARTESIAN_POINT('',(16.6681291028841,37.03,-8.50589256852586));
#36188=CARTESIAN_POINT('',(16.0251680583905,37.03,-7.37084445728621));
#36189=CARTESIAN_POINT('',(16.3598414208564,37.03,-7.91980289947517));
#36190=CARTESIAN_POINT('',(15.6651937101241,37.03,-6.86159254803069));
#36191=CARTESIAN_POINT('',(16.0251680583905,37.03,-7.37084445728621));
#36192=CARTESIAN_POINT('',(15.2807225748869,37.03,-6.39533953317997));
#36193=CARTESIAN_POINT('',(15.6651937101241,37.03,-6.86159254803069));
#36194=CARTESIAN_POINT('',(15.2354376384623,37.03,-6.34896741059669));
#36195=CARTESIAN_POINT('',(15.2807225748869,37.03,-6.39533953317997));
#36196=CARTESIAN_POINT('',(12.0498844378435,37.03,-5.13336928983991));
#36197=CARTESIAN_POINT('',(5.92380243612284,37.03,-2.79567366841787));
#36198=CARTESIAN_POINT('',(12.617406105901,37.03,-3.38082377665168));
#36199=CARTESIAN_POINT('',(12.2041262243426,37.03,-4.65706016176646));
#36200=CARTESIAN_POINT('',(13.0021906807592,37.03,-1.57931400691349));
#36201=CARTESIAN_POINT('',(12.617406105901,37.03,-3.38082377665168));
#36202=CARTESIAN_POINT('',(16.3687597379803,37.03,-2.11935175385489));
#36203=CARTESIAN_POINT('',(7.46185087477454,37.03,-0.690577558838536));
#36204=CARTESIAN_POINT('',(16.4311637046244,37.03,-2.10183478588267));
#36205=CARTESIAN_POINT('',(15.8679351687486,37.03,-2.25993461117485));
#36206=CARTESIAN_POINT('',(16.997251982187,37.03,-1.8902833980495));
#36207=CARTESIAN_POINT('',(16.4311637046244,37.03,-2.10183478588267));
#36208=CARTESIAN_POINT('',(17.5636248671243,37.03,-1.62924548184168));
#36209=CARTESIAN_POINT('',(16.997251982187,37.03,-1.8902833980495));
#36210=CARTESIAN_POINT('',(18.1279397220842,37.03,-1.32117020651705));
#36211=CARTESIAN_POINT('',(17.5636248671243,37.03,-1.62924548184168));
#36212=CARTESIAN_POINT('',(18.6879695209193,37.03,-0.967745505237384));
#36213=CARTESIAN_POINT('',(18.1279397220842,37.03,-1.32117020651705));
#36214=CARTESIAN_POINT('',(19.2415520497946,37.03,-0.570240927191682));
#36215=CARTESIAN_POINT('',(18.6879695209193,37.03,-0.967745505237384));
#36216=CARTESIAN_POINT('',(19.247887896579,37.03,-0.285151750348434));
#36217=CARTESIAN_POINT('',(19.2415520497946,37.03,-0.570240927191682));
#36218=CARTESIAN_POINT('',(19.25,37.03,0.));
#36219=CARTESIAN_POINT('',(19.247887896579,37.03,-0.285151750348434));
#36220=CARTESIAN_POINT('',(19.247887896579,37.03,0.285151750348434));
#36221=CARTESIAN_POINT('',(19.25,37.03,0.));
#36222=CARTESIAN_POINT('',(19.2415520497946,37.03,0.570240927191682));
#36223=CARTESIAN_POINT('',(19.247887896579,37.03,0.285151750348434));
#36224=CARTESIAN_POINT('',(18.6879695209193,37.03,0.967745505237384));
#36225=CARTESIAN_POINT('',(19.2415520497946,37.03,0.570240927191682));
#36226=CARTESIAN_POINT('',(18.1279397220842,37.03,1.32117020651705));
#36227=CARTESIAN_POINT('',(18.6879695209193,37.03,0.967745505237384));
#36228=CARTESIAN_POINT('',(17.5636248671243,37.03,1.62924548184168));
#36229=CARTESIAN_POINT('',(18.1279397220842,37.03,1.32117020651705));
#36230=CARTESIAN_POINT('',(16.997251982187,37.03,1.8902833980495));
#36231=CARTESIAN_POINT('',(17.5636248671243,37.03,1.62924548184168));
#36232=CARTESIAN_POINT('',(16.4311637046244,37.03,2.10183478588267));
#36233=CARTESIAN_POINT('',(16.997251982187,37.03,1.8902833980495));
#36234=CARTESIAN_POINT('',(16.3687597379803,37.03,2.11935175385489));
#36235=CARTESIAN_POINT('',(16.4311637046244,37.03,2.10183478588267));
#36236=CARTESIAN_POINT('',(13.0021906807592,37.03,1.57931400691349));
#36237=CARTESIAN_POINT('',(6.52800023089146,37.03,0.540776800520309));
#36238=CARTESIAN_POINT('',(12.617406105901,37.03,3.38082377665168));
#36239=CARTESIAN_POINT('',(12.8976134221558,37.03,2.0689307051291));
#36240=CARTESIAN_POINT('',(12.0498844378435,37.03,5.13336928983991));
#36241=CARTESIAN_POINT('',(12.617406105901,37.03,3.38082377665168));
#36242=CARTESIAN_POINT('',(15.2354376384623,37.03,6.34896741059669));
#36243=CARTESIAN_POINT('',(6.80744119622516,37.03,3.13286772814966));
#36244=CARTESIAN_POINT('',(15.2807225748869,37.03,6.39533953317997));
#36245=CARTESIAN_POINT('',(14.8720022673282,37.03,5.97680680020517));
#36246=CARTESIAN_POINT('',(15.6651937101241,37.03,6.86159254803069));
#36247=CARTESIAN_POINT('',(15.2807225748869,37.03,6.39533953317997));
#36248=CARTESIAN_POINT('',(16.0251680583905,37.03,7.37084445728621));
#36249=CARTESIAN_POINT('',(15.6651937101241,37.03,6.86159254803069));
#36250=CARTESIAN_POINT('',(16.3598414208564,37.03,7.91980289947517));
#36251=CARTESIAN_POINT('',(16.0251680583905,37.03,7.37084445728621));
#36252=CARTESIAN_POINT('',(16.6681291028841,37.03,8.50589256852586));
#36253=CARTESIAN_POINT('',(16.3598414208564,37.03,7.91980289947517));
#36254=CARTESIAN_POINT('',(16.9487933469585,37.03,9.12693289567172));
#36255=CARTESIAN_POINT('',(16.6681291028841,37.03,8.50589256852586));
#36256=CARTESIAN_POINT('',(16.8117357628067,37.03,9.37699528855417));
#36257=CARTESIAN_POINT('',(16.9487933469585,37.03,9.12693289567172));
#36258=CARTESIAN_POINT('',(16.6709890228504,37.03,9.625));
#36259=CARTESIAN_POINT('',(16.8117357628067,37.03,9.37699528855417));
#36260=CARTESIAN_POINT('',(16.5265840124582,37.03,9.87089260802485));
#36261=CARTESIAN_POINT('',(16.6709890228504,37.03,9.625));
#36262=CARTESIAN_POINT('',(16.3785524197668,37.03,10.1146191541229));
#36263=CARTESIAN_POINT('',(16.5265840124582,37.03,9.87089260802485));
#36264=CARTESIAN_POINT('',(15.7003835976467,37.03,10.1820769523934));
#36265=CARTESIAN_POINT('',(16.3785524197668,37.03,10.1146191541229));
#36266=CARTESIAN_POINT('',(15.0386712143394,37.03,10.208136822609));
#36267=CARTESIAN_POINT('',(15.7003835976467,37.03,10.1820769523934));
#36268=CARTESIAN_POINT('',(14.3959225765489,37.03,10.192780409838));
#36269=CARTESIAN_POINT('',(15.0386712143394,37.03,10.208136822609));
#36270=CARTESIAN_POINT('',(13.7749103120746,37.03,10.1356594341564));
#36271=CARTESIAN_POINT('',(14.3959225765489,37.03,10.192780409838));
#36272=CARTESIAN_POINT('',(13.1788877890042,37.03,10.0358241714444));
#36273=CARTESIAN_POINT('',(13.7749103120746,37.03,10.1356594341564));
#36274=CARTESIAN_POINT('',(13.1160858846074,37.03,10.0197923273836));
#36275=CARTESIAN_POINT('',(13.1788877890042,37.03,10.0358241714444));
#36276=CARTESIAN_POINT('',(10.47057043093,37.03,7.86882139091926));
#36277=CARTESIAN_POINT('',(5.38302563560253,37.03,3.73232656247359));
#36278=CARTESIAN_POINT('',(9.23658232924928,37.03,9.23658232924928));
#36279=CARTESIAN_POINT('',(10.1351955192135,37.03,8.24055326038936));
#36280=CARTESIAN_POINT('',(7.86882139091926,37.03,10.47057043093));
#36281=CARTESIAN_POINT('',(9.23658232924928,37.03,9.23658232924928));
#36282=CARTESIAN_POINT('',(10.0197923273836,37.03,13.1160858846074));
#36283=CARTESIAN_POINT('',(4.32898314662489,37.03,6.11686363738663));
#36284=CARTESIAN_POINT('',(10.0358241714444,37.03,13.1788877890042));
#36285=CARTESIAN_POINT('',(9.89112836854343,37.03,12.6120676561534));
#36286=CARTESIAN_POINT('',(10.1356594341564,37.03,13.7749103120746));
#36287=CARTESIAN_POINT('',(10.0358241714444,37.03,13.1788877890042));
#36288=CARTESIAN_POINT('',(10.192780409838,37.03,14.3959225765489));
#36289=CARTESIAN_POINT('',(10.1356594341564,37.03,13.7749103120746));
#36290=CARTESIAN_POINT('',(10.208136822609,37.03,15.0386712143394));
#36291=CARTESIAN_POINT('',(10.192780409838,37.03,14.3959225765489));
#36292=CARTESIAN_POINT('',(10.1820769523934,37.03,15.7003835976467));
#36293=CARTESIAN_POINT('',(10.208136822609,37.03,15.0386712143394));
#36294=CARTESIAN_POINT('',(10.1146191541229,37.03,16.3785524197668));
#36295=CARTESIAN_POINT('',(10.1820769523934,37.03,15.7003835976467));
#36296=CARTESIAN_POINT('',(9.87089260802485,37.03,16.5265840124582));
#36297=CARTESIAN_POINT('',(10.1146191541229,37.03,16.3785524197668));
#36298=CARTESIAN_POINT('',(9.625,37.03,16.6709890228504));
#36299=CARTESIAN_POINT('',(9.87089260802485,37.03,16.5265840124582));
#36300=CARTESIAN_POINT('',(9.37699528855417,37.03,16.8117357628067));
#36301=CARTESIAN_POINT('',(9.625,37.03,16.6709890228504));
#36302=CARTESIAN_POINT('',(9.12693289567173,37.03,16.9487933469585));
#36303=CARTESIAN_POINT('',(9.37699528855417,37.03,16.8117357628067));
#36304=CARTESIAN_POINT('',(8.50589256852587,37.03,16.6681291028841));
#36305=CARTESIAN_POINT('',(9.12693289567173,37.03,16.9487933469585));
#36306=CARTESIAN_POINT('',(7.91980289947518,37.03,16.3598414208564));
#36307=CARTESIAN_POINT('',(8.50589256852587,37.03,16.6681291028841));
#36308=CARTESIAN_POINT('',(7.37084445728622,37.03,16.0251680583905));
#36309=CARTESIAN_POINT('',(7.91980289947518,37.03,16.3598414208564));
#36310=CARTESIAN_POINT('',(6.86159254803069,37.03,15.6651937101241));
#36311=CARTESIAN_POINT('',(7.37084445728622,37.03,16.0251680583905));
#36312=CARTESIAN_POINT('',(6.39533953317997,37.03,15.2807225748869));
#36313=CARTESIAN_POINT('',(6.86159254803069,37.03,15.6651937101241));
#36314=CARTESIAN_POINT('',(6.34896741059669,37.03,15.2354376384623));
#36315=CARTESIAN_POINT('',(6.39533953317997,37.03,15.2807225748869));
#36316=CARTESIAN_POINT('',(5.13336928983992,37.03,12.0498844378435));
#36317=CARTESIAN_POINT('',(2.79567366841787,37.03,5.92380243612285));
#36318=CARTESIAN_POINT('',(3.38082377665168,37.03,12.617406105901));
#36319=CARTESIAN_POINT('',(4.65706016176646,37.03,12.2041262243426));
#36320=CARTESIAN_POINT('',(1.57931400691349,37.03,13.0021906807592));
#36321=CARTESIAN_POINT('',(3.38082377665168,37.03,12.617406105901));
#36322=CARTESIAN_POINT('',(2.11935175385489,37.03,16.3687597379803));
#36323=CARTESIAN_POINT('',(0.690577558838536,37.03,7.46185087477454));
#36324=CARTESIAN_POINT('',(2.10183478588268,37.03,16.4311637046244));
#36325=CARTESIAN_POINT('',(2.25993461117485,37.03,15.8679351687486));
#36326=CARTESIAN_POINT('',(1.8902833980495,37.03,16.997251982187));
#36327=CARTESIAN_POINT('',(2.10183478588268,37.03,16.4311637046244));
#36328=CARTESIAN_POINT('',(1.62924548184168,37.03,17.5636248671243));
#36329=CARTESIAN_POINT('',(1.8902833980495,37.03,16.997251982187));
#36330=CARTESIAN_POINT('',(1.32117020651705,37.03,18.1279397220842));
#36331=CARTESIAN_POINT('',(1.62924548184168,37.03,17.5636248671243));
#36332=CARTESIAN_POINT('',(0.967745505237385,37.03,18.6879695209193));
#36333=CARTESIAN_POINT('',(1.32117020651705,37.03,18.1279397220842));
#36334=CARTESIAN_POINT('',(0.570240927191682,37.03,19.2415520497946));
#36335=CARTESIAN_POINT('',(0.967745505237385,37.03,18.6879695209193));
#36336=CARTESIAN_POINT('',(0.285151750348434,37.03,19.247887896579));
#36337=CARTESIAN_POINT('',(0.570240927191682,37.03,19.2415520497946));
#36338=CARTESIAN_POINT('',(1.17872254417933E-15,37.03,19.25));
#36339=CARTESIAN_POINT('',(0.285151750348434,37.03,19.247887896579));
#36340=CARTESIAN_POINT('',(-0.285151750348432,37.03,19.247887896579));
#36341=CARTESIAN_POINT('',(1.17872254417933E-15,37.03,19.25));
#36342=CARTESIAN_POINT('',(-0.57024092719168,37.03,19.2415520497946));
#36343=CARTESIAN_POINT('',(-0.285151750348432,37.03,19.247887896579));
#36344=CARTESIAN_POINT('',(-0.967745505237382,37.03,18.6879695209193));
#36345=CARTESIAN_POINT('',(-0.57024092719168,37.03,19.2415520497946));
#36346=CARTESIAN_POINT('',(-1.32117020651705,37.03,18.1279397220842));
#36347=CARTESIAN_POINT('',(-0.967745505237382,37.03,18.6879695209193));
#36348=CARTESIAN_POINT('',(-1.62924548184168,37.03,17.5636248671243));
#36349=CARTESIAN_POINT('',(-1.32117020651705,37.03,18.1279397220842));
#36350=CARTESIAN_POINT('',(-1.8902833980495,37.03,16.997251982187));
#36351=CARTESIAN_POINT('',(-1.62924548184168,37.03,17.5636248671243));
#36352=CARTESIAN_POINT('',(-2.10183478588267,37.03,16.4311637046244));
#36353=CARTESIAN_POINT('',(-1.8902833980495,37.03,16.997251982187));
#36354=CARTESIAN_POINT('',(-2.11935175385489,37.03,16.3687597379803));
#36355=CARTESIAN_POINT('',(-2.10183478588267,37.03,16.4311637046244));
#36356=CARTESIAN_POINT('',(-1.57931400691349,37.03,13.0021906807592));
#36357=CARTESIAN_POINT('',(-0.540776800520307,37.03,6.52800023089147));
#36358=CARTESIAN_POINT('',(-3.38082377665168,37.03,12.617406105901));
#36359=CARTESIAN_POINT('',(-2.0689307051291,37.03,12.8976134221558));
#36360=CARTESIAN_POINT('',(-5.13336928983991,37.03,12.0498844378435));
#36361=CARTESIAN_POINT('',(-3.38082377665168,37.03,12.617406105901));
#36362=CARTESIAN_POINT('',(-6.34896741059669,37.03,15.2354376384623));
#36363=CARTESIAN_POINT('',(-3.13286772814965,37.03,6.80744119622516));
#36364=CARTESIAN_POINT('',(-6.39533953317997,37.03,15.2807225748869));
#36365=CARTESIAN_POINT('',(-5.97680680020517,37.03,14.8720022673282));
#36366=CARTESIAN_POINT('',(-6.86159254803068,37.03,15.6651937101241));
#36367=CARTESIAN_POINT('',(-6.39533953317997,37.03,15.2807225748869));
#36368=CARTESIAN_POINT('',(-7.37084445728621,37.03,16.0251680583905));
#36369=CARTESIAN_POINT('',(-6.86159254803068,37.03,15.6651937101241));
#36370=CARTESIAN_POINT('',(-7.91980289947517,37.03,16.3598414208564));
#36371=CARTESIAN_POINT('',(-7.37084445728621,37.03,16.0251680583905));
#36372=CARTESIAN_POINT('',(-8.50589256852586,37.03,16.6681291028841));
#36373=CARTESIAN_POINT('',(-7.91980289947517,37.03,16.3598414208564));
#36374=CARTESIAN_POINT('',(-9.12693289567172,37.03,16.9487933469585));
#36375=CARTESIAN_POINT('',(-8.50589256852586,37.03,16.6681291028841));
#36376=CARTESIAN_POINT('',(-9.37699528855417,37.03,16.8117357628067));
#36377=CARTESIAN_POINT('',(-9.12693289567172,37.03,16.9487933469585));
#36378=CARTESIAN_POINT('',(-9.625,37.03,16.6709890228504));
#36379=CARTESIAN_POINT('',(-9.37699528855417,37.03,16.8117357628067));
#36380=CARTESIAN_POINT('',(-9.87089260802485,37.03,16.5265840124582));
#36381=CARTESIAN_POINT('',(-9.625,37.03,16.6709890228504));
#36382=CARTESIAN_POINT('',(-10.1146191541229,37.03,16.3785524197668));
#36383=CARTESIAN_POINT('',(-9.87089260802485,37.03,16.5265840124582));
#36384=CARTESIAN_POINT('',(-10.1820769523934,37.03,15.7003835976467));
#36385=CARTESIAN_POINT('',(-10.1146191541229,37.03,16.3785524197668));
#36386=CARTESIAN_POINT('',(-10.208136822609,37.03,15.0386712143394));
#36387=CARTESIAN_POINT('',(-10.1820769523934,37.03,15.7003835976467));
#36388=CARTESIAN_POINT('',(-10.192780409838,37.03,14.3959225765489));
#36389=CARTESIAN_POINT('',(-10.208136822609,37.03,15.0386712143394));
#36390=CARTESIAN_POINT('',(-10.1356594341564,37.03,13.7749103120746));
#36391=CARTESIAN_POINT('',(-10.192780409838,37.03,14.3959225765489));
#36392=CARTESIAN_POINT('',(-10.0358241714444,37.03,13.1788877890042));
#36393=CARTESIAN_POINT('',(-10.1356594341564,37.03,13.7749103120746));
#36394=CARTESIAN_POINT('',(-10.0197923273836,37.03,13.1160858846074));
#36395=CARTESIAN_POINT('',(-10.0358241714444,37.03,13.1788877890042));
#36396=CARTESIAN_POINT('',(-7.86882139091926,37.03,10.47057043093));
#36397=CARTESIAN_POINT('',(-3.73232656247359,37.03,5.38302563560253));
#36398=CARTESIAN_POINT('',(-9.23658232924928,37.03,9.23658232924928));
#36399=CARTESIAN_POINT('',(-8.24055326038936,37.03,10.1351955192135));
#36400=CARTESIAN_POINT('',(-10.47057043093,37.03,7.86882139091926));
#36401=CARTESIAN_POINT('',(-9.23658232924928,37.03,9.23658232924928));
#36402=CARTESIAN_POINT('',(-13.1160858846074,37.03,10.0197923273836));
#36403=CARTESIAN_POINT('',(-6.11686363738663,37.03,4.32898314662489));
#36404=CARTESIAN_POINT('',(-13.1788877890042,37.03,10.0358241714444));
#36405=CARTESIAN_POINT('',(-12.6120676561534,37.03,9.89112836854343));
#36406=CARTESIAN_POINT('',(-13.7749103120746,37.03,10.1356594341564));
#36407=CARTESIAN_POINT('',(-13.1788877890042,37.03,10.0358241714444));
#36408=CARTESIAN_POINT('',(-14.3959225765489,37.03,10.192780409838));
#36409=CARTESIAN_POINT('',(-13.7749103120746,37.03,10.1356594341564));
#36410=CARTESIAN_POINT('',(-15.0386712143394,37.03,10.208136822609));
#36411=CARTESIAN_POINT('',(-14.3959225765489,37.03,10.192780409838));
#36412=CARTESIAN_POINT('',(-15.7003835976467,37.03,10.1820769523934));
#36413=CARTESIAN_POINT('',(-15.0386712143394,37.03,10.208136822609));
#36414=CARTESIAN_POINT('',(-16.3785524197668,37.03,10.1146191541229));
#36415=CARTESIAN_POINT('',(-15.7003835976467,37.03,10.1820769523934));
#36416=CARTESIAN_POINT('',(-16.5265840124582,37.03,9.87089260802485));
#36417=CARTESIAN_POINT('',(-16.3785524197668,37.03,10.1146191541229));
#36418=CARTESIAN_POINT('',(-16.6709890228504,37.03,9.625));
#36419=CARTESIAN_POINT('',(-16.5265840124582,37.03,9.87089260802485));
#36420=CARTESIAN_POINT('',(-16.8117357628067,37.03,9.37699528855417));
#36421=CARTESIAN_POINT('',(-16.6709890228504,37.03,9.625));
#36422=CARTESIAN_POINT('',(-16.9487933469585,37.03,9.12693289567172));
#36423=CARTESIAN_POINT('',(-16.8117357628067,37.03,9.37699528855417));
#36424=CARTESIAN_POINT('',(-16.6681291028841,37.03,8.50589256852586));
#36425=CARTESIAN_POINT('',(-16.9487933469585,37.03,9.12693289567172));
#36426=CARTESIAN_POINT('',(-16.3598414208564,37.03,7.91980289947518));
#36427=CARTESIAN_POINT('',(-16.6681291028841,37.03,8.50589256852586));
#36428=CARTESIAN_POINT('',(-16.0251680583905,37.03,7.37084445728621));
#36429=CARTESIAN_POINT('',(-16.3598414208564,37.03,7.91980289947518));
#36430=CARTESIAN_POINT('',(-15.6651937101241,37.03,6.86159254803069));
#36431=CARTESIAN_POINT('',(-16.0251680583905,37.03,7.37084445728621));
#36432=CARTESIAN_POINT('',(-15.2807225748869,37.03,6.39533953317997));
#36433=CARTESIAN_POINT('',(-15.6651937101241,37.03,6.86159254803069));
#36434=CARTESIAN_POINT('',(-15.2354376384623,37.03,6.34896741059668));
#36435=CARTESIAN_POINT('',(-15.2807225748869,37.03,6.39533953317997));
#36436=CARTESIAN_POINT('',(-12.0498844378435,37.03,5.13336928983991));
#36437=CARTESIAN_POINT('',(-5.92380243612285,37.03,2.79567366841787));
#36438=CARTESIAN_POINT('',(-12.617406105901,37.03,3.38082377665168));
#36439=CARTESIAN_POINT('',(-12.2041262243426,37.03,4.65706016176645));
#36440=CARTESIAN_POINT('',(-13.0021906807592,37.03,1.57931400691349));
#36441=CARTESIAN_POINT('',(-12.617406105901,37.03,3.38082377665168));
#36442=CARTESIAN_POINT('',(-16.3687597379803,37.03,2.1193517538549));
#36443=CARTESIAN_POINT('',(-7.46185087477454,37.03,0.690577558838538));
#36444=CARTESIAN_POINT('',(-16.4311637046244,37.03,2.10183478588268));
#36445=CARTESIAN_POINT('',(-15.8679351687486,37.03,2.25993461117486));
#36446=CARTESIAN_POINT('',(-16.997251982187,37.03,1.8902833980495));
#36447=CARTESIAN_POINT('',(-16.4311637046244,37.03,2.10183478588268));
#36448=CARTESIAN_POINT('',(-17.5636248671243,37.03,1.62924548184169));
#36449=CARTESIAN_POINT('',(-16.997251982187,37.03,1.8902833980495));
#36450=CARTESIAN_POINT('',(-18.1279397220842,37.03,1.32117020651705));
#36451=CARTESIAN_POINT('',(-17.5636248671243,37.03,1.62924548184169));
#36452=CARTESIAN_POINT('',(-18.6879695209193,37.03,0.96774550523739));
#36453=CARTESIAN_POINT('',(-18.1279397220842,37.03,1.32117020651705));
#36454=CARTESIAN_POINT('',(-19.2415520497946,37.03,0.570240927191683));
#36455=CARTESIAN_POINT('',(-18.6879695209193,37.03,0.96774550523739));
#36456=CARTESIAN_POINT('',(-19.247887896579,37.03,0.285151750348435));
#36457=CARTESIAN_POINT('',(-19.2415520497946,37.03,0.570240927191683));
#36458=CARTESIAN_POINT('',(-19.25,37.03,2.35744508835865E-15));
#36459=CARTESIAN_POINT('',(-19.247887896579,37.03,0.285151750348435));
#36460=CARTESIAN_POINT('',(-19.247887896579,37.03,-0.285151750348431));
#36461=CARTESIAN_POINT('',(-19.25,37.03,2.35744508835865E-15));
#36462=CARTESIAN_POINT('',(-19.2415520497946,37.03,-0.570240927191679));
#36463=CARTESIAN_POINT('',(-19.247887896579,37.03,-0.285151750348431));
#36464=CARTESIAN_POINT('',(-18.6879695209193,37.03,-0.967745505237385));
#36465=CARTESIAN_POINT('',(-19.2415520497946,37.03,-0.570240927191679));
#36466=CARTESIAN_POINT('',(-18.1279397220842,37.03,-1.32117020651705));
#36467=CARTESIAN_POINT('',(-18.6879695209193,37.03,-0.967745505237385));
#36468=CARTESIAN_POINT('',(-17.5636248671243,37.03,-1.62924548184168));
#36469=CARTESIAN_POINT('',(-18.1279397220842,37.03,-1.32117020651705));
#36470=CARTESIAN_POINT('',(-16.997251982187,37.03,-1.89028339804949));
#36471=CARTESIAN_POINT('',(-17.5636248671243,37.03,-1.62924548184168));
#36472=CARTESIAN_POINT('',(-16.4311637046244,37.03,-2.10183478588267));
#36473=CARTESIAN_POINT('',(-16.997251982187,37.03,-1.89028339804949));
#36474=CARTESIAN_POINT('',(-16.3687597379803,37.03,-2.11935175385489));
#36475=CARTESIAN_POINT('',(-16.4311637046244,37.03,-2.10183478588267));
#36476=CARTESIAN_POINT('',(-13.0021906807592,37.03,-1.57931400691349));
#36477=CARTESIAN_POINT('',(-6.52800023089146,37.03,-0.540776800520311));
#36478=CARTESIAN_POINT('',(-12.617406105901,37.03,-3.38082377665168));
#36479=CARTESIAN_POINT('',(-12.8976134221558,37.03,-2.0689307051291));
#36480=CARTESIAN_POINT('',(-12.0498844378435,37.03,-5.13336928983991));
#36481=CARTESIAN_POINT('',(-12.617406105901,37.03,-3.38082377665168));
#36482=CARTESIAN_POINT('',(-15.2354376384623,37.03,-6.34896741059669));
#36483=CARTESIAN_POINT('',(-6.80744119622516,37.03,-3.13286772814966));
#36484=CARTESIAN_POINT('',(-15.2807225748869,37.03,-6.39533953317997));
#36485=CARTESIAN_POINT('',(-14.8720022673282,37.03,-5.97680680020517));
#36486=CARTESIAN_POINT('',(-15.6651937101241,37.03,-6.86159254803069));
#36487=CARTESIAN_POINT('',(-15.2807225748869,37.03,-6.39533953317997));
#36488=CARTESIAN_POINT('',(-16.0251680583905,37.03,-7.37084445728622));
#36489=CARTESIAN_POINT('',(-15.6651937101241,37.03,-6.86159254803069));
#36490=CARTESIAN_POINT('',(-16.3598414208564,37.03,-7.91980289947518));
#36491=CARTESIAN_POINT('',(-16.0251680583905,37.03,-7.37084445728622));
#36492=CARTESIAN_POINT('',(-16.6681291028841,37.03,-8.50589256852587));
#36493=CARTESIAN_POINT('',(-16.3598414208564,37.03,-7.91980289947518));
#36494=CARTESIAN_POINT('',(-16.9487933469585,37.03,-9.12693289567173));
#36495=CARTESIAN_POINT('',(-16.6681291028841,37.03,-8.50589256852587));
#36496=CARTESIAN_POINT('',(-16.8117357628067,37.03,-9.37699528855417));
#36497=CARTESIAN_POINT('',(-16.9487933469585,37.03,-9.12693289567173));
#36498=CARTESIAN_POINT('',(-16.6709890228504,37.03,-9.625));
#36499=CARTESIAN_POINT('',(-16.8117357628067,37.03,-9.37699528855417));
#36500=CARTESIAN_POINT('',(-16.5265840124582,37.03,-9.87089260802485));
#36501=CARTESIAN_POINT('',(-16.6709890228504,37.03,-9.625));
#36502=CARTESIAN_POINT('',(-16.3785524197668,37.03,-10.1146191541229));
#36503=CARTESIAN_POINT('',(-16.5265840124582,37.03,-9.87089260802485));
#36504=CARTESIAN_POINT('',(-15.7003835976467,37.03,-10.1820769523934));
#36505=CARTESIAN_POINT('',(-16.3785524197668,37.03,-10.1146191541229));
#36506=CARTESIAN_POINT('',(-15.0386712143394,37.03,-10.208136822609));
#36507=CARTESIAN_POINT('',(-15.7003835976467,37.03,-10.1820769523934));
#36508=CARTESIAN_POINT('',(-14.3959225765489,37.03,-10.192780409838));
#36509=CARTESIAN_POINT('',(-15.0386712143394,37.03,-10.208136822609));
#36510=CARTESIAN_POINT('',(-13.7749103120746,37.03,-10.1356594341564));
#36511=CARTESIAN_POINT('',(-14.3959225765489,37.03,-10.192780409838));
#36512=CARTESIAN_POINT('',(-13.1788877890042,37.03,-10.0358241714444));
#36513=CARTESIAN_POINT('',(-13.7749103120746,37.03,-10.1356594341564));
#36514=CARTESIAN_POINT('',(-13.1160858846074,37.03,-10.0197923273836));
#36515=CARTESIAN_POINT('',(-13.1788877890042,37.03,-10.0358241714444));
#36516=CARTESIAN_POINT('',(-10.47057043093,37.03,-7.86882139091926));
#36517=CARTESIAN_POINT('',(-5.38302563560254,37.03,-3.73232656247359));
#36518=CARTESIAN_POINT('',(-10.1351955192135,37.03,-8.24055326038937));
#36519=CARTESIAN_POINT('',(1.04094977927525E-15,37.03,-8.5));
#36520=CARTESIAN_POINT('Origin',(0.,37.03,0.));
#36521=CARTESIAN_POINT('Origin',(-10.0358241714444,37.03,-13.1788877890042));
#36522=CARTESIAN_POINT('',(-9.89112836854344,64.7518675845618,-12.6120676561534));
#36523=CARTESIAN_POINT('',(-9.89112836854344,37.03,-12.6120676561534));
#36524=CARTESIAN_POINT('',(-10.0197923273836,64.97,-13.1160858846074));
#36525=CARTESIAN_POINT('',(-7.91093399030624,61.3947146828798,-4.85500754770592));
#36526=CARTESIAN_POINT('',(-10.0358241714444,64.97,-13.1788877890042));
#36527=CARTESIAN_POINT('',(-9.89112836854344,64.97,-12.6120676561534));
#36528=CARTESIAN_POINT('',(-10.0358241714444,37.03,-13.1788877890042));
#36529=CARTESIAN_POINT('Origin',(-9.89112836854344,37.03,-12.6120676561534));
#36530=CARTESIAN_POINT('',(-9.69653989065522,64.5678155074499,-12.0809901437375));
#36531=CARTESIAN_POINT('',(-9.69653989065522,37.03,-12.0809901437375));
#36532=CARTESIAN_POINT('',(-7.22739122706622,62.2323640708404,-5.34210537381292));
#36533=CARTESIAN_POINT('Origin',(-6.8965715342494,37.28,-2.89929593438234));
#36534=CARTESIAN_POINT('',(-14.8720022673282,37.2481324154382,-5.97680680020517));
#36535=CARTESIAN_POINT('',(-12.7594118264622,38.5161005118285,-3.81349796890809));
#36536=CARTESIAN_POINT('',(-12.2041262243426,37.53,-4.65706016176646));
#36537=CARTESIAN_POINT('',(-12.1492258527638,37.3520314584495,-4.82659624346733));
#36538=CARTESIAN_POINT('',(-13.9714037445473,37.53,-5.33144828123002));
#36539=CARTESIAN_POINT('',(-6.98570187227364,37.53,-2.66572414061501));
#36540=CARTESIAN_POINT('',(-14.4379449459854,37.4321844925501,-5.61417442201851));
#36541=CARTESIAN_POINT('',(-11.2242343577003,38.1059743550986,-3.66665083902897));
#36542=CARTESIAN_POINT('',(-12.0847770735356,38.4299914950389,-3.64822471929515));
#36543=CARTESIAN_POINT('Origin',(-15.2807225748869,37.03,-6.39533953317997));
#36544=CARTESIAN_POINT('',(-14.8720022673282,64.7518675845618,-5.97680680020517));
#36545=CARTESIAN_POINT('',(-14.8720022673282,37.03,-5.97680680020517));
#36546=CARTESIAN_POINT('',(-15.2354376384623,64.97,-6.34896741059669));
#36547=CARTESIAN_POINT('',(-9.27857357711986,61.3947146828801,-0.249092876725649));
#36548=CARTESIAN_POINT('',(-15.2807225748869,64.97,-6.39533953317997));
#36549=CARTESIAN_POINT('',(-14.8720022673282,64.97,-5.97680680020517));
#36550=CARTESIAN_POINT('',(-15.2807225748869,37.03,-6.39533953317997));
#36551=CARTESIAN_POINT('Origin',(-14.8720022673282,37.03,-5.97680680020517));
#36552=CARTESIAN_POINT('',(-14.4379449459854,64.5678155074499,-5.61417442201851));
#36553=CARTESIAN_POINT('',(-14.4379449459854,37.03,-5.61417442201851));
#36554=CARTESIAN_POINT('',(-8.93015709263458,62.2323640708404,-1.01270334988218));
#36555=CARTESIAN_POINT('Origin',(-7.42225411486777,37.28,0.937421834860659));
#36556=CARTESIAN_POINT('',(-15.8679351687486,37.2481324154382,2.25993461117486));
#36557=CARTESIAN_POINT('',(-12.9567237635179,38.5161005118285,3.07711979487634));
#36558=CARTESIAN_POINT('',(-12.8976134221558,37.53,2.0689307051291));
#36559=CARTESIAN_POINT('',(-12.9348363465418,37.3520314584495,1.89465796572867));
#36560=CARTESIAN_POINT('',(-14.765314709922,37.53,2.36853222176556));
#36561=CARTESIAN_POINT('',(-7.38265735496099,37.53,1.18426611088278));
#36562=CARTESIAN_POINT('',(-15.3107143126737,37.4321844925501,2.35695480224783));
#36563=CARTESIAN_POINT('',(-11.5537975113131,38.1059743550986,2.43670440544354));
#36564=CARTESIAN_POINT('',(-12.2898363044011,38.4299914950389,2.88293325114382));
#36565=CARTESIAN_POINT('Origin',(-16.4311637046244,37.03,2.10183478588268));
#36566=CARTESIAN_POINT('',(-15.8679351687486,64.7518675845618,2.25993461117486));
#36567=CARTESIAN_POINT('',(-15.8679351687486,37.03,2.25993461117486));
#36568=CARTESIAN_POINT('',(-16.3687597379803,64.97,2.1193517538549));
#36569=CARTESIAN_POINT('',(-8.16002686703167,61.39471468288,4.42356602941383));
#36570=CARTESIAN_POINT('',(-16.4311637046244,64.97,2.10183478588268));
#36571=CARTESIAN_POINT('',(-15.8679351687486,64.97,2.25993461117486));
#36572=CARTESIAN_POINT('',(-16.4311637046244,37.03,2.10183478588268));
#36573=CARTESIAN_POINT('Origin',(-15.8679351687486,37.03,2.25993461117486));
#36574=CARTESIAN_POINT('',(-15.3107143126737,64.5678155074499,2.35695480224783));
#36575=CARTESIAN_POINT('',(-15.3107143126737,37.03,2.35695480224783));
#36576=CARTESIAN_POINT('',(-8.24009457694845,62.2323640708404,3.58805171882167));
#36577=CARTESIAN_POINT('Origin',(-5.95914969938874,37.28,4.52295818048543));
#36578=CARTESIAN_POINT('',(-12.6120676561534,37.2481324154382,9.89112836854343));
#36579=CARTESIAN_POINT('',(-9.68229203158586,38.5161005118285,9.14322579460982));
#36580=CARTESIAN_POINT('',(-10.1351955192135,37.53,8.24055326038937));
#36581=CARTESIAN_POINT('',(-10.2545678870352,37.3520314584495,8.10824010307447));
#36582=CARTESIAN_POINT('',(-11.6028715227817,37.53,9.43386642869196));
#36583=CARTESIAN_POINT('',(-5.80143576139086,37.53,4.71693321434598));
#36584=CARTESIAN_POINT('',(-12.0809901437375,37.4321844925501,9.69653989065521));
#36585=CARTESIAN_POINT('',(-8.78752995225676,38.1059743550986,7.88714667228409));
#36586=CARTESIAN_POINT('',(-9.20184382239172,38.4299914950389,8.64161158510596));
#36587=CARTESIAN_POINT('Origin',(-13.1788877890042,37.03,10.0358241714444));
#36588=CARTESIAN_POINT('',(-12.6120676561534,64.7518675845618,9.89112836854343));
#36589=CARTESIAN_POINT('',(-12.6120676561534,37.03,9.89112836854343));
#36590=CARTESIAN_POINT('',(-13.1160858846074,64.97,10.0197923273836));
#36591=CARTESIAN_POINT('',(-4.85500754770607,61.39471468288,7.91093399030606));
#36592=CARTESIAN_POINT('',(-13.1788877890042,64.97,10.0358241714444));
#36593=CARTESIAN_POINT('',(-12.6120676561534,64.97,9.89112836854343));
#36594=CARTESIAN_POINT('',(-13.1788877890042,37.03,10.0358241714444));
#36595=CARTESIAN_POINT('Origin',(-12.6120676561534,37.03,9.89112836854343));
#36596=CARTESIAN_POINT('',(-12.0809901437375,64.5678155074499,9.69653989065521));
#36597=CARTESIAN_POINT('',(-12.0809901437375,37.03,9.69653989065521));
#36598=CARTESIAN_POINT('',(-5.34210537381293,62.2323640708404,7.22739122706621));
#36599=CARTESIAN_POINT('Origin',(-2.89929593438233,37.28,6.8965715342494));
#36600=CARTESIAN_POINT('',(-5.97680680020517,37.2481324154382,14.8720022673282));
#36601=CARTESIAN_POINT('',(-3.81349796890809,38.5161005118285,12.7594118264622));
#36602=CARTESIAN_POINT('',(-4.65706016176645,37.53,12.2041262243426));
#36603=CARTESIAN_POINT('',(-4.82659624346733,37.3520314584495,12.1492258527638));
#36604=CARTESIAN_POINT('',(-5.33144828123002,37.53,13.9714037445473));
#36605=CARTESIAN_POINT('',(-2.66572414061501,37.53,6.98570187227364));
#36606=CARTESIAN_POINT('',(-5.6141744220185,37.4321844925501,14.4379449459854));
#36607=CARTESIAN_POINT('',(-3.66665083902899,38.1059743550985,11.2242343577003));
#36608=CARTESIAN_POINT('',(-3.64822471929515,38.4299914950389,12.0847770735356));
#36609=CARTESIAN_POINT('Origin',(-6.39533953317997,37.03,15.2807225748869));
#36610=CARTESIAN_POINT('',(-5.97680680020517,64.7518675845618,14.8720022673282));
#36611=CARTESIAN_POINT('',(-5.97680680020517,37.03,14.8720022673282));
#36612=CARTESIAN_POINT('',(-6.34896741059669,64.97,15.2354376384623));
#36613=CARTESIAN_POINT('',(-0.24909287672559,61.39471468288,9.27857357711989));
#36614=CARTESIAN_POINT('',(-6.39533953317997,64.97,15.2807225748869));
#36615=CARTESIAN_POINT('',(-5.97680680020517,64.97,14.8720022673282));
#36616=CARTESIAN_POINT('',(-6.39533953317997,37.03,15.2807225748869));
#36617=CARTESIAN_POINT('Origin',(-5.97680680020517,37.03,14.8720022673282));
#36618=CARTESIAN_POINT('',(-5.6141744220185,64.5678155074499,14.4379449459854));
#36619=CARTESIAN_POINT('',(-5.6141744220185,37.03,14.4379449459854));
#36620=CARTESIAN_POINT('',(-1.01270334988219,62.2323640708404,8.93015709263459));
#36621=CARTESIAN_POINT('Origin',(0.937421834860657,37.28,7.42225411486777));
#36622=CARTESIAN_POINT('',(2.25993461117485,37.2481324154382,15.8679351687486));
#36623=CARTESIAN_POINT('',(3.07711979487634,38.5161005118285,12.9567237635179));
#36624=CARTESIAN_POINT('',(2.0689307051291,37.53,12.8976134221558));
#36625=CARTESIAN_POINT('',(1.89465796572866,37.3520314584495,12.9348363465418));
#36626=CARTESIAN_POINT('',(2.36853222176556,37.53,14.765314709922));
#36627=CARTESIAN_POINT('',(1.18426611088278,37.53,7.38265735496099));
#36628=CARTESIAN_POINT('',(2.35695480224784,37.4321844925501,15.3107143126737));
#36629=CARTESIAN_POINT('',(2.4367044054435,38.1059743550985,11.553797511313));
#36630=CARTESIAN_POINT('',(2.88293325114383,38.4299914950389,12.2898363044011));
#36631=CARTESIAN_POINT('Origin',(2.10183478588268,37.03,16.4311637046244));
#36632=CARTESIAN_POINT('',(2.25993461117485,64.7518675845618,15.8679351687486));
#36633=CARTESIAN_POINT('',(2.25993461117485,37.03,15.8679351687486));
#36634=CARTESIAN_POINT('',(2.11935175385489,64.97,16.3687597379803));
#36635=CARTESIAN_POINT('',(4.42356602941384,61.39471468288,8.16002686703167));
#36636=CARTESIAN_POINT('',(2.10183478588268,64.97,16.4311637046244));
#36637=CARTESIAN_POINT('',(2.25993461117485,64.97,15.8679351687486));
#36638=CARTESIAN_POINT('',(2.10183478588268,37.03,16.4311637046244));
#36639=CARTESIAN_POINT('Origin',(2.25993461117485,37.03,15.8679351687486));
#36640=CARTESIAN_POINT('',(2.35695480224784,64.5678155074499,15.3107143126737));
#36641=CARTESIAN_POINT('',(2.35695480224784,37.03,15.3107143126737));
#36642=CARTESIAN_POINT('',(3.58805171882171,62.2323640708404,8.24009457694843));
#36643=CARTESIAN_POINT('Origin',(4.52295818048543,37.28,5.95914969938874));
#36644=CARTESIAN_POINT('',(9.89112836854343,37.2481324154382,12.6120676561534));
#36645=CARTESIAN_POINT('',(9.14322579460982,38.5161005118285,9.68229203158586));
#36646=CARTESIAN_POINT('',(8.24055326038937,37.53,10.1351955192135));
#36647=CARTESIAN_POINT('',(8.10824010307447,37.3520314584495,10.2545678870352));
#36648=CARTESIAN_POINT('',(9.43386642869196,37.53,11.6028715227817));
#36649=CARTESIAN_POINT('',(4.71693321434598,37.53,5.80143576139086));
#36650=CARTESIAN_POINT('',(9.69653989065521,37.4321844925501,12.0809901437375));
#36651=CARTESIAN_POINT('',(7.88714667228404,38.1059743550985,8.78752995225676));
#36652=CARTESIAN_POINT('',(8.641611585106,38.4299914950389,9.20184382239174));
#36653=CARTESIAN_POINT('Origin',(10.0358241714444,37.03,13.1788877890042));
#36654=CARTESIAN_POINT('',(9.89112836854343,64.7518675845618,12.6120676561534));
#36655=CARTESIAN_POINT('',(9.89112836854343,37.03,12.6120676561534));
#36656=CARTESIAN_POINT('',(10.0197923273836,64.97,13.1160858846074));
#36657=CARTESIAN_POINT('',(7.91093399030605,61.3947146828801,4.85500754770609));
#36658=CARTESIAN_POINT('',(10.0358241714444,64.97,13.1788877890042));
#36659=CARTESIAN_POINT('',(9.89112836854343,64.97,12.6120676561534));
#36660=CARTESIAN_POINT('',(10.0358241714444,37.03,13.1788877890042));
#36661=CARTESIAN_POINT('Origin',(9.89112836854343,37.03,12.6120676561534));
#36662=CARTESIAN_POINT('',(9.69653989065521,64.5678155074499,12.0809901437375));
#36663=CARTESIAN_POINT('',(9.69653989065521,37.03,12.0809901437375));
#36664=CARTESIAN_POINT('',(7.22739122706626,62.2323640708404,5.34210537381285));
#36665=CARTESIAN_POINT('Origin',(6.8965715342494,37.28,2.89929593438233));
#36666=CARTESIAN_POINT('',(14.8720022673282,37.2481324154382,5.97680680020517));
#36667=CARTESIAN_POINT('',(12.7594118264622,38.5161005118285,3.81349796890809));
#36668=CARTESIAN_POINT('',(12.2041262243426,37.53,4.65706016176646));
#36669=CARTESIAN_POINT('',(12.1492258527638,37.3520314584495,4.82659624346733));
#36670=CARTESIAN_POINT('',(13.9714037445473,37.53,5.33144828123002));
#36671=CARTESIAN_POINT('',(6.98570187227364,37.53,2.66572414061501));
#36672=CARTESIAN_POINT('',(14.4379449459854,37.4321844925501,5.6141744220185));
#36673=CARTESIAN_POINT('',(11.2242343577003,38.1059743550985,3.66665083902898));
#36674=CARTESIAN_POINT('',(12.0847770735356,38.4299914950389,3.64822471929515));
#36675=CARTESIAN_POINT('Origin',(15.2807225748869,37.03,6.39533953317997));
#36676=CARTESIAN_POINT('',(14.8720022673282,64.7518675845618,5.97680680020517));
#36677=CARTESIAN_POINT('',(14.8720022673282,37.03,5.97680680020517));
#36678=CARTESIAN_POINT('',(15.2354376384623,64.97,6.34896741059669));
#36679=CARTESIAN_POINT('',(9.27857357711988,61.39471468288,0.249092876725602));
#36680=CARTESIAN_POINT('',(15.2807225748869,64.97,6.39533953317997));
#36681=CARTESIAN_POINT('',(14.8720022673282,64.97,5.97680680020517));
#36682=CARTESIAN_POINT('',(15.2807225748869,37.03,6.39533953317997));
#36683=CARTESIAN_POINT('Origin',(14.8720022673282,37.03,5.97680680020517));
#36684=CARTESIAN_POINT('',(14.4379449459854,64.5678155074499,5.6141744220185));
#36685=CARTESIAN_POINT('',(14.4379449459854,37.03,5.6141744220185));
#36686=CARTESIAN_POINT('',(8.93015709263458,62.2323640708404,1.01270334988217));
#36687=CARTESIAN_POINT('Origin',(7.42225411486777,37.28,-0.937421834860657));
#36688=CARTESIAN_POINT('',(15.8679351687486,37.2481324154382,-2.25993461117485));
#36689=CARTESIAN_POINT('',(12.9567237635179,38.5161005118285,-3.07711979487634));
#36690=CARTESIAN_POINT('',(12.8976134221558,37.53,-2.0689307051291));
#36691=CARTESIAN_POINT('',(12.9348363465418,37.3520314584495,-1.89465796572866));
#36692=CARTESIAN_POINT('',(14.765314709922,37.53,-2.36853222176556));
#36693=CARTESIAN_POINT('',(7.38265735496099,37.53,-1.18426611088278));
#36694=CARTESIAN_POINT('',(15.3107143126737,37.4321844925501,-2.35695480224783));
#36695=CARTESIAN_POINT('',(11.553797511313,38.1059743550985,-2.43670440544351));
#36696=CARTESIAN_POINT('',(12.2898363044011,38.4299914950389,-2.88293325114382));
#36697=CARTESIAN_POINT('Origin',(16.4311637046244,37.03,-2.10183478588267));
#36698=CARTESIAN_POINT('',(15.8679351687486,64.7518675845618,-2.25993461117485));
#36699=CARTESIAN_POINT('',(15.8679351687486,37.03,-2.25993461117485));
#36700=CARTESIAN_POINT('',(16.3687597379803,64.97,-2.11935175385489));
#36701=CARTESIAN_POINT('',(8.16002686703167,61.39471468288,-4.42356602941385));
#36702=CARTESIAN_POINT('',(16.4311637046244,64.97,-2.10183478588267));
#36703=CARTESIAN_POINT('',(15.8679351687486,64.97,-2.25993461117485));
#36704=CARTESIAN_POINT('',(16.4311637046244,37.03,-2.10183478588267));
#36705=CARTESIAN_POINT('Origin',(15.8679351687486,37.03,-2.25993461117485));
#36706=CARTESIAN_POINT('',(15.3107143126737,64.5678155074499,-2.35695480224783));
#36707=CARTESIAN_POINT('',(15.3107143126737,37.03,-2.35695480224783));
#36708=CARTESIAN_POINT('',(8.24009457694844,62.2323640708404,-3.58805171882169));
#36709=CARTESIAN_POINT('Origin',(5.95914969938874,37.28,-4.52295818048544));
#36710=CARTESIAN_POINT('',(12.6120676561534,37.2481324154382,-9.89112836854343));
#36711=CARTESIAN_POINT('',(9.68229203158587,38.5161005118285,-9.14322579460984));
#36712=CARTESIAN_POINT('',(10.1351955192135,37.53,-8.24055326038936));
#36713=CARTESIAN_POINT('',(10.2545678870352,37.3520314584495,-8.10824010307447));
#36714=CARTESIAN_POINT('',(11.6028715227817,37.53,-9.43386642869196));
#36715=CARTESIAN_POINT('',(5.80143576139085,37.53,-4.71693321434598));
#36716=CARTESIAN_POINT('',(12.0809901437375,37.4321844925501,-9.69653989065521));
#36717=CARTESIAN_POINT('',(8.78752995225676,38.1059743550985,-7.88714667228404));
#36718=CARTESIAN_POINT('',(9.20184382239173,38.4299914950389,-8.64161158510599));
#36719=CARTESIAN_POINT('Origin',(13.1788877890042,37.03,-10.0358241714444));
#36720=CARTESIAN_POINT('',(12.6120676561534,64.7518675845618,-9.89112836854343));
#36721=CARTESIAN_POINT('',(12.6120676561534,37.03,-9.89112836854343));
#36722=CARTESIAN_POINT('',(13.1160858846074,64.97,-10.0197923273836));
#36723=CARTESIAN_POINT('',(4.85500754770605,61.39471468288,-7.91093399030609));
#36724=CARTESIAN_POINT('',(13.1788877890042,64.97,-10.0358241714444));
#36725=CARTESIAN_POINT('',(12.6120676561534,64.97,-9.89112836854343));
#36726=CARTESIAN_POINT('',(13.1788877890042,37.03,-10.0358241714444));
#36727=CARTESIAN_POINT('Origin',(12.6120676561534,37.03,-9.89112836854343));
#36728=CARTESIAN_POINT('',(12.0809901437375,64.5678155074499,-9.69653989065521));
#36729=CARTESIAN_POINT('',(12.0809901437375,37.03,-9.69653989065521));
#36730=CARTESIAN_POINT('',(5.34210537381288,62.2323640708404,-7.22739122706624));
#36731=CARTESIAN_POINT('Origin',(2.89929593438233,37.28,-6.8965715342494));
#36732=CARTESIAN_POINT('',(5.97680680020517,37.2481324154382,-14.8720022673282));
#36733=CARTESIAN_POINT('',(3.81349796890809,38.5161005118285,-12.7594118264622));
#36734=CARTESIAN_POINT('',(4.65706016176646,37.53,-12.2041262243426));
#36735=CARTESIAN_POINT('',(4.82659624346733,37.3520314584495,-12.1492258527638));
#36736=CARTESIAN_POINT('',(5.33144828123002,37.53,-13.9714037445473));
#36737=CARTESIAN_POINT('',(2.66572414061501,37.53,-6.98570187227364));
#36738=CARTESIAN_POINT('',(5.61417442201851,37.4321844925501,-14.4379449459854));
#36739=CARTESIAN_POINT('',(3.66665083902899,38.1059743550985,-11.2242343577003));
#36740=CARTESIAN_POINT('',(3.64822471929515,38.4299914950389,-12.0847770735356));
#36741=CARTESIAN_POINT('Origin',(6.39533953317997,37.03,-15.2807225748869));
#36742=CARTESIAN_POINT('',(5.97680680020517,64.7518675845618,-14.8720022673282));
#36743=CARTESIAN_POINT('',(5.97680680020517,37.03,-14.8720022673282));
#36744=CARTESIAN_POINT('',(6.34896741059669,64.97,-15.2354376384623));
#36745=CARTESIAN_POINT('',(0.249092876725617,61.39471468288,-9.27857357711988));
#36746=CARTESIAN_POINT('',(6.39533953317997,64.97,-15.2807225748869));
#36747=CARTESIAN_POINT('',(5.97680680020517,64.97,-14.8720022673282));
#36748=CARTESIAN_POINT('',(6.39533953317997,37.03,-15.2807225748869));
#36749=CARTESIAN_POINT('Origin',(5.97680680020517,37.03,-14.8720022673282));
#36750=CARTESIAN_POINT('',(5.61417442201851,64.5678155074499,-14.4379449459854));
#36751=CARTESIAN_POINT('',(5.61417442201851,37.03,-14.4379449459854));
#36752=CARTESIAN_POINT('',(1.01270334988216,62.2323640708403,-8.93015709263459));
#36753=CARTESIAN_POINT('Origin',(-0.937421834860655,37.28,-7.42225411486777));
#36754=CARTESIAN_POINT('',(-2.25993461117485,37.2481324154382,-15.8679351687486));
#36755=CARTESIAN_POINT('',(-3.07711979487634,38.5161005118285,-12.9567237635179));
#36756=CARTESIAN_POINT('',(-2.0689307051291,37.53,-12.8976134221558));
#36757=CARTESIAN_POINT('',(-1.89465796572866,37.3520314584495,-12.9348363465418));
#36758=CARTESIAN_POINT('',(-2.36853222176555,37.53,-14.765314709922));
#36759=CARTESIAN_POINT('',(-1.18426611088278,37.53,-7.38265735496099));
#36760=CARTESIAN_POINT('',(-2.35695480224783,37.4321844925501,-15.3107143126737));
#36761=CARTESIAN_POINT('',(-2.4367044054435,38.1059743550985,-11.553797511313));
#36762=CARTESIAN_POINT('',(-2.88293325114383,38.4299914950389,-12.2898363044011));
#36763=CARTESIAN_POINT('Origin',(-2.10183478588267,37.03,-16.4311637046244));
#36764=CARTESIAN_POINT('',(-2.25993461117485,64.7518675845618,-15.8679351687486));
#36765=CARTESIAN_POINT('',(-2.25993461117485,37.03,-15.8679351687486));
#36766=CARTESIAN_POINT('',(-2.11935175385489,64.97,-16.3687597379803));
#36767=CARTESIAN_POINT('',(-4.42356602941384,61.39471468288,-8.16002686703167));
#36768=CARTESIAN_POINT('',(-2.10183478588267,64.97,-16.4311637046244));
#36769=CARTESIAN_POINT('',(-2.25993461117485,64.97,-15.8679351687486));
#36770=CARTESIAN_POINT('',(-2.10183478588267,37.03,-16.4311637046244));
#36771=CARTESIAN_POINT('Origin',(-2.25993461117485,37.03,-15.8679351687486));
#36772=CARTESIAN_POINT('',(-2.35695480224783,64.5678155074499,-15.3107143126737));
#36773=CARTESIAN_POINT('',(-2.35695480224783,37.03,-15.3107143126737));
#36774=CARTESIAN_POINT('',(-3.58805171882171,62.2323640708404,-8.24009457694843));
#36775=CARTESIAN_POINT('Origin',(-2.56210187465055,37.28,-6.01293277414708));
#36776=CARTESIAN_POINT('',(-5.61417442201851,37.4321844925501,-14.4379449459854));
#36777=CARTESIAN_POINT('',(-5.33144828123003,37.53,-13.9714037445473));
#36778=CARTESIAN_POINT('',(-3.29608808746436,38.2341789260845,-10.6127493678757));
#36779=CARTESIAN_POINT('',(-4.65706016176646,37.53,-12.2041262243426));
#36780=CARTESIAN_POINT('',(-2.32853008088323,37.53,-6.10206311217132));
#36781=CARTESIAN_POINT('',(-4.49554999076345,37.6995434345929,-12.2564275888243));
#36782=CARTESIAN_POINT('',(-5.97680680020517,37.2481324154382,-14.8720022673282));
#36783=CARTESIAN_POINT('',(-3.37431437066651,38.7735167359811,-12.3305248094967));
#36784=CARTESIAN_POINT('',(-3.22502994327358,38.6447816854218,-11.5782288391921));
#36785=CARTESIAN_POINT('Origin',(-4.65706016176646,37.03,-12.2041262243426));
#36786=CARTESIAN_POINT('',(-5.33144828123003,64.47,-13.9714037445473));
#36787=CARTESIAN_POINT('',(-5.33144828123003,37.03,-13.9714037445473));
#36788=CARTESIAN_POINT('',(-4.65706016176646,64.47,-12.2041262243426));
#36789=CARTESIAN_POINT('',(-2.32853008088323,64.47,-6.10206311217132));
#36790=CARTESIAN_POINT('',(-4.65706016176646,37.03,-12.2041262243426));
#36791=CARTESIAN_POINT('Origin',(-5.33144828123003,37.03,-13.9714037445473));
#36792=CARTESIAN_POINT('',(-5.61417442201851,64.5678155074499,-14.4379449459854));
#36793=CARTESIAN_POINT('',(-5.61417442201851,37.03,-14.4379449459854));
#36794=CARTESIAN_POINT('',(-2.03831674197423,63.3306666093445,-8.53723504499476));
#36795=CARTESIAN_POINT('Origin',(-5.22531169760465,37.28,-3.92630159633413));
#36796=CARTESIAN_POINT('',(-12.0809901437375,37.4321844925501,-9.69653989065521));
#36797=CARTESIAN_POINT('',(-11.6028715227817,37.53,-9.43386642869196));
#36798=CARTESIAN_POINT('',(-8.16087070079327,38.2341789260846,-7.54286651284552));
#36799=CARTESIAN_POINT('',(-10.1351955192135,37.53,-8.24055326038937));
#36800=CARTESIAN_POINT('',(-5.06759775960677,37.53,-4.12027663019468));
#36801=CARTESIAN_POINT('',(-10.0214742903962,37.6995434345929,-8.36660265618453));
#36802=CARTESIAN_POINT('',(-12.6120676561534,37.2481324154382,-9.89112836854343));
#36803=CARTESIAN_POINT('',(-9.08750437010039,38.773516735981,-8.99139054168508));
#36804=CARTESIAN_POINT('',(-8.58207227843645,38.6447816854217,-8.41452533393317));
#36805=CARTESIAN_POINT('Origin',(-10.1351955192135,37.03,-8.24055326038937));
#36806=CARTESIAN_POINT('',(-11.6028715227817,64.47,-9.43386642869196));
#36807=CARTESIAN_POINT('',(-11.6028715227817,37.03,-9.43386642869196));
#36808=CARTESIAN_POINT('',(-10.1351955192135,64.47,-8.24055326038937));
#36809=CARTESIAN_POINT('',(-5.06759775960677,64.47,-4.12027663019468));
#36810=CARTESIAN_POINT('',(-10.1351955192135,37.03,-8.24055326038937));
#36811=CARTESIAN_POINT('Origin',(-11.6028715227817,37.03,-9.43386642869196));
#36812=CARTESIAN_POINT('',(-12.0809901437375,64.5678155074499,-9.69653989065521));
#36813=CARTESIAN_POINT('',(-12.0809901437375,37.03,-9.69653989065521));
#36814=CARTESIAN_POINT('',(-6.03385160200604,63.3306666093444,-6.37430405605714));
#36815=CARTESIAN_POINT('Origin',(-6.48840347098469,37.28,-0.787621076542431));
#36816=CARTESIAN_POINT('',(-15.3107143126737,37.4321844925501,-2.35695480224783));
#36817=CARTESIAN_POINT('',(-14.765314709922,37.53,-2.36853222176556));
#36818=CARTESIAN_POINT('',(-10.8389546003099,38.2341789260846,-2.45187866708253));
#36819=CARTESIAN_POINT('',(-12.8976134221558,37.53,-2.0689307051291));
#36820=CARTESIAN_POINT('',(-6.44880671107791,37.53,-1.03446535256455));
#36821=CARTESIAN_POINT('',(-12.862152646948,37.6995434345929,-2.23495329842808));
#36822=CARTESIAN_POINT('',(-15.8679351687486,37.2481324154382,-2.25993461117485));
#36823=CARTESIAN_POINT('',(-12.3657049123516,38.773516735981,-3.24302043939622));
#36824=CARTESIAN_POINT('',(-11.6395552772067,38.6447816854217,-2.99615656075563));
#36825=CARTESIAN_POINT('Origin',(-12.8976134221558,37.03,-2.0689307051291));
#36826=CARTESIAN_POINT('',(-14.765314709922,64.47,-2.36853222176556));
#36827=CARTESIAN_POINT('',(-14.765314709922,37.03,-2.36853222176556));
#36828=CARTESIAN_POINT('',(-12.8976134221558,64.47,-2.0689307051291));
#36829=CARTESIAN_POINT('',(-6.44880671107791,64.47,-1.03446535256455));
#36830=CARTESIAN_POINT('',(-12.8976134221558,37.03,-2.0689307051291));
#36831=CARTESIAN_POINT('Origin',(-14.765314709922,37.03,-2.36853222176556));
#36832=CARTESIAN_POINT('',(-15.3107143126737,64.5678155074499,-2.35695480224783));
#36833=CARTESIAN_POINT('',(-15.3107143126737,37.03,-2.35695480224783));
#36834=CARTESIAN_POINT('',(-8.41262079803121,63.3306666093444,-2.50338344298866));
#36835=CARTESIAN_POINT('Origin',(-6.01293277414708,37.28,2.56210187465055));
#36836=CARTESIAN_POINT('',(-14.4379449459854,37.4321844925501,5.61417442201851));
#36837=CARTESIAN_POINT('',(-13.9714037445473,37.53,5.33144828123002));
#36838=CARTESIAN_POINT('',(-10.6127493678758,38.2341789260846,3.29608808746433));
#36839=CARTESIAN_POINT('',(-12.2041262243426,37.53,4.65706016176645));
#36840=CARTESIAN_POINT('',(-6.10206311217132,37.53,2.32853008088323));
#36841=CARTESIAN_POINT('',(-12.2564275888243,37.6995434345929,4.49554999076345));
#36842=CARTESIAN_POINT('',(-14.8720022673282,37.2481324154382,5.97680680020517));
#36843=CARTESIAN_POINT('',(-12.3305248094966,38.773516735981,3.3743143706665));
#36844=CARTESIAN_POINT('',(-11.5782288391921,38.6447816854218,3.22502994327358));
#36845=CARTESIAN_POINT('Origin',(-12.2041262243426,37.03,4.65706016176645));
#36846=CARTESIAN_POINT('',(-13.9714037445473,64.47,5.33144828123002));
#36847=CARTESIAN_POINT('',(-13.9714037445473,37.03,5.33144828123002));
#36848=CARTESIAN_POINT('',(-12.2041262243426,64.47,4.65706016176645));
#36849=CARTESIAN_POINT('',(-6.10206311217132,64.47,2.32853008088323));
#36850=CARTESIAN_POINT('',(-12.2041262243426,37.03,4.65706016176645));
#36851=CARTESIAN_POINT('Origin',(-13.9714037445473,37.03,5.33144828123002));
#36852=CARTESIAN_POINT('',(-14.4379449459854,64.5678155074499,5.61417442201851));
#36853=CARTESIAN_POINT('',(-14.4379449459854,37.03,5.61417442201851));
#36854=CARTESIAN_POINT('',(-8.53723504499469,63.3306666093444,2.0383167419741));
#36855=CARTESIAN_POINT('Origin',(-3.92630159633414,37.28,5.22531169760465));
#36856=CARTESIAN_POINT('',(-9.6965398906552,37.4321844925501,12.0809901437375));
#36857=CARTESIAN_POINT('',(-9.43386642869196,37.53,11.6028715227817));
#36858=CARTESIAN_POINT('',(-7.54286651284552,38.2341789260846,8.16087070079328));
#36859=CARTESIAN_POINT('',(-8.24055326038936,37.53,10.1351955192135));
#36860=CARTESIAN_POINT('',(-4.12027663019469,37.53,5.06759775960677));
#36861=CARTESIAN_POINT('',(-8.36660265618453,37.6995434345929,10.0214742903962));
#36862=CARTESIAN_POINT('',(-9.89112836854343,37.2481324154382,12.6120676561534));
#36863=CARTESIAN_POINT('',(-8.9913905416851,38.773516735981,9.08750437010041));
#36864=CARTESIAN_POINT('',(-8.41452533393316,38.6447816854217,8.58207227843645));
#36865=CARTESIAN_POINT('Origin',(-8.24055326038936,37.03,10.1351955192135));
#36866=CARTESIAN_POINT('',(-9.43386642869196,64.47,11.6028715227817));
#36867=CARTESIAN_POINT('',(-9.43386642869196,37.03,11.6028715227817));
#36868=CARTESIAN_POINT('',(-8.24055326038936,64.47,10.1351955192135));
#36869=CARTESIAN_POINT('',(-4.12027663019469,64.47,5.06759775960677));
#36870=CARTESIAN_POINT('',(-8.24055326038936,37.03,10.1351955192135));
#36871=CARTESIAN_POINT('Origin',(-9.43386642869196,37.03,11.6028715227817));
#36872=CARTESIAN_POINT('',(-9.6965398906552,64.5678155074499,12.0809901437375));
#36873=CARTESIAN_POINT('',(-9.6965398906552,37.03,12.0809901437375));
#36874=CARTESIAN_POINT('',(-6.37430405605714,63.3306666093444,6.03385160200603));
#36875=CARTESIAN_POINT('Origin',(-0.787621076542428,37.28,6.48840347098469));
#36876=CARTESIAN_POINT('',(-2.35695480224783,37.4321844925501,15.3107143126737));
#36877=CARTESIAN_POINT('',(-2.36853222176555,37.53,14.765314709922));
#36878=CARTESIAN_POINT('',(-2.45187866708248,38.2341789260845,10.8389546003098));
#36879=CARTESIAN_POINT('',(-2.0689307051291,37.53,12.8976134221558));
#36880=CARTESIAN_POINT('',(-1.03446535256455,37.53,6.44880671107791));
#36881=CARTESIAN_POINT('',(-2.23495329842808,37.6995434345929,12.862152646948));
#36882=CARTESIAN_POINT('',(-2.25993461117485,37.2481324154382,15.8679351687486));
#36883=CARTESIAN_POINT('',(-3.24302043939622,38.773516735981,12.3657049123516));
#36884=CARTESIAN_POINT('',(-2.99615656075565,38.6447816854218,11.6395552772068));
#36885=CARTESIAN_POINT('Origin',(-2.0689307051291,37.03,12.8976134221558));
#36886=CARTESIAN_POINT('',(-2.36853222176555,64.47,14.765314709922));
#36887=CARTESIAN_POINT('',(-2.36853222176555,37.03,14.765314709922));
#36888=CARTESIAN_POINT('',(-2.0689307051291,64.47,12.8976134221558));
#36889=CARTESIAN_POINT('',(-1.03446535256455,64.47,6.44880671107791));
#36890=CARTESIAN_POINT('',(-2.0689307051291,37.03,12.8976134221558));
#36891=CARTESIAN_POINT('Origin',(-2.36853222176555,37.03,14.765314709922));
#36892=CARTESIAN_POINT('',(-2.35695480224783,64.5678155074499,15.3107143126737));
#36893=CARTESIAN_POINT('',(-2.35695480224783,37.03,15.3107143126737));
#36894=CARTESIAN_POINT('',(-2.50338344298858,63.3306666093445,8.41262079803133));
#36895=CARTESIAN_POINT('Origin',(2.56210187465055,37.28,6.01293277414708));
#36896=CARTESIAN_POINT('',(5.61417442201851,37.4321844925501,14.4379449459854));
#36897=CARTESIAN_POINT('',(5.33144828123002,37.53,13.9714037445473));
#36898=CARTESIAN_POINT('',(3.29608808746436,38.2341789260845,10.6127493678757));
#36899=CARTESIAN_POINT('',(4.65706016176646,37.53,12.2041262243426));
#36900=CARTESIAN_POINT('',(2.32853008088323,37.53,6.10206311217132));
#36901=CARTESIAN_POINT('',(4.49554999076345,37.6995434345929,12.2564275888243));
#36902=CARTESIAN_POINT('',(5.97680680020517,37.2481324154382,14.8720022673282));
#36903=CARTESIAN_POINT('',(3.37431437066651,38.773516735981,12.3305248094966));
#36904=CARTESIAN_POINT('',(3.22502994327357,38.6447816854218,11.5782288391921));
#36905=CARTESIAN_POINT('Origin',(4.65706016176646,37.03,12.2041262243426));
#36906=CARTESIAN_POINT('',(5.33144828123002,64.47,13.9714037445473));
#36907=CARTESIAN_POINT('',(5.33144828123002,37.03,13.9714037445473));
#36908=CARTESIAN_POINT('',(4.65706016176646,64.47,12.2041262243426));
#36909=CARTESIAN_POINT('',(2.32853008088323,64.47,6.10206311217132));
#36910=CARTESIAN_POINT('',(4.65706016176646,37.03,12.2041262243426));
#36911=CARTESIAN_POINT('Origin',(5.33144828123002,37.03,13.9714037445473));
#36912=CARTESIAN_POINT('',(5.61417442201851,64.5678155074499,14.4379449459854));
#36913=CARTESIAN_POINT('',(5.61417442201851,37.03,14.4379449459854));
#36914=CARTESIAN_POINT('',(2.03831674197423,63.3306666093445,8.53723504499476));
#36915=CARTESIAN_POINT('Origin',(5.22531169760465,37.28,3.92630159633414));
#36916=CARTESIAN_POINT('',(12.0809901437375,37.4321844925501,9.69653989065521));
#36917=CARTESIAN_POINT('',(11.6028715227817,37.53,9.43386642869196));
#36918=CARTESIAN_POINT('',(8.16087070079327,38.2341789260845,7.54286651284547));
#36919=CARTESIAN_POINT('',(10.1351955192135,37.53,8.24055326038936));
#36920=CARTESIAN_POINT('',(5.06759775960677,37.53,4.12027663019469));
#36921=CARTESIAN_POINT('',(10.0214742903962,37.6995434345929,8.36660265618453));
#36922=CARTESIAN_POINT('',(12.6120676561534,37.2481324154382,9.89112836854343));
#36923=CARTESIAN_POINT('',(9.08750437010041,38.773516735981,8.9913905416851));
#36924=CARTESIAN_POINT('',(8.58207227843646,38.6447816854218,8.41452533393319));
#36925=CARTESIAN_POINT('Origin',(10.1351955192135,37.03,8.24055326038936));
#36926=CARTESIAN_POINT('',(11.6028715227817,64.47,9.43386642869196));
#36927=CARTESIAN_POINT('',(11.6028715227817,37.03,9.43386642869196));
#36928=CARTESIAN_POINT('',(10.1351955192135,64.47,8.24055326038936));
#36929=CARTESIAN_POINT('',(5.06759775960677,64.47,4.12027663019469));
#36930=CARTESIAN_POINT('',(10.1351955192135,37.03,8.24055326038936));
#36931=CARTESIAN_POINT('Origin',(11.6028715227817,37.03,9.43386642869196));
#36932=CARTESIAN_POINT('',(12.0809901437375,64.5678155074499,9.69653989065521));
#36933=CARTESIAN_POINT('',(12.0809901437375,37.03,9.69653989065521));
#36934=CARTESIAN_POINT('',(6.03385160200616,63.3306666093445,6.37430405605714));
#36935=CARTESIAN_POINT('Origin',(6.48840347098469,37.28,0.78762107654243));
#36936=CARTESIAN_POINT('',(15.3107143126737,37.4321844925501,2.35695480224783));
#36937=CARTESIAN_POINT('',(14.765314709922,37.53,2.36853222176556));
#36938=CARTESIAN_POINT('',(10.8389546003098,38.2341789260845,2.4518786670825));
#36939=CARTESIAN_POINT('',(12.8976134221558,37.53,2.0689307051291));
#36940=CARTESIAN_POINT('',(6.44880671107791,37.53,1.03446535256455));
#36941=CARTESIAN_POINT('',(12.862152646948,37.6995434345929,2.23495329842808));
#36942=CARTESIAN_POINT('',(15.8679351687486,37.2481324154382,2.25993461117485));
#36943=CARTESIAN_POINT('',(12.3657049123516,38.773516735981,3.24302043939622));
#36944=CARTESIAN_POINT('',(11.6395552772068,38.6447816854218,2.99615656075564));
#36945=CARTESIAN_POINT('Origin',(12.8976134221558,37.03,2.0689307051291));
#36946=CARTESIAN_POINT('',(14.765314709922,64.47,2.36853222176556));
#36947=CARTESIAN_POINT('',(14.765314709922,37.03,2.36853222176556));
#36948=CARTESIAN_POINT('',(12.8976134221558,64.47,2.0689307051291));
#36949=CARTESIAN_POINT('',(6.44880671107791,64.47,1.03446535256455));
#36950=CARTESIAN_POINT('',(12.8976134221558,37.03,2.0689307051291));
#36951=CARTESIAN_POINT('Origin',(14.765314709922,37.03,2.36853222176556));
#36952=CARTESIAN_POINT('',(15.3107143126737,64.5678155074499,2.35695480224783));
#36953=CARTESIAN_POINT('',(15.3107143126737,37.03,2.35695480224783));
#36954=CARTESIAN_POINT('',(8.4126207980313,63.3306666093445,2.5033834429886));
#36955=CARTESIAN_POINT('Origin',(6.01293277414708,37.28,-2.56210187465055));
#36956=CARTESIAN_POINT('',(14.4379449459854,37.4321844925501,-5.6141744220185));
#36957=CARTESIAN_POINT('',(13.9714037445473,37.53,-5.33144828123002));
#36958=CARTESIAN_POINT('',(10.6127493678758,38.2341789260845,-3.29608808746435));
#36959=CARTESIAN_POINT('',(12.2041262243426,37.53,-4.65706016176646));
#36960=CARTESIAN_POINT('',(6.10206311217132,37.53,-2.32853008088323));
#36961=CARTESIAN_POINT('',(12.2564275888243,37.6995434345929,-4.49554999076345));
#36962=CARTESIAN_POINT('',(14.8720022673282,37.2481324154382,-5.97680680020517));
#36963=CARTESIAN_POINT('',(12.3305248094966,38.773516735981,-3.3743143706665));
#36964=CARTESIAN_POINT('',(11.5782288391921,38.6447816854218,-3.22502994327357));
#36965=CARTESIAN_POINT('Origin',(12.2041262243426,37.03,-4.65706016176646));
#36966=CARTESIAN_POINT('',(13.9714037445473,64.47,-5.33144828123002));
#36967=CARTESIAN_POINT('',(13.9714037445473,37.03,-5.33144828123002));
#36968=CARTESIAN_POINT('',(12.2041262243426,64.47,-4.65706016176646));
#36969=CARTESIAN_POINT('',(6.10206311217132,64.47,-2.32853008088323));
#36970=CARTESIAN_POINT('',(12.2041262243426,37.03,-4.65706016176646));
#36971=CARTESIAN_POINT('Origin',(13.9714037445473,37.03,-5.33144828123002));
#36972=CARTESIAN_POINT('',(14.4379449459854,64.5678155074499,-5.6141744220185));
#36973=CARTESIAN_POINT('',(14.4379449459854,37.03,-5.6141744220185));
#36974=CARTESIAN_POINT('',(8.53723504499474,63.3306666093445,-2.03831674197418));
#36975=CARTESIAN_POINT('Origin',(3.92630159633414,37.28,-5.22531169760465));
#36976=CARTESIAN_POINT('',(9.69653989065521,37.4321844925501,-12.0809901437375));
#36977=CARTESIAN_POINT('',(9.43386642869196,37.53,-11.6028715227817));
#36978=CARTESIAN_POINT('',(7.54286651284547,38.2341789260845,-8.16087070079327));
#36979=CARTESIAN_POINT('',(8.24055326038937,37.53,-10.1351955192135));
#36980=CARTESIAN_POINT('',(4.12027663019468,37.53,-5.06759775960677));
#36981=CARTESIAN_POINT('',(8.36660265618453,37.6995434345929,-10.0214742903962));
#36982=CARTESIAN_POINT('',(9.89112836854343,37.2481324154382,-12.6120676561534));
#36983=CARTESIAN_POINT('',(8.99139054168508,38.773516735981,-9.08750437010039));
#36984=CARTESIAN_POINT('',(8.41452533393321,38.6447816854218,-8.58207227843647));
#36985=CARTESIAN_POINT('Origin',(8.24055326038937,37.03,-10.1351955192135));
#36986=CARTESIAN_POINT('',(9.43386642869196,64.47,-11.6028715227817));
#36987=CARTESIAN_POINT('',(9.43386642869196,37.03,-11.6028715227817));
#36988=CARTESIAN_POINT('',(8.24055326038937,64.47,-10.1351955192135));
#36989=CARTESIAN_POINT('',(4.12027663019468,64.47,-5.06759775960677));
#36990=CARTESIAN_POINT('',(8.24055326038937,37.03,-10.1351955192135));
#36991=CARTESIAN_POINT('Origin',(9.43386642869196,37.03,-11.6028715227817));
#36992=CARTESIAN_POINT('',(9.69653989065521,64.5678155074499,-12.0809901437375));
#36993=CARTESIAN_POINT('',(9.69653989065521,37.03,-12.0809901437375));
#36994=CARTESIAN_POINT('',(6.37430405605713,63.3306666093445,-6.03385160200617));
#36995=CARTESIAN_POINT('Origin',(0.78762107654243,37.28,-6.48840347098469));
#36996=CARTESIAN_POINT('',(2.35695480224784,37.4321844925501,-15.3107143126737));
#36997=CARTESIAN_POINT('',(2.36853222176556,37.53,-14.765314709922));
#36998=CARTESIAN_POINT('',(2.45187866708248,38.2341789260845,-10.8389546003098));
#36999=CARTESIAN_POINT('',(2.0689307051291,37.53,-12.8976134221558));
#37000=CARTESIAN_POINT('',(1.03446535256455,37.53,-6.44880671107791));
#37001=CARTESIAN_POINT('',(2.23495329842808,37.6995434345929,-12.862152646948));
#37002=CARTESIAN_POINT('',(2.25993461117485,37.2481324154382,-15.8679351687486));
#37003=CARTESIAN_POINT('',(3.24302043939622,38.773516735981,-12.3657049123516));
#37004=CARTESIAN_POINT('',(2.99615656075565,38.6447816854218,-11.6395552772068));
#37005=CARTESIAN_POINT('Origin',(2.0689307051291,37.03,-12.8976134221558));
#37006=CARTESIAN_POINT('',(2.36853222176556,64.47,-14.765314709922));
#37007=CARTESIAN_POINT('',(2.36853222176556,37.03,-14.765314709922));
#37008=CARTESIAN_POINT('',(2.0689307051291,64.47,-12.8976134221558));
#37009=CARTESIAN_POINT('',(1.03446535256455,64.47,-6.44880671107791));
#37010=CARTESIAN_POINT('',(2.0689307051291,37.03,-12.8976134221558));
#37011=CARTESIAN_POINT('Origin',(2.36853222176556,37.03,-14.765314709922));
#37012=CARTESIAN_POINT('',(2.35695480224784,64.5678155074499,-15.3107143126737));
#37013=CARTESIAN_POINT('',(2.35695480224784,37.03,-15.3107143126737));
#37014=CARTESIAN_POINT('',(2.50338344298858,63.3306666093445,-8.41262079803134));
#37015=CARTESIAN_POINT('Origin',(-0.937421834860655,64.72,-7.42225411486777));
#37016=CARTESIAN_POINT('',(-2.36853222176555,64.47,-14.765314709922));
#37017=CARTESIAN_POINT('',(-2.4882091813496,63.4588711803305,-9.12746370903454));
#37018=CARTESIAN_POINT('',(-2.0689307051291,64.47,-12.8976134221558));
#37019=CARTESIAN_POINT('',(-1.18426611088278,64.47,-7.38265735496099));
#37020=CARTESIAN_POINT('',(-1.57931400691349,64.97,-13.0021906807592));
#37021=CARTESIAN_POINT('',(-8.72557394122276,57.6721893244721,-11.4758206122532));
#37022=CARTESIAN_POINT('',(-0.690577558838534,64.97,-7.46185087477454));
#37023=CARTESIAN_POINT('Origin',(0.,64.97,0.));
#37024=CARTESIAN_POINT('',(-3.38082377665168,64.97,-12.617406105901));
#37025=CARTESIAN_POINT('',(-3.38082377665168,64.97,-12.617406105901));
#37026=CARTESIAN_POINT('',(-5.13336928983992,64.97,-12.0498844378435));
#37027=CARTESIAN_POINT('',(-4.65706016176646,64.97,-12.2041262243426));
#37028=CARTESIAN_POINT('',(-6.34896741059669,64.97,-15.2354376384622));
#37029=CARTESIAN_POINT('',(-2.79567366841787,64.97,-5.92380243612285));
#37030=CARTESIAN_POINT('',(-6.39533953317998,64.97,-15.2807225748869));
#37031=CARTESIAN_POINT('',(-6.39533953317998,64.97,-15.2807225748869));
#37032=CARTESIAN_POINT('',(-6.86159254803069,64.97,-15.6651937101241));
#37033=CARTESIAN_POINT('',(-6.86159254803069,64.97,-15.6651937101241));
#37034=CARTESIAN_POINT('',(-7.37084445728623,64.97,-16.0251680583905));
#37035=CARTESIAN_POINT('',(-7.37084445728623,64.97,-16.0251680583905));
#37036=CARTESIAN_POINT('',(-7.91980289947518,64.97,-16.3598414208564));
#37037=CARTESIAN_POINT('',(-7.91980289947518,64.97,-16.3598414208564));
#37038=CARTESIAN_POINT('',(-8.50589256852587,64.97,-16.6681291028841));
#37039=CARTESIAN_POINT('',(-8.50589256852587,64.97,-16.6681291028841));
#37040=CARTESIAN_POINT('',(-9.12693289567173,64.97,-16.9487933469585));
#37041=CARTESIAN_POINT('',(-9.12693289567173,64.97,-16.9487933469585));
#37042=CARTESIAN_POINT('',(-9.37699528855417,64.97,-16.8117357628067));
#37043=CARTESIAN_POINT('',(-9.37699528855417,64.97,-16.8117357628067));
#37044=CARTESIAN_POINT('',(-9.62500000000001,64.97,-16.6709890228504));
#37045=CARTESIAN_POINT('',(-9.62500000000001,64.97,-16.6709890228504));
#37046=CARTESIAN_POINT('',(-9.87089260802487,64.97,-16.5265840124582));
#37047=CARTESIAN_POINT('',(-9.87089260802487,64.97,-16.5265840124582));
#37048=CARTESIAN_POINT('',(-10.1146191541229,64.97,-16.3785524197668));
#37049=CARTESIAN_POINT('',(-10.1146191541229,64.97,-16.3785524197668));
#37050=CARTESIAN_POINT('',(-10.1820769523934,64.97,-15.7003835976467));
#37051=CARTESIAN_POINT('',(-10.1820769523934,64.97,-15.7003835976467));
#37052=CARTESIAN_POINT('',(-10.208136822609,64.97,-15.0386712143394));
#37053=CARTESIAN_POINT('',(-10.208136822609,64.97,-15.0386712143394));
#37054=CARTESIAN_POINT('',(-10.192780409838,64.97,-14.3959225765489));
#37055=CARTESIAN_POINT('',(-10.192780409838,64.97,-14.3959225765489));
#37056=CARTESIAN_POINT('',(-10.1356594341564,64.97,-13.7749103120746));
#37057=CARTESIAN_POINT('',(-10.1356594341564,64.97,-13.7749103120746));
#37058=CARTESIAN_POINT('',(-10.0358241714444,64.97,-13.1788877890042));
#37059=CARTESIAN_POINT('',(-7.86882139091927,64.97,-10.47057043093));
#37060=CARTESIAN_POINT('',(-4.32898314662489,64.97,-6.11686363738662));
#37061=CARTESIAN_POINT('',(-9.23658232924928,64.97,-9.23658232924928));
#37062=CARTESIAN_POINT('',(-9.23658232924928,64.97,-9.23658232924928));
#37063=CARTESIAN_POINT('',(-10.47057043093,64.97,-7.86882139091926));
#37064=CARTESIAN_POINT('',(-10.1351955192135,64.97,-8.24055326038937));
#37065=CARTESIAN_POINT('',(-13.1160858846074,64.97,-10.0197923273836));
#37066=CARTESIAN_POINT('',(-5.38302563560254,64.97,-3.73232656247359));
#37067=CARTESIAN_POINT('',(-13.1788877890042,64.97,-10.0358241714444));
#37068=CARTESIAN_POINT('',(-13.1788877890042,64.97,-10.0358241714444));
#37069=CARTESIAN_POINT('',(-13.7749103120746,64.97,-10.1356594341564));
#37070=CARTESIAN_POINT('',(-13.7749103120746,64.97,-10.1356594341564));
#37071=CARTESIAN_POINT('',(-14.3959225765489,64.97,-10.192780409838));
#37072=CARTESIAN_POINT('',(-14.3959225765489,64.97,-10.192780409838));
#37073=CARTESIAN_POINT('',(-15.0386712143394,64.97,-10.208136822609));
#37074=CARTESIAN_POINT('',(-15.0386712143394,64.97,-10.208136822609));
#37075=CARTESIAN_POINT('',(-15.7003835976467,64.97,-10.1820769523934));
#37076=CARTESIAN_POINT('',(-15.7003835976467,64.97,-10.1820769523934));
#37077=CARTESIAN_POINT('',(-16.3785524197668,64.97,-10.1146191541229));
#37078=CARTESIAN_POINT('',(-16.3785524197668,64.97,-10.1146191541229));
#37079=CARTESIAN_POINT('',(-16.5265840124582,64.97,-9.87089260802485));
#37080=CARTESIAN_POINT('',(-16.5265840124582,64.97,-9.87089260802485));
#37081=CARTESIAN_POINT('',(-16.6709890228504,64.97,-9.625));
#37082=CARTESIAN_POINT('',(-16.6709890228504,64.97,-9.625));
#37083=CARTESIAN_POINT('',(-16.8117357628067,64.97,-9.37699528855417));
#37084=CARTESIAN_POINT('',(-16.8117357628067,64.97,-9.37699528855417));
#37085=CARTESIAN_POINT('',(-16.9487933469585,64.97,-9.12693289567173));
#37086=CARTESIAN_POINT('',(-16.9487933469585,64.97,-9.12693289567173));
#37087=CARTESIAN_POINT('',(-16.6681291028841,64.97,-8.50589256852587));
#37088=CARTESIAN_POINT('',(-16.6681291028841,64.97,-8.50589256852587));
#37089=CARTESIAN_POINT('',(-16.3598414208564,64.97,-7.91980289947518));
#37090=CARTESIAN_POINT('',(-16.3598414208564,64.97,-7.91980289947518));
#37091=CARTESIAN_POINT('',(-16.0251680583905,64.97,-7.37084445728622));
#37092=CARTESIAN_POINT('',(-16.0251680583905,64.97,-7.37084445728622));
#37093=CARTESIAN_POINT('',(-15.6651937101241,64.97,-6.86159254803069));
#37094=CARTESIAN_POINT('',(-15.6651937101241,64.97,-6.86159254803069));
#37095=CARTESIAN_POINT('',(-15.2807225748869,64.97,-6.39533953317997));
#37096=CARTESIAN_POINT('',(-12.0498844378435,64.97,-5.13336928983991));
#37097=CARTESIAN_POINT('',(-6.80744119622516,64.97,-3.13286772814966));
#37098=CARTESIAN_POINT('',(-12.617406105901,64.97,-3.38082377665168));
#37099=CARTESIAN_POINT('',(-12.617406105901,64.97,-3.38082377665168));
#37100=CARTESIAN_POINT('',(-13.0021906807592,64.97,-1.57931400691349));
#37101=CARTESIAN_POINT('',(-12.8976134221558,64.97,-2.0689307051291));
#37102=CARTESIAN_POINT('',(-16.3687597379803,64.97,-2.11935175385489));
#37103=CARTESIAN_POINT('',(-6.52800023089146,64.97,-0.540776800520311));
#37104=CARTESIAN_POINT('',(-16.4311637046244,64.97,-2.10183478588267));
#37105=CARTESIAN_POINT('',(-16.4311637046244,64.97,-2.10183478588267));
#37106=CARTESIAN_POINT('',(-16.997251982187,64.97,-1.89028339804949));
#37107=CARTESIAN_POINT('',(-16.997251982187,64.97,-1.89028339804949));
#37108=CARTESIAN_POINT('',(-17.5636248671243,64.97,-1.62924548184168));
#37109=CARTESIAN_POINT('',(-17.5636248671243,64.97,-1.62924548184168));
#37110=CARTESIAN_POINT('',(-18.1279397220842,64.97,-1.32117020651705));
#37111=CARTESIAN_POINT('',(-18.1279397220842,64.97,-1.32117020651705));
#37112=CARTESIAN_POINT('',(-18.6879695209193,64.97,-0.967745505237385));
#37113=CARTESIAN_POINT('',(-18.6879695209193,64.97,-0.967745505237385));
#37114=CARTESIAN_POINT('',(-19.2415520497946,64.97,-0.570240927191679));
#37115=CARTESIAN_POINT('',(-19.2415520497946,64.97,-0.570240927191679));
#37116=CARTESIAN_POINT('',(-19.247887896579,64.97,-0.285151750348431));
#37117=CARTESIAN_POINT('',(-19.247887896579,64.97,-0.285151750348431));
#37118=CARTESIAN_POINT('',(-19.25,64.97,2.22044604925031E-15));
#37119=CARTESIAN_POINT('',(-19.25,64.97,2.35744508835865E-15));
#37120=CARTESIAN_POINT('',(-19.247887896579,64.97,0.285151750348436));
#37121=CARTESIAN_POINT('',(-19.247887896579,64.97,0.285151750348435));
#37122=CARTESIAN_POINT('',(-19.2415520497946,64.97,0.570240927191683));
#37123=CARTESIAN_POINT('',(-19.2415520497946,64.97,0.570240927191683));
#37124=CARTESIAN_POINT('',(-18.6879695209193,64.97,0.96774550523739));
#37125=CARTESIAN_POINT('',(-18.6879695209193,64.97,0.96774550523739));
#37126=CARTESIAN_POINT('',(-18.1279397220842,64.97,1.32117020651705));
#37127=CARTESIAN_POINT('',(-18.1279397220842,64.97,1.32117020651705));
#37128=CARTESIAN_POINT('',(-17.5636248671243,64.97,1.62924548184169));
#37129=CARTESIAN_POINT('',(-17.5636248671243,64.97,1.62924548184169));
#37130=CARTESIAN_POINT('',(-16.997251982187,64.97,1.89028339804949));
#37131=CARTESIAN_POINT('',(-16.997251982187,64.97,1.8902833980495));
#37132=CARTESIAN_POINT('',(-16.4311637046244,64.97,2.10183478588268));
#37133=CARTESIAN_POINT('',(-13.0021906807592,64.97,1.57931400691349));
#37134=CARTESIAN_POINT('',(-7.46185087477454,64.97,0.690577558838538));
#37135=CARTESIAN_POINT('',(-12.617406105901,64.97,3.38082377665168));
#37136=CARTESIAN_POINT('',(-12.617406105901,64.97,3.38082377665168));
#37137=CARTESIAN_POINT('',(-12.0498844378435,64.97,5.13336928983991));
#37138=CARTESIAN_POINT('',(-12.2041262243426,64.97,4.65706016176645));
#37139=CARTESIAN_POINT('',(-15.2354376384623,64.97,6.34896741059668));
#37140=CARTESIAN_POINT('',(-5.92380243612285,64.97,2.79567366841787));
#37141=CARTESIAN_POINT('',(-15.2807225748869,64.97,6.39533953317997));
#37142=CARTESIAN_POINT('',(-15.2807225748869,64.97,6.39533953317997));
#37143=CARTESIAN_POINT('',(-15.6651937101241,64.97,6.86159254803069));
#37144=CARTESIAN_POINT('',(-15.6651937101241,64.97,6.86159254803069));
#37145=CARTESIAN_POINT('',(-16.0251680583905,64.97,7.37084445728621));
#37146=CARTESIAN_POINT('',(-16.0251680583905,64.97,7.37084445728621));
#37147=CARTESIAN_POINT('',(-16.3598414208564,64.97,7.91980289947518));
#37148=CARTESIAN_POINT('',(-16.3598414208564,64.97,7.91980289947518));
#37149=CARTESIAN_POINT('',(-16.6681291028841,64.97,8.50589256852586));
#37150=CARTESIAN_POINT('',(-16.6681291028841,64.97,8.50589256852586));
#37151=CARTESIAN_POINT('',(-16.9487933469585,64.97,9.12693289567173));
#37152=CARTESIAN_POINT('',(-16.9487933469585,64.97,9.12693289567172));
#37153=CARTESIAN_POINT('',(-16.8117357628067,64.97,9.37699528855417));
#37154=CARTESIAN_POINT('',(-16.8117357628067,64.97,9.37699528855417));
#37155=CARTESIAN_POINT('',(-16.6709890228504,64.97,9.625));
#37156=CARTESIAN_POINT('',(-16.6709890228504,64.97,9.625));
#37157=CARTESIAN_POINT('',(-16.5265840124582,64.97,9.87089260802485));
#37158=CARTESIAN_POINT('',(-16.5265840124582,64.97,9.87089260802485));
#37159=CARTESIAN_POINT('',(-16.3785524197668,64.97,10.1146191541229));
#37160=CARTESIAN_POINT('',(-16.3785524197668,64.97,10.1146191541229));
#37161=CARTESIAN_POINT('',(-15.7003835976467,64.97,10.1820769523934));
#37162=CARTESIAN_POINT('',(-15.7003835976467,64.97,10.1820769523934));
#37163=CARTESIAN_POINT('',(-15.0386712143394,64.97,10.208136822609));
#37164=CARTESIAN_POINT('',(-15.0386712143394,64.97,10.208136822609));
#37165=CARTESIAN_POINT('',(-14.3959225765489,64.97,10.192780409838));
#37166=CARTESIAN_POINT('',(-14.3959225765489,64.97,10.192780409838));
#37167=CARTESIAN_POINT('',(-13.7749103120746,64.97,10.1356594341564));
#37168=CARTESIAN_POINT('',(-13.7749103120746,64.97,10.1356594341564));
#37169=CARTESIAN_POINT('',(-13.1788877890042,64.97,10.0358241714444));
#37170=CARTESIAN_POINT('',(-10.47057043093,64.97,7.86882139091926));
#37171=CARTESIAN_POINT('',(-6.11686363738663,64.97,4.32898314662489));
#37172=CARTESIAN_POINT('',(-9.23658232924928,64.97,9.23658232924927));
#37173=CARTESIAN_POINT('',(-9.23658232924928,64.97,9.23658232924928));
#37174=CARTESIAN_POINT('',(-7.86882139091926,64.97,10.47057043093));
#37175=CARTESIAN_POINT('',(-8.24055326038936,64.97,10.1351955192135));
#37176=CARTESIAN_POINT('',(-10.0197923273836,64.97,13.1160858846074));
#37177=CARTESIAN_POINT('',(-3.73232656247359,64.97,5.38302563560253));
#37178=CARTESIAN_POINT('',(-10.0358241714444,64.97,13.1788877890042));
#37179=CARTESIAN_POINT('',(-10.0358241714444,64.97,13.1788877890042));
#37180=CARTESIAN_POINT('',(-10.1356594341564,64.97,13.7749103120746));
#37181=CARTESIAN_POINT('',(-10.1356594341564,64.97,13.7749103120746));
#37182=CARTESIAN_POINT('',(-10.192780409838,64.97,14.3959225765489));
#37183=CARTESIAN_POINT('',(-10.192780409838,64.97,14.3959225765489));
#37184=CARTESIAN_POINT('',(-10.208136822609,64.97,15.0386712143394));
#37185=CARTESIAN_POINT('',(-10.208136822609,64.97,15.0386712143394));
#37186=CARTESIAN_POINT('',(-10.1820769523934,64.97,15.7003835976467));
#37187=CARTESIAN_POINT('',(-10.1820769523934,64.97,15.7003835976467));
#37188=CARTESIAN_POINT('',(-10.1146191541229,64.97,16.3785524197668));
#37189=CARTESIAN_POINT('',(-10.1146191541229,64.97,16.3785524197668));
#37190=CARTESIAN_POINT('',(-9.87089260802485,64.97,16.5265840124582));
#37191=CARTESIAN_POINT('',(-9.87089260802485,64.97,16.5265840124582));
#37192=CARTESIAN_POINT('',(-9.625,64.97,16.6709890228504));
#37193=CARTESIAN_POINT('',(-9.625,64.97,16.6709890228504));
#37194=CARTESIAN_POINT('',(-9.37699528855417,64.97,16.8117357628067));
#37195=CARTESIAN_POINT('',(-9.37699528855417,64.97,16.8117357628067));
#37196=CARTESIAN_POINT('',(-9.12693289567172,64.97,16.9487933469585));
#37197=CARTESIAN_POINT('',(-9.12693289567172,64.97,16.9487933469585));
#37198=CARTESIAN_POINT('',(-8.50589256852586,64.97,16.6681291028841));
#37199=CARTESIAN_POINT('',(-8.50589256852586,64.97,16.6681291028841));
#37200=CARTESIAN_POINT('',(-7.91980289947517,64.97,16.3598414208564));
#37201=CARTESIAN_POINT('',(-7.91980289947517,64.97,16.3598414208564));
#37202=CARTESIAN_POINT('',(-7.37084445728621,64.97,16.0251680583905));
#37203=CARTESIAN_POINT('',(-7.37084445728621,64.97,16.0251680583905));
#37204=CARTESIAN_POINT('',(-6.86159254803068,64.97,15.6651937101241));
#37205=CARTESIAN_POINT('',(-6.86159254803068,64.97,15.6651937101241));
#37206=CARTESIAN_POINT('',(-6.39533953317997,64.97,15.2807225748869));
#37207=CARTESIAN_POINT('',(-5.13336928983991,64.97,12.0498844378435));
#37208=CARTESIAN_POINT('',(-3.13286772814965,64.97,6.80744119622516));
#37209=CARTESIAN_POINT('',(-3.38082377665168,64.97,12.617406105901));
#37210=CARTESIAN_POINT('',(-3.38082377665168,64.97,12.617406105901));
#37211=CARTESIAN_POINT('',(-1.57931400691349,64.97,13.0021906807592));
#37212=CARTESIAN_POINT('',(-2.0689307051291,64.97,12.8976134221558));
#37213=CARTESIAN_POINT('',(-2.11935175385489,64.97,16.3687597379803));
#37214=CARTESIAN_POINT('',(-0.540776800520307,64.97,6.52800023089147));
#37215=CARTESIAN_POINT('',(-2.10183478588267,64.97,16.4311637046244));
#37216=CARTESIAN_POINT('',(-2.10183478588267,64.97,16.4311637046244));
#37217=CARTESIAN_POINT('',(-1.8902833980495,64.97,16.997251982187));
#37218=CARTESIAN_POINT('',(-1.8902833980495,64.97,16.997251982187));
#37219=CARTESIAN_POINT('',(-1.62924548184168,64.97,17.5636248671243));
#37220=CARTESIAN_POINT('',(-1.62924548184168,64.97,17.5636248671243));
#37221=CARTESIAN_POINT('',(-1.32117020651705,64.97,18.1279397220841));
#37222=CARTESIAN_POINT('',(-1.32117020651705,64.97,18.1279397220842));
#37223=CARTESIAN_POINT('',(-0.967745505237382,64.97,18.6879695209193));
#37224=CARTESIAN_POINT('',(-0.967745505237382,64.97,18.6879695209193));
#37225=CARTESIAN_POINT('',(-0.57024092719168,64.97,19.2415520497946));
#37226=CARTESIAN_POINT('',(-0.57024092719168,64.97,19.2415520497946));
#37227=CARTESIAN_POINT('',(-0.285151750348432,64.97,19.247887896579));
#37228=CARTESIAN_POINT('',(-0.285151750348432,64.97,19.247887896579));
#37229=CARTESIAN_POINT('',(1.11022302462516E-15,64.97,19.25));
#37230=CARTESIAN_POINT('',(1.17872254417933E-15,64.97,19.25));
#37231=CARTESIAN_POINT('',(0.285151750348434,64.97,19.247887896579));
#37232=CARTESIAN_POINT('',(0.285151750348434,64.97,19.247887896579));
#37233=CARTESIAN_POINT('',(0.570240927191682,64.97,19.2415520497946));
#37234=CARTESIAN_POINT('',(0.570240927191682,64.97,19.2415520497946));
#37235=CARTESIAN_POINT('',(0.967745505237384,64.97,18.6879695209193));
#37236=CARTESIAN_POINT('',(0.967745505237385,64.97,18.6879695209193));
#37237=CARTESIAN_POINT('',(1.32117020651705,64.97,18.1279397220841));
#37238=CARTESIAN_POINT('',(1.32117020651705,64.97,18.1279397220842));
#37239=CARTESIAN_POINT('',(1.62924548184168,64.97,17.5636248671243));
#37240=CARTESIAN_POINT('',(1.62924548184168,64.97,17.5636248671243));
#37241=CARTESIAN_POINT('',(1.8902833980495,64.97,16.997251982187));
#37242=CARTESIAN_POINT('',(1.8902833980495,64.97,16.997251982187));
#37243=CARTESIAN_POINT('',(2.10183478588268,64.97,16.4311637046244));
#37244=CARTESIAN_POINT('',(1.57931400691349,64.97,13.0021906807592));
#37245=CARTESIAN_POINT('',(0.690577558838536,64.97,7.46185087477454));
#37246=CARTESIAN_POINT('',(3.38082377665168,64.97,12.617406105901));
#37247=CARTESIAN_POINT('',(3.38082377665168,64.97,12.617406105901));
#37248=CARTESIAN_POINT('',(5.13336928983992,64.97,12.0498844378435));
#37249=CARTESIAN_POINT('',(4.65706016176646,64.97,12.2041262243426));
#37250=CARTESIAN_POINT('',(6.34896741059669,64.97,15.2354376384623));
#37251=CARTESIAN_POINT('',(2.79567366841787,64.97,5.92380243612285));
#37252=CARTESIAN_POINT('',(6.39533953317997,64.97,15.2807225748869));
#37253=CARTESIAN_POINT('',(6.39533953317997,64.97,15.2807225748869));
#37254=CARTESIAN_POINT('',(6.86159254803069,64.97,15.6651937101241));
#37255=CARTESIAN_POINT('',(6.86159254803069,64.97,15.6651937101241));
#37256=CARTESIAN_POINT('',(7.37084445728622,64.97,16.0251680583905));
#37257=CARTESIAN_POINT('',(7.37084445728622,64.97,16.0251680583905));
#37258=CARTESIAN_POINT('',(7.91980289947518,64.97,16.3598414208564));
#37259=CARTESIAN_POINT('',(7.91980289947518,64.97,16.3598414208564));
#37260=CARTESIAN_POINT('',(8.50589256852587,64.97,16.6681291028841));
#37261=CARTESIAN_POINT('',(8.50589256852587,64.97,16.6681291028841));
#37262=CARTESIAN_POINT('',(9.12693289567173,64.97,16.9487933469585));
#37263=CARTESIAN_POINT('',(9.12693289567173,64.97,16.9487933469585));
#37264=CARTESIAN_POINT('',(9.37699528855417,64.97,16.8117357628067));
#37265=CARTESIAN_POINT('',(9.37699528855417,64.97,16.8117357628067));
#37266=CARTESIAN_POINT('',(9.625,64.97,16.6709890228504));
#37267=CARTESIAN_POINT('',(9.625,64.97,16.6709890228504));
#37268=CARTESIAN_POINT('',(9.87089260802485,64.97,16.5265840124582));
#37269=CARTESIAN_POINT('',(9.87089260802485,64.97,16.5265840124582));
#37270=CARTESIAN_POINT('',(10.1146191541229,64.97,16.3785524197668));
#37271=CARTESIAN_POINT('',(10.1146191541229,64.97,16.3785524197668));
#37272=CARTESIAN_POINT('',(10.1820769523934,64.97,15.7003835976467));
#37273=CARTESIAN_POINT('',(10.1820769523934,64.97,15.7003835976467));
#37274=CARTESIAN_POINT('',(10.208136822609,64.97,15.0386712143394));
#37275=CARTESIAN_POINT('',(10.208136822609,64.97,15.0386712143394));
#37276=CARTESIAN_POINT('',(10.192780409838,64.97,14.3959225765489));
#37277=CARTESIAN_POINT('',(10.192780409838,64.97,14.3959225765489));
#37278=CARTESIAN_POINT('',(10.1356594341564,64.97,13.7749103120746));
#37279=CARTESIAN_POINT('',(10.1356594341564,64.97,13.7749103120746));
#37280=CARTESIAN_POINT('',(10.0358241714444,64.97,13.1788877890042));
#37281=CARTESIAN_POINT('',(7.86882139091926,64.97,10.47057043093));
#37282=CARTESIAN_POINT('',(4.32898314662489,64.97,6.11686363738663));
#37283=CARTESIAN_POINT('',(9.23658232924928,64.97,9.23658232924927));
#37284=CARTESIAN_POINT('',(9.23658232924928,64.97,9.23658232924928));
#37285=CARTESIAN_POINT('',(10.47057043093,64.97,7.86882139091926));
#37286=CARTESIAN_POINT('',(10.1351955192135,64.97,8.24055326038936));
#37287=CARTESIAN_POINT('',(13.1160858846074,64.97,10.0197923273836));
#37288=CARTESIAN_POINT('',(5.38302563560253,64.97,3.73232656247359));
#37289=CARTESIAN_POINT('',(13.1788877890042,64.97,10.0358241714444));
#37290=CARTESIAN_POINT('',(13.1788877890042,64.97,10.0358241714444));
#37291=CARTESIAN_POINT('',(13.7749103120746,64.97,10.1356594341564));
#37292=CARTESIAN_POINT('',(13.7749103120746,64.97,10.1356594341564));
#37293=CARTESIAN_POINT('',(14.3959225765489,64.97,10.192780409838));
#37294=CARTESIAN_POINT('',(14.3959225765489,64.97,10.192780409838));
#37295=CARTESIAN_POINT('',(15.0386712143394,64.97,10.208136822609));
#37296=CARTESIAN_POINT('',(15.0386712143394,64.97,10.208136822609));
#37297=CARTESIAN_POINT('',(15.7003835976467,64.97,10.1820769523934));
#37298=CARTESIAN_POINT('',(15.7003835976467,64.97,10.1820769523934));
#37299=CARTESIAN_POINT('',(16.3785524197668,64.97,10.1146191541229));
#37300=CARTESIAN_POINT('',(16.3785524197668,64.97,10.1146191541229));
#37301=CARTESIAN_POINT('',(16.5265840124582,64.97,9.87089260802485));
#37302=CARTESIAN_POINT('',(16.5265840124582,64.97,9.87089260802485));
#37303=CARTESIAN_POINT('',(16.6709890228504,64.97,9.625));
#37304=CARTESIAN_POINT('',(16.6709890228504,64.97,9.625));
#37305=CARTESIAN_POINT('',(16.8117357628067,64.97,9.37699528855417));
#37306=CARTESIAN_POINT('',(16.8117357628067,64.97,9.37699528855417));
#37307=CARTESIAN_POINT('',(16.9487933469585,64.97,9.12693289567172));
#37308=CARTESIAN_POINT('',(16.9487933469585,64.97,9.12693289567172));
#37309=CARTESIAN_POINT('',(16.6681291028841,64.97,8.50589256852586));
#37310=CARTESIAN_POINT('',(16.6681291028841,64.97,8.50589256852586));
#37311=CARTESIAN_POINT('',(16.3598414208564,64.97,7.91980289947518));
#37312=CARTESIAN_POINT('',(16.3598414208564,64.97,7.91980289947517));
#37313=CARTESIAN_POINT('',(16.0251680583905,64.97,7.37084445728621));
#37314=CARTESIAN_POINT('',(16.0251680583905,64.97,7.37084445728621));
#37315=CARTESIAN_POINT('',(15.6651937101241,64.97,6.86159254803069));
#37316=CARTESIAN_POINT('',(15.6651937101241,64.97,6.86159254803069));
#37317=CARTESIAN_POINT('',(15.2807225748869,64.97,6.39533953317997));
#37318=CARTESIAN_POINT('',(12.0498844378435,64.97,5.13336928983991));
#37319=CARTESIAN_POINT('',(6.80744119622516,64.97,3.13286772814966));
#37320=CARTESIAN_POINT('',(12.617406105901,64.97,3.38082377665168));
#37321=CARTESIAN_POINT('',(12.617406105901,64.97,3.38082377665168));
#37322=CARTESIAN_POINT('',(13.0021906807592,64.97,1.57931400691349));
#37323=CARTESIAN_POINT('',(12.8976134221558,64.97,2.0689307051291));
#37324=CARTESIAN_POINT('',(16.3687597379803,64.97,2.11935175385489));
#37325=CARTESIAN_POINT('',(6.52800023089146,64.97,0.540776800520309));
#37326=CARTESIAN_POINT('',(16.4311637046244,64.97,2.10183478588267));
#37327=CARTESIAN_POINT('',(16.4311637046244,64.97,2.10183478588267));
#37328=CARTESIAN_POINT('',(16.997251982187,64.97,1.8902833980495));
#37329=CARTESIAN_POINT('',(16.997251982187,64.97,1.8902833980495));
#37330=CARTESIAN_POINT('',(17.5636248671243,64.97,1.62924548184168));
#37331=CARTESIAN_POINT('',(17.5636248671243,64.97,1.62924548184168));
#37332=CARTESIAN_POINT('',(18.1279397220841,64.97,1.32117020651705));
#37333=CARTESIAN_POINT('',(18.1279397220842,64.97,1.32117020651705));
#37334=CARTESIAN_POINT('',(18.6879695209193,64.97,0.967745505237385));
#37335=CARTESIAN_POINT('',(18.6879695209193,64.97,0.967745505237384));
#37336=CARTESIAN_POINT('',(19.2415520497946,64.97,0.570240927191681));
#37337=CARTESIAN_POINT('',(19.2415520497946,64.97,0.570240927191682));
#37338=CARTESIAN_POINT('',(19.247887896579,64.97,0.285151750348434));
#37339=CARTESIAN_POINT('',(19.247887896579,64.97,0.285151750348434));
#37340=CARTESIAN_POINT('',(19.25,64.97,0.));
#37341=CARTESIAN_POINT('',(19.25,64.97,0.));
#37342=CARTESIAN_POINT('',(19.247887896579,64.97,-0.285151750348434));
#37343=CARTESIAN_POINT('',(19.247887896579,64.97,-0.285151750348434));
#37344=CARTESIAN_POINT('',(19.2415520497946,64.97,-0.570240927191681));
#37345=CARTESIAN_POINT('',(19.2415520497946,64.97,-0.570240927191682));
#37346=CARTESIAN_POINT('',(18.6879695209193,64.97,-0.967745505237385));
#37347=CARTESIAN_POINT('',(18.6879695209193,64.97,-0.967745505237384));
#37348=CARTESIAN_POINT('',(18.1279397220841,64.97,-1.32117020651705));
#37349=CARTESIAN_POINT('',(18.1279397220842,64.97,-1.32117020651705));
#37350=CARTESIAN_POINT('',(17.5636248671243,64.97,-1.62924548184168));
#37351=CARTESIAN_POINT('',(17.5636248671243,64.97,-1.62924548184168));
#37352=CARTESIAN_POINT('',(16.997251982187,64.97,-1.8902833980495));
#37353=CARTESIAN_POINT('',(16.997251982187,64.97,-1.8902833980495));
#37354=CARTESIAN_POINT('',(16.4311637046244,64.97,-2.10183478588267));
#37355=CARTESIAN_POINT('',(13.0021906807592,64.97,-1.57931400691349));
#37356=CARTESIAN_POINT('',(7.46185087477454,64.97,-0.690577558838536));
#37357=CARTESIAN_POINT('',(12.617406105901,64.97,-3.38082377665168));
#37358=CARTESIAN_POINT('',(12.617406105901,64.97,-3.38082377665168));
#37359=CARTESIAN_POINT('',(12.0498844378435,64.97,-5.13336928983991));
#37360=CARTESIAN_POINT('',(12.2041262243426,64.97,-4.65706016176646));
#37361=CARTESIAN_POINT('',(15.2354376384623,64.97,-6.34896741059669));
#37362=CARTESIAN_POINT('',(5.92380243612284,64.97,-2.79567366841787));
#37363=CARTESIAN_POINT('',(15.2807225748869,64.97,-6.39533953317997));
#37364=CARTESIAN_POINT('',(15.2807225748869,64.97,-6.39533953317997));
#37365=CARTESIAN_POINT('',(15.6651937101241,64.97,-6.86159254803069));
#37366=CARTESIAN_POINT('',(15.6651937101241,64.97,-6.86159254803069));
#37367=CARTESIAN_POINT('',(16.0251680583905,64.97,-7.37084445728621));
#37368=CARTESIAN_POINT('',(16.0251680583905,64.97,-7.37084445728621));
#37369=CARTESIAN_POINT('',(16.3598414208564,64.97,-7.91980289947517));
#37370=CARTESIAN_POINT('',(16.3598414208564,64.97,-7.91980289947517));
#37371=CARTESIAN_POINT('',(16.6681291028841,64.97,-8.50589256852586));
#37372=CARTESIAN_POINT('',(16.6681291028841,64.97,-8.50589256852586));
#37373=CARTESIAN_POINT('',(16.9487933469585,64.97,-9.12693289567172));
#37374=CARTESIAN_POINT('',(16.9487933469585,64.97,-9.12693289567172));
#37375=CARTESIAN_POINT('',(16.8117357628067,64.97,-9.37699528855417));
#37376=CARTESIAN_POINT('',(16.8117357628067,64.97,-9.37699528855417));
#37377=CARTESIAN_POINT('',(16.6709890228504,64.97,-9.625));
#37378=CARTESIAN_POINT('',(16.6709890228504,64.97,-9.625));
#37379=CARTESIAN_POINT('',(16.5265840124582,64.97,-9.87089260802485));
#37380=CARTESIAN_POINT('',(16.5265840124582,64.97,-9.87089260802485));
#37381=CARTESIAN_POINT('',(16.3785524197668,64.97,-10.1146191541229));
#37382=CARTESIAN_POINT('',(16.3785524197668,64.97,-10.1146191541229));
#37383=CARTESIAN_POINT('',(15.7003835976467,64.97,-10.1820769523934));
#37384=CARTESIAN_POINT('',(15.7003835976467,64.97,-10.1820769523934));
#37385=CARTESIAN_POINT('',(15.0386712143394,64.97,-10.208136822609));
#37386=CARTESIAN_POINT('',(15.0386712143394,64.97,-10.208136822609));
#37387=CARTESIAN_POINT('',(14.3959225765489,64.97,-10.192780409838));
#37388=CARTESIAN_POINT('',(14.3959225765489,64.97,-10.192780409838));
#37389=CARTESIAN_POINT('',(13.7749103120746,64.97,-10.1356594341564));
#37390=CARTESIAN_POINT('',(13.7749103120746,64.97,-10.1356594341564));
#37391=CARTESIAN_POINT('',(13.1788877890042,64.97,-10.0358241714444));
#37392=CARTESIAN_POINT('',(10.47057043093,64.97,-7.86882139091926));
#37393=CARTESIAN_POINT('',(6.11686363738662,64.97,-4.32898314662489));
#37394=CARTESIAN_POINT('',(9.23658232924928,64.97,-9.23658232924928));
#37395=CARTESIAN_POINT('',(9.23658232924928,64.97,-9.23658232924928));
#37396=CARTESIAN_POINT('',(7.86882139091926,64.97,-10.47057043093));
#37397=CARTESIAN_POINT('',(8.24055326038937,64.97,-10.1351955192135));
#37398=CARTESIAN_POINT('',(10.0197923273836,64.97,-13.1160858846074));
#37399=CARTESIAN_POINT('',(3.73232656247359,64.97,-5.38302563560254));
#37400=CARTESIAN_POINT('',(10.0358241714444,64.97,-13.1788877890042));
#37401=CARTESIAN_POINT('',(10.0358241714444,64.97,-13.1788877890042));
#37402=CARTESIAN_POINT('',(10.1356594341564,64.97,-13.7749103120746));
#37403=CARTESIAN_POINT('',(10.1356594341564,64.97,-13.7749103120746));
#37404=CARTESIAN_POINT('',(10.192780409838,64.97,-14.3959225765489));
#37405=CARTESIAN_POINT('',(10.192780409838,64.97,-14.3959225765489));
#37406=CARTESIAN_POINT('',(10.208136822609,64.97,-15.0386712143394));
#37407=CARTESIAN_POINT('',(10.208136822609,64.97,-15.0386712143394));
#37408=CARTESIAN_POINT('',(10.1820769523934,64.97,-15.7003835976467));
#37409=CARTESIAN_POINT('',(10.1820769523934,64.97,-15.7003835976467));
#37410=CARTESIAN_POINT('',(10.1146191541229,64.97,-16.3785524197668));
#37411=CARTESIAN_POINT('',(10.1146191541229,64.97,-16.3785524197668));
#37412=CARTESIAN_POINT('',(9.87089260802485,64.97,-16.5265840124582));
#37413=CARTESIAN_POINT('',(9.87089260802485,64.97,-16.5265840124582));
#37414=CARTESIAN_POINT('',(9.625,64.97,-16.6709890228504));
#37415=CARTESIAN_POINT('',(9.625,64.97,-16.6709890228504));
#37416=CARTESIAN_POINT('',(9.37699528855417,64.97,-16.8117357628067));
#37417=CARTESIAN_POINT('',(9.37699528855417,64.97,-16.8117357628067));
#37418=CARTESIAN_POINT('',(9.12693289567173,64.97,-16.9487933469585));
#37419=CARTESIAN_POINT('',(9.12693289567173,64.97,-16.9487933469585));
#37420=CARTESIAN_POINT('',(8.50589256852587,64.97,-16.6681291028841));
#37421=CARTESIAN_POINT('',(8.50589256852587,64.97,-16.6681291028841));
#37422=CARTESIAN_POINT('',(7.91980289947518,64.97,-16.3598414208564));
#37423=CARTESIAN_POINT('',(7.91980289947518,64.97,-16.3598414208564));
#37424=CARTESIAN_POINT('',(7.37084445728622,64.97,-16.0251680583905));
#37425=CARTESIAN_POINT('',(7.37084445728622,64.97,-16.0251680583905));
#37426=CARTESIAN_POINT('',(6.86159254803069,64.97,-15.6651937101241));
#37427=CARTESIAN_POINT('',(6.86159254803069,64.97,-15.6651937101241));
#37428=CARTESIAN_POINT('',(6.39533953317997,64.97,-15.2807225748869));
#37429=CARTESIAN_POINT('',(5.13336928983992,64.97,-12.0498844378435));
#37430=CARTESIAN_POINT('',(3.13286772814966,64.97,-6.80744119622516));
#37431=CARTESIAN_POINT('',(3.38082377665168,64.97,-12.617406105901));
#37432=CARTESIAN_POINT('',(3.38082377665168,64.97,-12.617406105901));
#37433=CARTESIAN_POINT('',(1.57931400691349,64.97,-13.0021906807592));
#37434=CARTESIAN_POINT('',(2.0689307051291,64.97,-12.8976134221558));
#37435=CARTESIAN_POINT('',(2.11935175385489,64.97,-16.3687597379803));
#37436=CARTESIAN_POINT('',(0.540776800520309,64.97,-6.52800023089146));
#37437=CARTESIAN_POINT('',(2.10183478588268,64.97,-16.4311637046244));
#37438=CARTESIAN_POINT('',(2.10183478588268,64.97,-16.4311637046244));
#37439=CARTESIAN_POINT('',(1.8902833980495,64.97,-16.997251982187));
#37440=CARTESIAN_POINT('',(1.8902833980495,64.97,-16.997251982187));
#37441=CARTESIAN_POINT('',(1.62924548184168,64.97,-17.5636248671243));
#37442=CARTESIAN_POINT('',(1.62924548184168,64.97,-17.5636248671243));
#37443=CARTESIAN_POINT('',(1.32117020651705,64.97,-18.1279397220842));
#37444=CARTESIAN_POINT('',(1.32117020651705,64.97,-18.1279397220842));
#37445=CARTESIAN_POINT('',(0.967745505237384,64.97,-18.6879695209193));
#37446=CARTESIAN_POINT('',(0.967745505237385,64.97,-18.6879695209193));
#37447=CARTESIAN_POINT('',(0.570240927191682,64.97,-19.2415520497946));
#37448=CARTESIAN_POINT('',(0.570240927191682,64.97,-19.2415520497946));
#37449=CARTESIAN_POINT('',(0.285151750348434,64.97,-19.247887896579));
#37450=CARTESIAN_POINT('',(0.285151750348434,64.97,-19.247887896579));
#37451=CARTESIAN_POINT('',(1.11022302462516E-15,64.97,-19.25));
#37452=CARTESIAN_POINT('',(1.17872254417933E-15,64.97,-19.25));
#37453=CARTESIAN_POINT('',(-0.285151750348432,64.97,-19.247887896579));
#37454=CARTESIAN_POINT('',(-0.285151750348432,64.97,-19.247887896579));
#37455=CARTESIAN_POINT('',(-0.57024092719168,64.97,-19.2415520497946));
#37456=CARTESIAN_POINT('',(-0.57024092719168,64.97,-19.2415520497946));
#37457=CARTESIAN_POINT('',(-0.967745505237382,64.97,-18.6879695209193));
#37458=CARTESIAN_POINT('',(-0.967745505237382,64.97,-18.6879695209193));
#37459=CARTESIAN_POINT('',(-1.32117020651705,64.97,-18.1279397220842));
#37460=CARTESIAN_POINT('',(-1.32117020651705,64.97,-18.1279397220842));
#37461=CARTESIAN_POINT('',(-1.62924548184168,64.97,-17.5636248671243));
#37462=CARTESIAN_POINT('',(-1.62924548184168,64.97,-17.5636248671243));
#37463=CARTESIAN_POINT('',(-1.8902833980495,64.97,-16.997251982187));
#37464=CARTESIAN_POINT('',(-1.8902833980495,64.97,-16.997251982187));
#37465=CARTESIAN_POINT('',(-2.10183478588267,64.97,-16.4311637046244));
#37466=CARTESIAN_POINT('',(-1.04094977927525E-15,64.97,-8.5));
#37467=CARTESIAN_POINT('Origin',(0.,64.97,0.));
#37468=CARTESIAN_POINT('Origin',(0.78762107654243,64.72,-6.48840347098469));
#37469=CARTESIAN_POINT('',(2.25993461117485,64.7518675845618,-15.8679351687486));
#37470=CARTESIAN_POINT('',(4.58946667393372,61.1372984587275,-7.56900801586535));
#37471=CARTESIAN_POINT('',(9.06586927392218,57.3246773483287,-11.4031369126593));
#37472=CARTESIAN_POINT('',(3.70127502843353,62.0175738804576,-7.58981354975406));
#37473=CARTESIAN_POINT('Origin',(2.89929593438233,64.72,-6.8965715342494));
#37474=CARTESIAN_POINT('',(5.33144828123002,64.47,-13.9714037445473));
#37475=CARTESIAN_POINT('',(2.40887949353887,63.4588711803305,-9.14872003481927));
#37476=CARTESIAN_POINT('',(4.65706016176646,64.47,-12.2041262243426));
#37477=CARTESIAN_POINT('',(2.66572414061501,64.47,-6.98570187227364));
#37478=CARTESIAN_POINT('',(-1.81865838957184,57.6721893244721,-14.3011391500957));
#37479=CARTESIAN_POINT('Origin',(3.92630159633414,64.72,-5.22531169760465));
#37480=CARTESIAN_POINT('',(9.89112836854343,64.7518675845618,-12.6120676561534));
#37481=CARTESIAN_POINT('',(7.75909873738132,61.1372984587275,-4.26021988622061));
#37482=CARTESIAN_POINT('',(13.5528415549351,57.3246773483287,-5.34247161223395));
#37483=CARTESIAN_POINT('',(7.00030497589346,62.0175738804575,-4.72233382985757));
#37484=CARTESIAN_POINT('Origin',(5.95914969938874,64.72,-4.52295818048544));
#37485=CARTESIAN_POINT('',(11.6028715227817,64.47,-9.43386642869196));
#37486=CARTESIAN_POINT('',(6.66051085346965,63.4588711803305,-6.71858421549571));
#37487=CARTESIAN_POINT('',(10.1351955192135,64.47,-8.24055326038936));
#37488=CARTESIAN_POINT('',(5.80143576139085,64.47,-4.71693321434598));
#37489=CARTESIAN_POINT('',(5.57556520887294,57.6721893244721,-13.294479001825));
#37490=CARTESIAN_POINT('Origin',(6.01293277414708,64.72,-2.56210187465055));
#37491=CARTESIAN_POINT('',(14.8720022673282,64.7518675845618,-5.97680680020517));
#37492=CARTESIAN_POINT('',(8.84968656015429,61.1372984587275,0.190090721515985));
#37493=CARTESIAN_POINT('',(14.4083408861561,57.3246773483287,2.14970464227572));
#37494=CARTESIAN_POINT('',(8.42360885829113,62.0175738804575,-0.589508573860589));
#37495=CARTESIAN_POINT('Origin',(7.42225411486777,64.72,-0.937421834860657));
#37496=CARTESIAN_POINT('',(14.765314709922,64.47,-2.36853222176556));
#37497=CARTESIAN_POINT('',(9.12746370903452,63.4588711803305,-2.48820918134962));
#37498=CARTESIAN_POINT('',(12.8976134221558,64.47,-2.0689307051291));
#37499=CARTESIAN_POINT('',(7.38265735496099,64.47,-1.18426611088278));
#37500=CARTESIAN_POINT('',(11.4758206122532,57.6721893244721,-8.72557394122277));
#37501=CARTESIAN_POINT('Origin',(6.48840347098469,64.72,0.78762107654243));
#37502=CARTESIAN_POINT('',(15.8679351687486,64.7518675845618,2.25993461117485));
#37503=CARTESIAN_POINT('',(7.56900801586535,61.1372984587275,4.58946667393373));
#37504=CARTESIAN_POINT('',(11.4031369126593,57.3246773483287,9.06586927392218));
#37505=CARTESIAN_POINT('',(7.58981354975407,62.0175738804576,3.70127502843351));
#37506=CARTESIAN_POINT('Origin',(6.8965715342494,64.72,2.89929593438233));
#37507=CARTESIAN_POINT('',(13.9714037445473,64.47,5.33144828123002));
#37508=CARTESIAN_POINT('',(9.14872003481924,63.4588711803305,2.40887949353882));
#37509=CARTESIAN_POINT('',(12.2041262243426,64.47,4.65706016176646));
#37510=CARTESIAN_POINT('',(6.98570187227364,64.47,2.66572414061501));
#37511=CARTESIAN_POINT('',(14.3011391500957,57.6721893244721,-1.81865838957184));
#37512=CARTESIAN_POINT('Origin',(5.22531169760465,64.72,3.92630159633414));
#37513=CARTESIAN_POINT('',(12.6120676561534,64.7518675845618,9.89112836854343));
#37514=CARTESIAN_POINT('',(4.26021988622058,61.1372984587275,7.75909873738136));
#37515=CARTESIAN_POINT('',(5.34247161223395,57.3246773483287,13.5528415549351));
#37516=CARTESIAN_POINT('',(4.7223338298576,62.0175738804576,7.00030497589344));
#37517=CARTESIAN_POINT('Origin',(4.52295818048543,64.72,5.95914969938874));
#37518=CARTESIAN_POINT('',(9.43386642869196,64.47,11.6028715227817));
#37519=CARTESIAN_POINT('',(6.71858421549571,63.4588711803305,6.66051085346967));
#37520=CARTESIAN_POINT('',(8.24055326038937,64.47,10.1351955192135));
#37521=CARTESIAN_POINT('',(4.71693321434598,64.47,5.80143576139086));
#37522=CARTESIAN_POINT('',(13.294479001825,57.6721893244721,5.57556520887294));
#37523=CARTESIAN_POINT('Origin',(2.56210187465055,64.72,6.01293277414708));
#37524=CARTESIAN_POINT('',(5.97680680020517,64.7518675845618,14.8720022673282));
#37525=CARTESIAN_POINT('',(-0.19009072151597,61.1372984587275,8.84968656015429));
#37526=CARTESIAN_POINT('',(-2.14970464227572,57.3246773483287,14.4083408861561));
#37527=CARTESIAN_POINT('',(0.589508573860579,62.0175738804575,8.42360885829113));
#37528=CARTESIAN_POINT('Origin',(0.937421834860657,64.72,7.42225411486777));
#37529=CARTESIAN_POINT('',(2.36853222176556,64.47,14.765314709922));
#37530=CARTESIAN_POINT('',(2.4882091813496,63.4588711803305,9.12746370903455));
#37531=CARTESIAN_POINT('',(2.0689307051291,64.47,12.8976134221558));
#37532=CARTESIAN_POINT('',(1.18426611088278,64.47,7.38265735496099));
#37533=CARTESIAN_POINT('',(8.72557394122277,57.6721893244721,11.4758206122532));
#37534=CARTESIAN_POINT('Origin',(-0.787621076542428,64.72,6.48840347098469));
#37535=CARTESIAN_POINT('',(-2.25993461117485,64.7518675845618,15.8679351687486));
#37536=CARTESIAN_POINT('',(-4.58946667393372,61.1372984587275,7.56900801586535));
#37537=CARTESIAN_POINT('',(-9.06586927392218,57.3246773483287,11.4031369126593));
#37538=CARTESIAN_POINT('',(-3.70127502843353,62.0175738804576,7.58981354975406));
#37539=CARTESIAN_POINT('Origin',(-2.89929593438233,64.72,6.8965715342494));
#37540=CARTESIAN_POINT('',(-5.33144828123002,64.47,13.9714037445473));
#37541=CARTESIAN_POINT('',(-2.40887949353884,63.4588711803305,9.14872003481926));
#37542=CARTESIAN_POINT('',(-4.65706016176645,64.47,12.2041262243426));
#37543=CARTESIAN_POINT('',(-2.66572414061501,64.47,6.98570187227364));
#37544=CARTESIAN_POINT('',(1.81865838957184,57.6721893244721,14.3011391500957));
#37545=CARTESIAN_POINT('Origin',(-3.92630159633414,64.72,5.22531169760465));
#37546=CARTESIAN_POINT('',(-9.89112836854343,64.7518675845618,12.6120676561534));
#37547=CARTESIAN_POINT('',(-7.75909873738135,61.1372984587275,4.26021988622059));
#37548=CARTESIAN_POINT('',(-13.5528415549351,57.3246773483287,5.34247161223395));
#37549=CARTESIAN_POINT('',(-7.0003049758934,62.0175738804576,4.72233382985765));
#37550=CARTESIAN_POINT('Origin',(-5.95914969938874,64.72,4.52295818048543));
#37551=CARTESIAN_POINT('',(-11.6028715227817,64.47,9.43386642869196));
#37552=CARTESIAN_POINT('',(-6.66051085346952,63.4588711803304,6.71858421549571));
#37553=CARTESIAN_POINT('',(-10.1351955192135,64.47,8.24055326038937));
#37554=CARTESIAN_POINT('',(-5.80143576139086,64.47,4.71693321434598));
#37555=CARTESIAN_POINT('',(-5.57556520887294,57.6721893244721,13.294479001825));
#37556=CARTESIAN_POINT('Origin',(-6.01293277414708,64.72,2.56210187465055));
#37557=CARTESIAN_POINT('',(-14.8720022673282,64.7518675845618,5.97680680020517));
#37558=CARTESIAN_POINT('',(-8.84968656015429,61.1372984587275,-0.190090721515974));
#37559=CARTESIAN_POINT('',(-14.4083408861561,57.3246773483287,-2.14970464227572));
#37560=CARTESIAN_POINT('',(-8.42360885829112,62.0175738804576,0.589508573860645));
#37561=CARTESIAN_POINT('Origin',(-7.42225411486777,64.72,0.937421834860659));
#37562=CARTESIAN_POINT('',(-14.765314709922,64.47,2.36853222176556));
#37563=CARTESIAN_POINT('',(-9.12746370903443,63.4588711803304,2.48820918134967));
#37564=CARTESIAN_POINT('',(-12.8976134221558,64.47,2.0689307051291));
#37565=CARTESIAN_POINT('',(-7.38265735496099,64.47,1.18426611088278));
#37566=CARTESIAN_POINT('',(-11.4758206122532,57.6721893244721,8.72557394122277));
#37567=CARTESIAN_POINT('Origin',(-6.48840347098469,64.72,-0.787621076542431));
#37568=CARTESIAN_POINT('',(-15.8679351687486,64.7518675845618,-2.25993461117485));
#37569=CARTESIAN_POINT('',(-7.56900801586535,61.1372984587275,-4.58946667393371));
#37570=CARTESIAN_POINT('',(-11.4031369126593,57.3246773483287,-9.06586927392218));
#37571=CARTESIAN_POINT('',(-7.58981354975408,62.0175738804576,-3.70127502843348));
#37572=CARTESIAN_POINT('Origin',(-6.8965715342494,64.72,-2.89929593438234));
#37573=CARTESIAN_POINT('',(-13.9714037445473,64.47,-5.33144828123002));
#37574=CARTESIAN_POINT('',(-9.14872003481919,63.4588711803304,-2.40887949353873));
#37575=CARTESIAN_POINT('',(-12.2041262243426,64.47,-4.65706016176646));
#37576=CARTESIAN_POINT('',(-6.98570187227364,64.47,-2.66572414061501));
#37577=CARTESIAN_POINT('',(-14.3011391500957,57.6721893244721,1.81865838957184));
#37578=CARTESIAN_POINT('Origin',(-5.22531169760465,64.72,-3.92630159633413));
#37579=CARTESIAN_POINT('',(-12.6120676561534,64.7518675845618,-9.89112836854343));
#37580=CARTESIAN_POINT('',(-4.26021988622061,61.1372984587275,-7.75909873738132));
#37581=CARTESIAN_POINT('',(-5.34247161223396,57.3246773483287,-13.5528415549351));
#37582=CARTESIAN_POINT('',(-4.72233382985763,62.0175738804576,-7.00030497589342));
#37583=CARTESIAN_POINT('Origin',(-4.52295818048544,64.72,-5.95914969938874));
#37584=CARTESIAN_POINT('',(-9.43386642869197,64.47,-11.6028715227817));
#37585=CARTESIAN_POINT('',(-6.71858421549571,63.4588711803305,-6.66051085346966));
#37586=CARTESIAN_POINT('',(-8.24055326038937,64.47,-10.1351955192135));
#37587=CARTESIAN_POINT('',(-4.71693321434598,64.47,-5.80143576139086));
#37588=CARTESIAN_POINT('',(-13.294479001825,57.6721893244721,-5.57556520887294));
#37589=CARTESIAN_POINT('Origin',(-2.56210187465055,64.72,-6.01293277414708));
#37590=CARTESIAN_POINT('',(-5.97680680020517,64.7518675845618,-14.8720022673282));
#37591=CARTESIAN_POINT('',(0.190090721516171,61.1372984587273,-8.84968656015439));
#37592=CARTESIAN_POINT('',(2.14970464227572,57.3246773483287,-14.4083408861561));
#37593=CARTESIAN_POINT('',(-0.589508573860655,62.0175738804576,-8.42360885829113));
#37594=CARTESIAN_POINT('Origin',(2.,-35.,7.94));
#37595=CARTESIAN_POINT('',(2.,-35.,7.68398334199131));
#37596=CARTESIAN_POINT('',(-2.,-35.,7.68398334199131));
#37597=CARTESIAN_POINT('Origin',(0.,-35.,0.));
#37598=CARTESIAN_POINT('',(2.,-35.,5.94));
#37599=CARTESIAN_POINT('',(2.,-35.,7.94));
#37600=CARTESIAN_POINT('',(-2.,-35.,5.94));
#37601=CARTESIAN_POINT('',(-2.,-35.,5.94));
#37602=CARTESIAN_POINT('',(-2.,-35.,7.94));
#37603=CARTESIAN_POINT('Origin',(-2.,-35.,7.94));
#37604=CARTESIAN_POINT('',(-2.,-10.,7.68398334199131));
#37605=CARTESIAN_POINT('',(-2.,-9.62499999999999,7.68398334199131));
#37606=CARTESIAN_POINT('',(-2.,-10.,5.94));
#37607=CARTESIAN_POINT('',(-2.,-10.,5.94));
#37608=CARTESIAN_POINT('',(-2.,-10.,7.94));
#37609=CARTESIAN_POINT('Origin',(2.,-10.,7.94));
#37610=CARTESIAN_POINT('',(2.,-10.,7.68398334199131));
#37611=CARTESIAN_POINT('',(2.,-9.62499999999999,7.68398334199131));
#37612=CARTESIAN_POINT('',(2.,-10.,5.94));
#37613=CARTESIAN_POINT('',(2.,-10.,7.94));
#37614=CARTESIAN_POINT('',(2.,-35.,5.94));
#37615=CARTESIAN_POINT('Origin',(-2.,-10.,7.94));
#37616=CARTESIAN_POINT('Origin',(0.,-10.,0.));
#37617=CARTESIAN_POINT('',(2.,-10.,5.94));
#37618=CARTESIAN_POINT('Origin',(0.,-22.5,5.94));
#37619=CARTESIAN_POINT('Origin',(-2.0689307051291,37.03,-12.8976134221558));
#37620=CARTESIAN_POINT('',(-3.38082377665168,37.03,-12.617406105901));
#37621=CARTESIAN_POINT('',(-2.0689307051291,37.03,-12.8976134221558));
#37622=CARTESIAN_POINT('Origin',(-2.36853222176555,37.03,-14.765314709922));
#37623=CARTESIAN_POINT('',(-2.36853222176555,37.03,-14.765314709922));
#37624=CARTESIAN_POINT('Origin',(-2.35695480224783,37.03,-15.3107143126737));
#37625=CARTESIAN_POINT('Origin',(-1.8902833980495,37.03,-16.997251982187));
#37626=CARTESIAN_POINT('',(-1.8902833980495,37.03,-16.997251982187));
#37627=CARTESIAN_POINT('Origin',(-1.62924548184168,37.03,-17.5636248671243));
#37628=CARTESIAN_POINT('',(-1.62924548184168,37.03,-17.5636248671243));
#37629=CARTESIAN_POINT('Origin',(-1.32117020651705,37.03,-18.1279397220842));
#37630=CARTESIAN_POINT('',(-1.32117020651705,37.03,-18.1279397220842));
#37631=CARTESIAN_POINT('Origin',(-0.967745505237382,37.03,-18.6879695209193));
#37632=CARTESIAN_POINT('',(-0.967745505237382,37.03,-18.6879695209193));
#37633=CARTESIAN_POINT('Origin',(-0.57024092719168,37.03,-19.2415520497946));
#37634=CARTESIAN_POINT('',(-0.57024092719168,37.03,-19.2415520497946));
#37635=CARTESIAN_POINT('Origin',(-0.285151750348432,37.03,-19.247887896579));
#37636=CARTESIAN_POINT('',(-0.285151750348432,37.03,-19.247887896579));
#37637=CARTESIAN_POINT('Origin',(1.17961196366423E-15,37.03,-19.25));
#37638=CARTESIAN_POINT('',(1.17872254417933E-15,37.03,-19.25));
#37639=CARTESIAN_POINT('Origin',(0.285151750348434,37.03,-19.247887896579));
#37640=CARTESIAN_POINT('',(0.285151750348434,37.03,-19.247887896579));
#37641=CARTESIAN_POINT('Origin',(0.570240927191682,37.03,-19.2415520497946));
#37642=CARTESIAN_POINT('',(0.570240927191682,37.03,-19.2415520497946));
#37643=CARTESIAN_POINT('Origin',(0.967745505237385,37.03,-18.6879695209193));
#37644=CARTESIAN_POINT('',(0.967745505237385,37.03,-18.6879695209193));
#37645=CARTESIAN_POINT('Origin',(1.32117020651705,37.03,-18.1279397220842));
#37646=CARTESIAN_POINT('',(1.32117020651705,37.03,-18.1279397220842));
#37647=CARTESIAN_POINT('Origin',(1.62924548184168,37.03,-17.5636248671243));
#37648=CARTESIAN_POINT('',(1.62924548184168,37.03,-17.5636248671243));
#37649=CARTESIAN_POINT('Origin',(1.8902833980495,37.03,-16.997251982187));
#37650=CARTESIAN_POINT('',(1.8902833980495,37.03,-16.997251982187));
#37651=CARTESIAN_POINT('Origin',(2.10183478588268,37.03,-16.4311637046244));
#37652=CARTESIAN_POINT('',(2.10183478588268,37.03,-16.4311637046244));
#37653=CARTESIAN_POINT('Origin',(2.25993461117485,37.03,-15.8679351687486));
#37654=CARTESIAN_POINT('',(2.25993461117485,37.03,-15.8679351687486));
#37655=CARTESIAN_POINT('Origin',(2.35695480224784,37.03,-15.3107143126737));
#37656=CARTESIAN_POINT('Origin',(3.38082377665168,37.03,-12.617406105901));
#37657=CARTESIAN_POINT('',(3.38082377665168,37.03,-12.617406105901));
#37658=CARTESIAN_POINT('Origin',(4.65706016176646,37.03,-12.2041262243426));
#37659=CARTESIAN_POINT('',(4.65706016176646,37.03,-12.2041262243426));
#37660=CARTESIAN_POINT('Origin',(5.33144828123002,37.03,-13.9714037445473));
#37661=CARTESIAN_POINT('',(5.33144828123002,37.03,-13.9714037445473));
#37662=CARTESIAN_POINT('Origin',(5.61417442201851,37.03,-14.4379449459854));
#37663=CARTESIAN_POINT('Origin',(6.86159254803069,37.03,-15.6651937101241));
#37664=CARTESIAN_POINT('',(6.86159254803069,37.03,-15.6651937101241));
#37665=CARTESIAN_POINT('Origin',(7.37084445728622,37.03,-16.0251680583905));
#37666=CARTESIAN_POINT('',(7.37084445728622,37.03,-16.0251680583905));
#37667=CARTESIAN_POINT('Origin',(7.91980289947518,37.03,-16.3598414208564));
#37668=CARTESIAN_POINT('',(7.91980289947518,37.03,-16.3598414208564));
#37669=CARTESIAN_POINT('Origin',(8.50589256852587,37.03,-16.6681291028841));
#37670=CARTESIAN_POINT('',(8.50589256852587,37.03,-16.6681291028841));
#37671=CARTESIAN_POINT('Origin',(9.12693289567173,37.03,-16.9487933469585));
#37672=CARTESIAN_POINT('',(9.12693289567173,37.03,-16.9487933469585));
#37673=CARTESIAN_POINT('Origin',(9.37699528855417,37.03,-16.8117357628067));
#37674=CARTESIAN_POINT('',(9.37699528855417,37.03,-16.8117357628067));
#37675=CARTESIAN_POINT('Origin',(9.625,37.03,-16.6709890228504));
#37676=CARTESIAN_POINT('',(9.625,37.03,-16.6709890228504));
#37677=CARTESIAN_POINT('Origin',(9.87089260802485,37.03,-16.5265840124582));
#37678=CARTESIAN_POINT('',(9.87089260802485,37.03,-16.5265840124582));
#37679=CARTESIAN_POINT('Origin',(10.1146191541229,37.03,-16.3785524197668));
#37680=CARTESIAN_POINT('',(10.1146191541229,37.03,-16.3785524197668));
#37681=CARTESIAN_POINT('Origin',(10.1820769523934,37.03,-15.7003835976467));
#37682=CARTESIAN_POINT('',(10.1820769523934,37.03,-15.7003835976467));
#37683=CARTESIAN_POINT('Origin',(10.208136822609,37.03,-15.0386712143394));
#37684=CARTESIAN_POINT('',(10.208136822609,37.03,-15.0386712143394));
#37685=CARTESIAN_POINT('Origin',(10.192780409838,37.03,-14.3959225765489));
#37686=CARTESIAN_POINT('',(10.192780409838,37.03,-14.3959225765489));
#37687=CARTESIAN_POINT('Origin',(10.1356594341564,37.03,-13.7749103120746));
#37688=CARTESIAN_POINT('',(10.1356594341564,37.03,-13.7749103120746));
#37689=CARTESIAN_POINT('Origin',(10.0358241714444,37.03,-13.1788877890042));
#37690=CARTESIAN_POINT('',(10.0358241714444,37.03,-13.1788877890042));
#37691=CARTESIAN_POINT('Origin',(9.89112836854343,37.03,-12.6120676561534));
#37692=CARTESIAN_POINT('',(9.89112836854343,37.03,-12.6120676561534));
#37693=CARTESIAN_POINT('Origin',(9.69653989065521,37.03,-12.0809901437375));
#37694=CARTESIAN_POINT('Origin',(9.23658232924928,37.03,-9.23658232924928));
#37695=CARTESIAN_POINT('',(9.23658232924928,37.03,-9.23658232924928));
#37696=CARTESIAN_POINT('Origin',(10.1351955192135,37.03,-8.24055326038936));
#37697=CARTESIAN_POINT('',(10.1351955192135,37.03,-8.24055326038936));
#37698=CARTESIAN_POINT('Origin',(11.6028715227817,37.03,-9.43386642869196));
#37699=CARTESIAN_POINT('',(11.6028715227817,37.03,-9.43386642869196));
#37700=CARTESIAN_POINT('Origin',(12.0809901437375,37.03,-9.69653989065521));
#37701=CARTESIAN_POINT('Origin',(13.7749103120746,37.03,-10.1356594341564));
#37702=CARTESIAN_POINT('',(13.7749103120746,37.03,-10.1356594341564));
#37703=CARTESIAN_POINT('Origin',(14.3959225765489,37.03,-10.192780409838));
#37704=CARTESIAN_POINT('',(14.3959225765489,37.03,-10.192780409838));
#37705=CARTESIAN_POINT('Origin',(15.0386712143394,37.03,-10.208136822609));
#37706=CARTESIAN_POINT('',(15.0386712143394,37.03,-10.208136822609));
#37707=CARTESIAN_POINT('Origin',(15.7003835976467,37.03,-10.1820769523934));
#37708=CARTESIAN_POINT('',(15.7003835976467,37.03,-10.1820769523934));
#37709=CARTESIAN_POINT('Origin',(16.3785524197668,37.03,-10.1146191541229));
#37710=CARTESIAN_POINT('',(16.3785524197668,37.03,-10.1146191541229));
#37711=CARTESIAN_POINT('Origin',(16.5265840124582,37.03,-9.87089260802485));
#37712=CARTESIAN_POINT('',(16.5265840124582,37.03,-9.87089260802485));
#37713=CARTESIAN_POINT('Origin',(16.6709890228504,37.03,-9.625));
#37714=CARTESIAN_POINT('',(16.6709890228504,37.03,-9.625));
#37715=CARTESIAN_POINT('Origin',(16.8117357628067,37.03,-9.37699528855417));
#37716=CARTESIAN_POINT('',(16.8117357628067,37.03,-9.37699528855417));
#37717=CARTESIAN_POINT('Origin',(16.9487933469585,37.03,-9.12693289567172));
#37718=CARTESIAN_POINT('',(16.9487933469585,37.03,-9.12693289567172));
#37719=CARTESIAN_POINT('Origin',(16.6681291028841,37.03,-8.50589256852586));
#37720=CARTESIAN_POINT('',(16.6681291028841,37.03,-8.50589256852586));
#37721=CARTESIAN_POINT('Origin',(16.3598414208564,37.03,-7.91980289947517));
#37722=CARTESIAN_POINT('',(16.3598414208564,37.03,-7.91980289947517));
#37723=CARTESIAN_POINT('Origin',(16.0251680583905,37.03,-7.37084445728621));
#37724=CARTESIAN_POINT('',(16.0251680583905,37.03,-7.37084445728621));
#37725=CARTESIAN_POINT('Origin',(15.6651937101241,37.03,-6.86159254803069));
#37726=CARTESIAN_POINT('',(15.6651937101241,37.03,-6.86159254803069));
#37727=CARTESIAN_POINT('Origin',(15.2807225748869,37.03,-6.39533953317997));
#37728=CARTESIAN_POINT('',(15.2807225748869,37.03,-6.39533953317997));
#37729=CARTESIAN_POINT('Origin',(14.8720022673282,37.03,-5.97680680020517));
#37730=CARTESIAN_POINT('',(14.8720022673282,37.03,-5.97680680020517));
#37731=CARTESIAN_POINT('Origin',(14.4379449459854,37.03,-5.6141744220185));
#37732=CARTESIAN_POINT('Origin',(12.617406105901,37.03,-3.38082377665168));
#37733=CARTESIAN_POINT('',(12.617406105901,37.03,-3.38082377665168));
#37734=CARTESIAN_POINT('Origin',(12.8976134221558,37.03,-2.0689307051291));
#37735=CARTESIAN_POINT('',(12.8976134221558,37.03,-2.0689307051291));
#37736=CARTESIAN_POINT('Origin',(14.765314709922,37.03,-2.36853222176556));
#37737=CARTESIAN_POINT('',(14.765314709922,37.03,-2.36853222176556));
#37738=CARTESIAN_POINT('Origin',(15.3107143126737,37.03,-2.35695480224783));
#37739=CARTESIAN_POINT('Origin',(16.997251982187,37.03,-1.8902833980495));
#37740=CARTESIAN_POINT('',(16.997251982187,37.03,-1.8902833980495));
#37741=CARTESIAN_POINT('Origin',(17.5636248671243,37.03,-1.62924548184168));
#37742=CARTESIAN_POINT('',(17.5636248671243,37.03,-1.62924548184168));
#37743=CARTESIAN_POINT('Origin',(18.1279397220842,37.03,-1.32117020651705));
#37744=CARTESIAN_POINT('',(18.1279397220842,37.03,-1.32117020651705));
#37745=CARTESIAN_POINT('Origin',(18.6879695209193,37.03,-0.967745505237384));
#37746=CARTESIAN_POINT('',(18.6879695209193,37.03,-0.967745505237384));
#37747=CARTESIAN_POINT('Origin',(19.2415520497946,37.03,-0.570240927191682));
#37748=CARTESIAN_POINT('',(19.2415520497946,37.03,-0.570240927191682));
#37749=CARTESIAN_POINT('Origin',(19.247887896579,37.03,-0.285151750348434));
#37750=CARTESIAN_POINT('',(19.247887896579,37.03,-0.285151750348434));
#37751=CARTESIAN_POINT('Origin',(19.25,37.03,0.));
#37752=CARTESIAN_POINT('',(19.25,37.03,0.));
#37753=CARTESIAN_POINT('Origin',(19.247887896579,37.03,0.285151750348434));
#37754=CARTESIAN_POINT('',(19.247887896579,37.03,0.285151750348434));
#37755=CARTESIAN_POINT('Origin',(19.2415520497946,37.03,0.570240927191682));
#37756=CARTESIAN_POINT('',(19.2415520497946,37.03,0.570240927191682));
#37757=CARTESIAN_POINT('Origin',(18.6879695209193,37.03,0.967745505237384));
#37758=CARTESIAN_POINT('',(18.6879695209193,37.03,0.967745505237384));
#37759=CARTESIAN_POINT('Origin',(18.1279397220842,37.03,1.32117020651705));
#37760=CARTESIAN_POINT('',(18.1279397220842,37.03,1.32117020651705));
#37761=CARTESIAN_POINT('Origin',(17.5636248671243,37.03,1.62924548184168));
#37762=CARTESIAN_POINT('',(17.5636248671243,37.03,1.62924548184168));
#37763=CARTESIAN_POINT('Origin',(16.997251982187,37.03,1.8902833980495));
#37764=CARTESIAN_POINT('',(16.997251982187,37.03,1.8902833980495));
#37765=CARTESIAN_POINT('Origin',(16.4311637046244,37.03,2.10183478588267));
#37766=CARTESIAN_POINT('',(16.4311637046244,37.03,2.10183478588267));
#37767=CARTESIAN_POINT('Origin',(15.8679351687486,37.03,2.25993461117485));
#37768=CARTESIAN_POINT('',(15.8679351687486,37.03,2.25993461117485));
#37769=CARTESIAN_POINT('Origin',(15.3107143126737,37.03,2.35695480224783));
#37770=CARTESIAN_POINT('Origin',(12.617406105901,37.03,3.38082377665168));
#37771=CARTESIAN_POINT('',(12.617406105901,37.03,3.38082377665168));
#37772=CARTESIAN_POINT('Origin',(12.2041262243426,37.03,4.65706016176646));
#37773=CARTESIAN_POINT('',(12.2041262243426,37.03,4.65706016176646));
#37774=CARTESIAN_POINT('Origin',(13.9714037445473,37.03,5.33144828123002));
#37775=CARTESIAN_POINT('',(13.9714037445473,37.03,5.33144828123002));
#37776=CARTESIAN_POINT('Origin',(14.4379449459854,37.03,5.6141744220185));
#37777=CARTESIAN_POINT('Origin',(15.6651937101241,37.03,6.86159254803069));
#37778=CARTESIAN_POINT('',(15.6651937101241,37.03,6.86159254803069));
#37779=CARTESIAN_POINT('Origin',(16.0251680583905,37.03,7.37084445728621));
#37780=CARTESIAN_POINT('',(16.0251680583905,37.03,7.37084445728621));
#37781=CARTESIAN_POINT('Origin',(16.3598414208564,37.03,7.91980289947517));
#37782=CARTESIAN_POINT('',(16.3598414208564,37.03,7.91980289947517));
#37783=CARTESIAN_POINT('Origin',(16.6681291028841,37.03,8.50589256852586));
#37784=CARTESIAN_POINT('',(16.6681291028841,37.03,8.50589256852586));
#37785=CARTESIAN_POINT('Origin',(16.9487933469585,37.03,9.12693289567172));
#37786=CARTESIAN_POINT('',(16.9487933469585,37.03,9.12693289567172));
#37787=CARTESIAN_POINT('Origin',(16.8117357628067,37.03,9.37699528855417));
#37788=CARTESIAN_POINT('',(16.8117357628067,37.03,9.37699528855417));
#37789=CARTESIAN_POINT('Origin',(16.6709890228504,37.03,9.625));
#37790=CARTESIAN_POINT('',(16.6709890228504,37.03,9.625));
#37791=CARTESIAN_POINT('Origin',(16.5265840124582,37.03,9.87089260802485));
#37792=CARTESIAN_POINT('',(16.5265840124582,37.03,9.87089260802485));
#37793=CARTESIAN_POINT('Origin',(16.3785524197668,37.03,10.1146191541229));
#37794=CARTESIAN_POINT('',(16.3785524197668,37.03,10.1146191541229));
#37795=CARTESIAN_POINT('Origin',(15.7003835976467,37.03,10.1820769523934));
#37796=CARTESIAN_POINT('',(15.7003835976467,37.03,10.1820769523934));
#37797=CARTESIAN_POINT('Origin',(15.0386712143394,37.03,10.208136822609));
#37798=CARTESIAN_POINT('',(15.0386712143394,37.03,10.208136822609));
#37799=CARTESIAN_POINT('Origin',(14.3959225765489,37.03,10.192780409838));
#37800=CARTESIAN_POINT('',(14.3959225765489,37.03,10.192780409838));
#37801=CARTESIAN_POINT('Origin',(13.7749103120746,37.03,10.1356594341564));
#37802=CARTESIAN_POINT('',(13.7749103120746,37.03,10.1356594341564));
#37803=CARTESIAN_POINT('Origin',(13.1788877890042,37.03,10.0358241714444));
#37804=CARTESIAN_POINT('',(13.1788877890042,37.03,10.0358241714444));
#37805=CARTESIAN_POINT('Origin',(12.6120676561534,37.03,9.89112836854343));
#37806=CARTESIAN_POINT('',(12.6120676561534,37.03,9.89112836854343));
#37807=CARTESIAN_POINT('Origin',(12.0809901437375,37.03,9.69653989065521));
#37808=CARTESIAN_POINT('Origin',(9.23658232924928,37.03,9.23658232924928));
#37809=CARTESIAN_POINT('',(9.23658232924928,37.03,9.23658232924928));
#37810=CARTESIAN_POINT('Origin',(8.24055326038937,37.03,10.1351955192135));
#37811=CARTESIAN_POINT('',(8.24055326038937,37.03,10.1351955192135));
#37812=CARTESIAN_POINT('Origin',(9.43386642869196,37.03,11.6028715227817));
#37813=CARTESIAN_POINT('',(9.43386642869196,37.03,11.6028715227817));
#37814=CARTESIAN_POINT('Origin',(9.69653989065521,37.03,12.0809901437375));
#37815=CARTESIAN_POINT('Origin',(10.1356594341564,37.03,13.7749103120746));
#37816=CARTESIAN_POINT('',(10.1356594341564,37.03,13.7749103120746));
#37817=CARTESIAN_POINT('Origin',(10.192780409838,37.03,14.3959225765489));
#37818=CARTESIAN_POINT('',(10.192780409838,37.03,14.3959225765489));
#37819=CARTESIAN_POINT('Origin',(10.208136822609,37.03,15.0386712143394));
#37820=CARTESIAN_POINT('',(10.208136822609,37.03,15.0386712143394));
#37821=CARTESIAN_POINT('Origin',(10.1820769523934,37.03,15.7003835976467));
#37822=CARTESIAN_POINT('',(10.1820769523934,37.03,15.7003835976467));
#37823=CARTESIAN_POINT('Origin',(10.1146191541229,37.03,16.3785524197668));
#37824=CARTESIAN_POINT('',(10.1146191541229,37.03,16.3785524197668));
#37825=CARTESIAN_POINT('Origin',(9.87089260802485,37.03,16.5265840124582));
#37826=CARTESIAN_POINT('',(9.87089260802485,37.03,16.5265840124582));
#37827=CARTESIAN_POINT('Origin',(9.625,37.03,16.6709890228504));
#37828=CARTESIAN_POINT('',(9.625,37.03,16.6709890228504));
#37829=CARTESIAN_POINT('Origin',(9.37699528855417,37.03,16.8117357628067));
#37830=CARTESIAN_POINT('',(9.37699528855417,37.03,16.8117357628067));
#37831=CARTESIAN_POINT('Origin',(9.12693289567173,37.03,16.9487933469585));
#37832=CARTESIAN_POINT('',(9.12693289567173,37.03,16.9487933469585));
#37833=CARTESIAN_POINT('Origin',(8.50589256852587,37.03,16.6681291028841));
#37834=CARTESIAN_POINT('',(8.50589256852587,37.03,16.6681291028841));
#37835=CARTESIAN_POINT('Origin',(7.91980289947518,37.03,16.3598414208564));
#37836=CARTESIAN_POINT('',(7.91980289947518,37.03,16.3598414208564));
#37837=CARTESIAN_POINT('Origin',(7.37084445728622,37.03,16.0251680583905));
#37838=CARTESIAN_POINT('',(7.37084445728622,37.03,16.0251680583905));
#37839=CARTESIAN_POINT('Origin',(6.86159254803069,37.03,15.6651937101241));
#37840=CARTESIAN_POINT('',(6.86159254803069,37.03,15.6651937101241));
#37841=CARTESIAN_POINT('Origin',(6.39533953317997,37.03,15.2807225748869));
#37842=CARTESIAN_POINT('',(6.39533953317997,37.03,15.2807225748869));
#37843=CARTESIAN_POINT('Origin',(5.97680680020517,37.03,14.8720022673282));
#37844=CARTESIAN_POINT('',(5.97680680020517,37.03,14.8720022673282));
#37845=CARTESIAN_POINT('Origin',(5.61417442201851,37.03,14.4379449459854));
#37846=CARTESIAN_POINT('Origin',(3.38082377665168,37.03,12.617406105901));
#37847=CARTESIAN_POINT('',(3.38082377665168,37.03,12.617406105901));
#37848=CARTESIAN_POINT('Origin',(2.0689307051291,37.03,12.8976134221558));
#37849=CARTESIAN_POINT('',(2.0689307051291,37.03,12.8976134221558));
#37850=CARTESIAN_POINT('Origin',(2.36853222176556,37.03,14.765314709922));
#37851=CARTESIAN_POINT('',(2.36853222176556,37.03,14.765314709922));
#37852=CARTESIAN_POINT('Origin',(2.35695480224784,37.03,15.3107143126737));
#37853=CARTESIAN_POINT('Origin',(1.8902833980495,37.03,16.997251982187));
#37854=CARTESIAN_POINT('',(1.8902833980495,37.03,16.997251982187));
#37855=CARTESIAN_POINT('Origin',(1.62924548184168,37.03,17.5636248671243));
#37856=CARTESIAN_POINT('',(1.62924548184168,37.03,17.5636248671243));
#37857=CARTESIAN_POINT('Origin',(1.32117020651705,37.03,18.1279397220842));
#37858=CARTESIAN_POINT('',(1.32117020651705,37.03,18.1279397220842));
#37859=CARTESIAN_POINT('Origin',(0.967745505237385,37.03,18.6879695209193));
#37860=CARTESIAN_POINT('',(0.967745505237385,37.03,18.6879695209193));
#37861=CARTESIAN_POINT('Origin',(0.570240927191682,37.03,19.2415520497946));
#37862=CARTESIAN_POINT('',(0.570240927191682,37.03,19.2415520497946));
#37863=CARTESIAN_POINT('Origin',(0.285151750348434,37.03,19.247887896579));
#37864=CARTESIAN_POINT('',(0.285151750348434,37.03,19.247887896579));
#37865=CARTESIAN_POINT('Origin',(1.17961196366423E-15,37.03,19.25));
#37866=CARTESIAN_POINT('',(1.17872254417933E-15,37.03,19.25));
#37867=CARTESIAN_POINT('Origin',(-0.285151750348432,37.03,19.247887896579));
#37868=CARTESIAN_POINT('',(-0.285151750348432,37.03,19.247887896579));
#37869=CARTESIAN_POINT('Origin',(-0.57024092719168,37.03,19.2415520497946));
#37870=CARTESIAN_POINT('',(-0.57024092719168,37.03,19.2415520497946));
#37871=CARTESIAN_POINT('Origin',(-0.967745505237382,37.03,18.6879695209193));
#37872=CARTESIAN_POINT('',(-0.967745505237382,37.03,18.6879695209193));
#37873=CARTESIAN_POINT('Origin',(-1.32117020651705,37.03,18.1279397220842));
#37874=CARTESIAN_POINT('',(-1.32117020651705,37.03,18.1279397220842));
#37875=CARTESIAN_POINT('Origin',(-1.62924548184168,37.03,17.5636248671243));
#37876=CARTESIAN_POINT('',(-1.62924548184168,37.03,17.5636248671243));
#37877=CARTESIAN_POINT('Origin',(-1.8902833980495,37.03,16.997251982187));
#37878=CARTESIAN_POINT('',(-1.8902833980495,37.03,16.997251982187));
#37879=CARTESIAN_POINT('Origin',(-2.10183478588267,37.03,16.4311637046244));
#37880=CARTESIAN_POINT('',(-2.10183478588267,37.03,16.4311637046244));
#37881=CARTESIAN_POINT('Origin',(-2.25993461117485,37.03,15.8679351687486));
#37882=CARTESIAN_POINT('',(-2.25993461117485,37.03,15.8679351687486));
#37883=CARTESIAN_POINT('Origin',(-2.35695480224783,37.03,15.3107143126737));
#37884=CARTESIAN_POINT('Origin',(-3.38082377665168,37.03,12.617406105901));
#37885=CARTESIAN_POINT('',(-3.38082377665168,37.03,12.617406105901));
#37886=CARTESIAN_POINT('Origin',(-4.65706016176645,37.03,12.2041262243426));
#37887=CARTESIAN_POINT('',(-4.65706016176645,37.03,12.2041262243426));
#37888=CARTESIAN_POINT('Origin',(-5.33144828123002,37.03,13.9714037445473));
#37889=CARTESIAN_POINT('',(-5.33144828123002,37.03,13.9714037445473));
#37890=CARTESIAN_POINT('Origin',(-5.6141744220185,37.03,14.4379449459854));
#37891=CARTESIAN_POINT('Origin',(-6.86159254803068,37.03,15.6651937101241));
#37892=CARTESIAN_POINT('',(-6.86159254803068,37.03,15.6651937101241));
#37893=CARTESIAN_POINT('Origin',(-7.37084445728621,37.03,16.0251680583905));
#37894=CARTESIAN_POINT('',(-7.37084445728621,37.03,16.0251680583905));
#37895=CARTESIAN_POINT('Origin',(-7.91980289947517,37.03,16.3598414208564));
#37896=CARTESIAN_POINT('',(-7.91980289947517,37.03,16.3598414208564));
#37897=CARTESIAN_POINT('Origin',(-8.50589256852586,37.03,16.6681291028841));
#37898=CARTESIAN_POINT('',(-8.50589256852586,37.03,16.6681291028841));
#37899=CARTESIAN_POINT('Origin',(-9.12693289567172,37.03,16.9487933469585));
#37900=CARTESIAN_POINT('',(-9.12693289567172,37.03,16.9487933469585));
#37901=CARTESIAN_POINT('Origin',(-9.37699528855417,37.03,16.8117357628067));
#37902=CARTESIAN_POINT('',(-9.37699528855417,37.03,16.8117357628067));
#37903=CARTESIAN_POINT('Origin',(-9.625,37.03,16.6709890228504));
#37904=CARTESIAN_POINT('',(-9.625,37.03,16.6709890228504));
#37905=CARTESIAN_POINT('Origin',(-9.87089260802485,37.03,16.5265840124582));
#37906=CARTESIAN_POINT('',(-9.87089260802485,37.03,16.5265840124582));
#37907=CARTESIAN_POINT('Origin',(-10.1146191541229,37.03,16.3785524197668));
#37908=CARTESIAN_POINT('',(-10.1146191541229,37.03,16.3785524197668));
#37909=CARTESIAN_POINT('Origin',(-10.1820769523934,37.03,15.7003835976467));
#37910=CARTESIAN_POINT('',(-10.1820769523934,37.03,15.7003835976467));
#37911=CARTESIAN_POINT('Origin',(-10.208136822609,37.03,15.0386712143394));
#37912=CARTESIAN_POINT('',(-10.208136822609,37.03,15.0386712143394));
#37913=CARTESIAN_POINT('Origin',(-10.192780409838,37.03,14.3959225765489));
#37914=CARTESIAN_POINT('',(-10.192780409838,37.03,14.3959225765489));
#37915=CARTESIAN_POINT('Origin',(-10.1356594341564,37.03,13.7749103120746));
#37916=CARTESIAN_POINT('',(-10.1356594341564,37.03,13.7749103120746));
#37917=CARTESIAN_POINT('Origin',(-10.0358241714444,37.03,13.1788877890042));
#37918=CARTESIAN_POINT('',(-10.0358241714444,37.03,13.1788877890042));
#37919=CARTESIAN_POINT('Origin',(-9.89112836854343,37.03,12.6120676561534));
#37920=CARTESIAN_POINT('',(-9.89112836854343,37.03,12.6120676561534));
#37921=CARTESIAN_POINT('Origin',(-9.6965398906552,37.03,12.0809901437375));
#37922=CARTESIAN_POINT('Origin',(-9.23658232924928,37.03,9.23658232924928));
#37923=CARTESIAN_POINT('',(-9.23658232924928,37.03,9.23658232924928));
#37924=CARTESIAN_POINT('Origin',(-10.1351955192135,37.03,8.24055326038937));
#37925=CARTESIAN_POINT('',(-10.1351955192135,37.03,8.24055326038937));
#37926=CARTESIAN_POINT('Origin',(-11.6028715227817,37.03,9.43386642869196));
#37927=CARTESIAN_POINT('',(-11.6028715227817,37.03,9.43386642869196));
#37928=CARTESIAN_POINT('Origin',(-12.0809901437375,37.03,9.69653989065521));
#37929=CARTESIAN_POINT('Origin',(-13.7749103120746,37.03,10.1356594341564));
#37930=CARTESIAN_POINT('',(-13.7749103120746,37.03,10.1356594341564));
#37931=CARTESIAN_POINT('Origin',(-14.3959225765489,37.03,10.192780409838));
#37932=CARTESIAN_POINT('',(-14.3959225765489,37.03,10.192780409838));
#37933=CARTESIAN_POINT('Origin',(-15.0386712143394,37.03,10.208136822609));
#37934=CARTESIAN_POINT('',(-15.0386712143394,37.03,10.208136822609));
#37935=CARTESIAN_POINT('Origin',(-15.7003835976467,37.03,10.1820769523934));
#37936=CARTESIAN_POINT('',(-15.7003835976467,37.03,10.1820769523934));
#37937=CARTESIAN_POINT('Origin',(-16.3785524197668,37.03,10.1146191541229));
#37938=CARTESIAN_POINT('',(-16.3785524197668,37.03,10.1146191541229));
#37939=CARTESIAN_POINT('Origin',(-16.5265840124582,37.03,9.87089260802485));
#37940=CARTESIAN_POINT('',(-16.5265840124582,37.03,9.87089260802485));
#37941=CARTESIAN_POINT('Origin',(-16.6709890228504,37.03,9.625));
#37942=CARTESIAN_POINT('',(-16.6709890228504,37.03,9.625));
#37943=CARTESIAN_POINT('Origin',(-16.8117357628067,37.03,9.37699528855417));
#37944=CARTESIAN_POINT('',(-16.8117357628067,37.03,9.37699528855417));
#37945=CARTESIAN_POINT('Origin',(-16.9487933469585,37.03,9.12693289567172));
#37946=CARTESIAN_POINT('',(-16.9487933469585,37.03,9.12693289567172));
#37947=CARTESIAN_POINT('Origin',(-16.6681291028841,37.03,8.50589256852586));
#37948=CARTESIAN_POINT('',(-16.6681291028841,37.03,8.50589256852586));
#37949=CARTESIAN_POINT('Origin',(-16.3598414208564,37.03,7.91980289947518));
#37950=CARTESIAN_POINT('',(-16.3598414208564,37.03,7.91980289947518));
#37951=CARTESIAN_POINT('Origin',(-16.0251680583905,37.03,7.37084445728621));
#37952=CARTESIAN_POINT('',(-16.0251680583905,37.03,7.37084445728621));
#37953=CARTESIAN_POINT('Origin',(-15.6651937101241,37.03,6.86159254803069));
#37954=CARTESIAN_POINT('',(-15.6651937101241,37.03,6.86159254803069));
#37955=CARTESIAN_POINT('Origin',(-15.2807225748869,37.03,6.39533953317997));
#37956=CARTESIAN_POINT('',(-15.2807225748869,37.03,6.39533953317997));
#37957=CARTESIAN_POINT('Origin',(-14.8720022673282,37.03,5.97680680020517));
#37958=CARTESIAN_POINT('',(-14.8720022673282,37.03,5.97680680020517));
#37959=CARTESIAN_POINT('Origin',(-14.4379449459854,37.03,5.61417442201851));
#37960=CARTESIAN_POINT('Origin',(-12.617406105901,37.03,3.38082377665168));
#37961=CARTESIAN_POINT('',(-12.617406105901,37.03,3.38082377665168));
#37962=CARTESIAN_POINT('Origin',(-12.8976134221558,37.03,2.0689307051291));
#37963=CARTESIAN_POINT('',(-12.8976134221558,37.03,2.0689307051291));
#37964=CARTESIAN_POINT('Origin',(-14.765314709922,37.03,2.36853222176556));
#37965=CARTESIAN_POINT('',(-14.765314709922,37.03,2.36853222176556));
#37966=CARTESIAN_POINT('Origin',(-15.3107143126737,37.03,2.35695480224783));
#37967=CARTESIAN_POINT('Origin',(-16.997251982187,37.03,1.8902833980495));
#37968=CARTESIAN_POINT('',(-16.997251982187,37.03,1.8902833980495));
#37969=CARTESIAN_POINT('Origin',(-17.5636248671243,37.03,1.62924548184169));
#37970=CARTESIAN_POINT('',(-17.5636248671243,37.03,1.62924548184169));
#37971=CARTESIAN_POINT('Origin',(-18.1279397220842,37.03,1.32117020651705));
#37972=CARTESIAN_POINT('',(-18.1279397220842,37.03,1.32117020651705));
#37973=CARTESIAN_POINT('Origin',(-18.6879695209193,37.03,0.96774550523739));
#37974=CARTESIAN_POINT('',(-18.6879695209193,37.03,0.96774550523739));
#37975=CARTESIAN_POINT('Origin',(-19.2415520497946,37.03,0.570240927191683));
#37976=CARTESIAN_POINT('',(-19.2415520497946,37.03,0.570240927191683));
#37977=CARTESIAN_POINT('Origin',(-19.247887896579,37.03,0.285151750348435));
#37978=CARTESIAN_POINT('',(-19.247887896579,37.03,0.285151750348435));
#37979=CARTESIAN_POINT('Origin',(-19.25,37.03,2.35922392732846E-15));
#37980=CARTESIAN_POINT('',(-19.25,37.03,2.35744508835865E-15));
#37981=CARTESIAN_POINT('Origin',(-19.247887896579,37.03,-0.285151750348431));
#37982=CARTESIAN_POINT('',(-19.247887896579,37.03,-0.285151750348431));
#37983=CARTESIAN_POINT('Origin',(-19.2415520497946,37.03,-0.570240927191679));
#37984=CARTESIAN_POINT('',(-19.2415520497946,37.03,-0.570240927191679));
#37985=CARTESIAN_POINT('Origin',(-18.6879695209193,37.03,-0.967745505237385));
#37986=CARTESIAN_POINT('',(-18.6879695209193,37.03,-0.967745505237385));
#37987=CARTESIAN_POINT('Origin',(-18.1279397220842,37.03,-1.32117020651705));
#37988=CARTESIAN_POINT('',(-18.1279397220842,37.03,-1.32117020651705));
#37989=CARTESIAN_POINT('Origin',(-17.5636248671243,37.03,-1.62924548184168));
#37990=CARTESIAN_POINT('',(-17.5636248671243,37.03,-1.62924548184168));
#37991=CARTESIAN_POINT('Origin',(-16.997251982187,37.03,-1.89028339804949));
#37992=CARTESIAN_POINT('',(-16.997251982187,37.03,-1.89028339804949));
#37993=CARTESIAN_POINT('Origin',(-16.4311637046244,37.03,-2.10183478588267));
#37994=CARTESIAN_POINT('',(-16.4311637046244,37.03,-2.10183478588267));
#37995=CARTESIAN_POINT('Origin',(-15.8679351687486,37.03,-2.25993461117485));
#37996=CARTESIAN_POINT('',(-15.8679351687486,37.03,-2.25993461117485));
#37997=CARTESIAN_POINT('Origin',(-15.3107143126737,37.03,-2.35695480224783));
#37998=CARTESIAN_POINT('Origin',(-12.617406105901,37.03,-3.38082377665168));
#37999=CARTESIAN_POINT('',(-12.617406105901,37.03,-3.38082377665168));
#38000=CARTESIAN_POINT('Origin',(-12.2041262243426,37.03,-4.65706016176646));
#38001=CARTESIAN_POINT('',(-12.2041262243426,37.03,-4.65706016176646));
#38002=CARTESIAN_POINT('Origin',(-13.9714037445473,37.03,-5.33144828123002));
#38003=CARTESIAN_POINT('',(-13.9714037445473,37.03,-5.33144828123002));
#38004=CARTESIAN_POINT('Origin',(-14.4379449459854,37.03,-5.61417442201851));
#38005=CARTESIAN_POINT('Origin',(-15.6651937101241,37.03,-6.86159254803069));
#38006=CARTESIAN_POINT('',(-15.6651937101241,37.03,-6.86159254803069));
#38007=CARTESIAN_POINT('Origin',(-16.0251680583905,37.03,-7.37084445728622));
#38008=CARTESIAN_POINT('',(-16.0251680583905,37.03,-7.37084445728622));
#38009=CARTESIAN_POINT('Origin',(-16.3598414208564,37.03,-7.91980289947518));
#38010=CARTESIAN_POINT('',(-16.3598414208564,37.03,-7.91980289947518));
#38011=CARTESIAN_POINT('Origin',(-16.6681291028841,37.03,-8.50589256852587));
#38012=CARTESIAN_POINT('',(-16.6681291028841,37.03,-8.50589256852587));
#38013=CARTESIAN_POINT('Origin',(-16.9487933469585,37.03,-9.12693289567173));
#38014=CARTESIAN_POINT('',(-16.9487933469585,37.03,-9.12693289567173));
#38015=CARTESIAN_POINT('Origin',(-16.8117357628067,37.03,-9.37699528855417));
#38016=CARTESIAN_POINT('',(-16.8117357628067,37.03,-9.37699528855417));
#38017=CARTESIAN_POINT('Origin',(-16.6709890228504,37.03,-9.625));
#38018=CARTESIAN_POINT('',(-16.6709890228504,37.03,-9.625));
#38019=CARTESIAN_POINT('Origin',(-16.5265840124582,37.03,-9.87089260802485));
#38020=CARTESIAN_POINT('',(-16.5265840124582,37.03,-9.87089260802485));
#38021=CARTESIAN_POINT('Origin',(-16.3785524197668,37.03,-10.1146191541229));
#38022=CARTESIAN_POINT('',(-16.3785524197668,37.03,-10.1146191541229));
#38023=CARTESIAN_POINT('Origin',(-15.7003835976467,37.03,-10.1820769523934));
#38024=CARTESIAN_POINT('',(-15.7003835976467,37.03,-10.1820769523934));
#38025=CARTESIAN_POINT('Origin',(-15.0386712143394,37.03,-10.208136822609));
#38026=CARTESIAN_POINT('',(-15.0386712143394,37.03,-10.208136822609));
#38027=CARTESIAN_POINT('Origin',(-14.3959225765489,37.03,-10.192780409838));
#38028=CARTESIAN_POINT('',(-14.3959225765489,37.03,-10.192780409838));
#38029=CARTESIAN_POINT('Origin',(-13.7749103120746,37.03,-10.1356594341564));
#38030=CARTESIAN_POINT('',(-13.7749103120746,37.03,-10.1356594341564));
#38031=CARTESIAN_POINT('Origin',(-13.1788877890042,37.03,-10.0358241714444));
#38032=CARTESIAN_POINT('',(-13.1788877890042,37.03,-10.0358241714444));
#38033=CARTESIAN_POINT('Origin',(-12.6120676561534,37.03,-9.89112836854343));
#38034=CARTESIAN_POINT('',(-12.6120676561534,37.03,-9.89112836854343));
#38035=CARTESIAN_POINT('Origin',(-12.0809901437375,37.03,-9.69653989065521));
#38036=CARTESIAN_POINT('Origin',(-9.23658232924928,37.03,-9.23658232924928));
#38037=CARTESIAN_POINT('',(-9.23658232924928,37.03,-9.23658232924928));
#38038=CARTESIAN_POINT('Origin',(-8.24055326038937,37.03,-10.1351955192135));
#38039=CARTESIAN_POINT('',(-8.24055326038937,37.03,-10.1351955192135));
#38040=CARTESIAN_POINT('Origin',(-9.43386642869197,37.03,-11.6028715227817));
#38041=CARTESIAN_POINT('',(-9.43386642869197,37.03,-11.6028715227817));
#38042=CARTESIAN_POINT('Origin',(-9.69653989065522,37.03,-12.0809901437375));
#38043=CARTESIAN_POINT('Origin',(-10.1356594341564,37.03,-13.7749103120746));
#38044=CARTESIAN_POINT('',(-10.1356594341564,37.03,-13.7749103120746));
#38045=CARTESIAN_POINT('Origin',(-10.192780409838,37.03,-14.3959225765489));
#38046=CARTESIAN_POINT('',(-10.192780409838,37.03,-14.3959225765489));
#38047=CARTESIAN_POINT('Origin',(-10.208136822609,37.03,-15.0386712143394));
#38048=CARTESIAN_POINT('',(-10.208136822609,37.03,-15.0386712143394));
#38049=CARTESIAN_POINT('Origin',(-10.1820769523934,37.03,-15.7003835976467));
#38050=CARTESIAN_POINT('',(-10.1820769523934,37.03,-15.7003835976467));
#38051=CARTESIAN_POINT('Origin',(-10.1146191541229,37.03,-16.3785524197668));
#38052=CARTESIAN_POINT('',(-10.1146191541229,37.03,-16.3785524197668));
#38053=CARTESIAN_POINT('Origin',(-9.87089260802487,37.03,-16.5265840124582));
#38054=CARTESIAN_POINT('',(-9.87089260802487,37.03,-16.5265840124582));
#38055=CARTESIAN_POINT('Origin',(-9.62500000000001,37.03,-16.6709890228504));
#38056=CARTESIAN_POINT('',(-9.62500000000001,37.03,-16.6709890228504));
#38057=CARTESIAN_POINT('Origin',(-9.37699528855417,37.03,-16.8117357628067));
#38058=CARTESIAN_POINT('',(-9.37699528855417,37.03,-16.8117357628067));
#38059=CARTESIAN_POINT('Origin',(-9.12693289567173,37.03,-16.9487933469585));
#38060=CARTESIAN_POINT('',(-9.12693289567173,37.03,-16.9487933469585));
#38061=CARTESIAN_POINT('Origin',(-8.50589256852587,37.03,-16.6681291028841));
#38062=CARTESIAN_POINT('',(-8.50589256852587,37.03,-16.6681291028841));
#38063=CARTESIAN_POINT('Origin',(-7.91980289947518,37.03,-16.3598414208564));
#38064=CARTESIAN_POINT('',(-7.91980289947518,37.03,-16.3598414208564));
#38065=CARTESIAN_POINT('Origin',(-7.37084445728623,37.03,-16.0251680583905));
#38066=CARTESIAN_POINT('',(-7.37084445728623,37.03,-16.0251680583905));
#38067=CARTESIAN_POINT('Origin',(-6.86159254803069,37.03,-15.6651937101241));
#38068=CARTESIAN_POINT('',(-6.86159254803069,37.03,-15.6651937101241));
#38069=CARTESIAN_POINT('Origin',(-6.39533953317998,37.03,-15.2807225748869));
#38070=CARTESIAN_POINT('',(-6.39533953317998,37.03,-15.2807225748869));
#38071=CARTESIAN_POINT('Origin',(-5.97680680020517,37.03,-14.8720022673282));
#38072=CARTESIAN_POINT('',(-5.97680680020517,37.03,-14.8720022673282));
#38073=CARTESIAN_POINT('Origin',(-5.61417442201851,37.03,-14.4379449459854));
#38074=CARTESIAN_POINT('Origin',(-3.38082377665168,37.03,-12.617406105901));
#38075=CARTESIAN_POINT('Origin',(0.,51.,0.));
#38076=CARTESIAN_POINT('',(-1.04094977927525E-15,18.05,-8.5));
#38077=CARTESIAN_POINT('',(-1.04094977927525E-15,51.,-8.5));
#38078=CARTESIAN_POINT('Origin',(0.,18.05,0.));
#38079=CARTESIAN_POINT('Origin',(0.,-37.8,7.44));
#38080=CARTESIAN_POINT('',(-9.11137218565631E-16,-37.8,-7.44));
#38081=CARTESIAN_POINT('Origin',(0.,-37.8,0.));
#38082=CARTESIAN_POINT('Origin',(0.,-37.55,0.));
#38083=CARTESIAN_POINT('',(-9.72369558522998E-16,-37.3,-7.93999999999999));
#38084=CARTESIAN_POINT('Origin',(0.,-37.3,0.));
#38085=CARTESIAN_POINT('',(-9.41753388544315E-16,-37.55,-7.69));
#38086=CARTESIAN_POINT('Origin',(0.,-9.62499999999999,0.));
#38087=CARTESIAN_POINT('',(-9.72369558522999E-16,18.05,-7.94));
#38088=CARTESIAN_POINT('Origin',(0.,18.05,0.));
#38089=CARTESIAN_POINT('',(-9.72369558522999E-16,-9.62499999999999,-7.94));
#38090=CARTESIAN_POINT('Origin',(0.,18.05,8.5));
#38091=CARTESIAN_POINT('Origin',(0.,51.,0.));
#38092=CARTESIAN_POINT('',(-1.04094977927525E-15,83.95,-8.5));
#38093=CARTESIAN_POINT('Origin',(0.,83.95,0.));
#38094=CARTESIAN_POINT('',(-1.04094977927525E-15,51.,-8.5));
#38095=CARTESIAN_POINT('Origin',(0.,83.95,0.));
#46368=UNCERTAINTY_MEASURE_WITH_UNIT(LENGTH_MEASURE(0.01),#46396,
'DISTANCE_ACCURACY_VALUE',
'Maximum model space distance between geometric entities at asserted c
onnectivities');
#46379=UNCERTAINTY_MEASURE_WITH_UNIT(LENGTH_MEASURE(0.01),#46396,
'DISTANCE_ACCURACY_VALUE',
'Maximum model space distance between geometric entities at asserted c
onnectivities');
#46384=(
GEOMETRIC_REPRESENTATION_CONTEXT(3)
GLOBAL_UNCERTAINTY_ASSIGNED_CONTEXT((#46368))
GLOBAL_UNIT_ASSIGNED_CONTEXT((#46396,#46398,#46399))
REPRESENTATION_CONTEXT('','3D')
);
#46395=(
GEOMETRIC_REPRESENTATION_CONTEXT(3)
GLOBAL_UNCERTAINTY_ASSIGNED_CONTEXT((#46379))
GLOBAL_UNIT_ASSIGNED_CONTEXT((#46396,#46398,#46399))
REPRESENTATION_CONTEXT('','3D')
);
#46396=(
LENGTH_UNIT()
NAMED_UNIT(*)
SI_UNIT(.MILLI.,.METRE.)
);
#46398=(
NAMED_UNIT(*)
PLANE_ANGLE_UNIT()
SI_UNIT($,.RADIAN.)
);
#46399=(
NAMED_UNIT(*)
SI_UNIT($,.STERADIAN.)
SOLID_ANGLE_UNIT()
);
#46404=SHAPE_DEFINITION_REPRESENTATION(#46419,#46459);
#46419=PRODUCT_DEFINITION_SHAPE('',$,#46475);
#46459=SHAPE_REPRESENTATION('',(#25703),#46384);
#46470=PRODUCT_DEFINITION_CONTEXT('part definition',#46517,'design');
#46475=PRODUCT_DEFINITION('2026-10-26-00-50-47-232',
'04_Drive_Gear_Shaft_z12_m2.75',#46490,#46470);
#46490=PRODUCT_DEFINITION_FORMATION('',$,#46523);
#46517=APPLICATION_CONTEXT(
'Core Data for Automotive Mechanical Design Process');
#46518=PRODUCT_CONTEXT('part definition',#46517,'mechanical');
#46523=PRODUCT('2026-10-26-00-50-47-232',
'04_Drive_Gear_Shaft_z12_m2.75',$,(#46518));
#46590=COLOUR_RGB('Grey',0.48,0.52,0.57);
#46591=FILL_AREA_STYLE_COLOUR('',#46590);
#46592=FILL_AREA_STYLE('',(#46591));
#46593=SURFACE_STYLE_FILL_AREA(#46592);
#46594=SURFACE_SIDE_STYLE('',(#46593));
#46595=SURFACE_STYLE_USAGE(.BOTH.,#46594);
#46596=PRESENTATION_STYLE_ASSIGNMENT((#46595));
ENDSEC;
END-ISO-10303-21;
